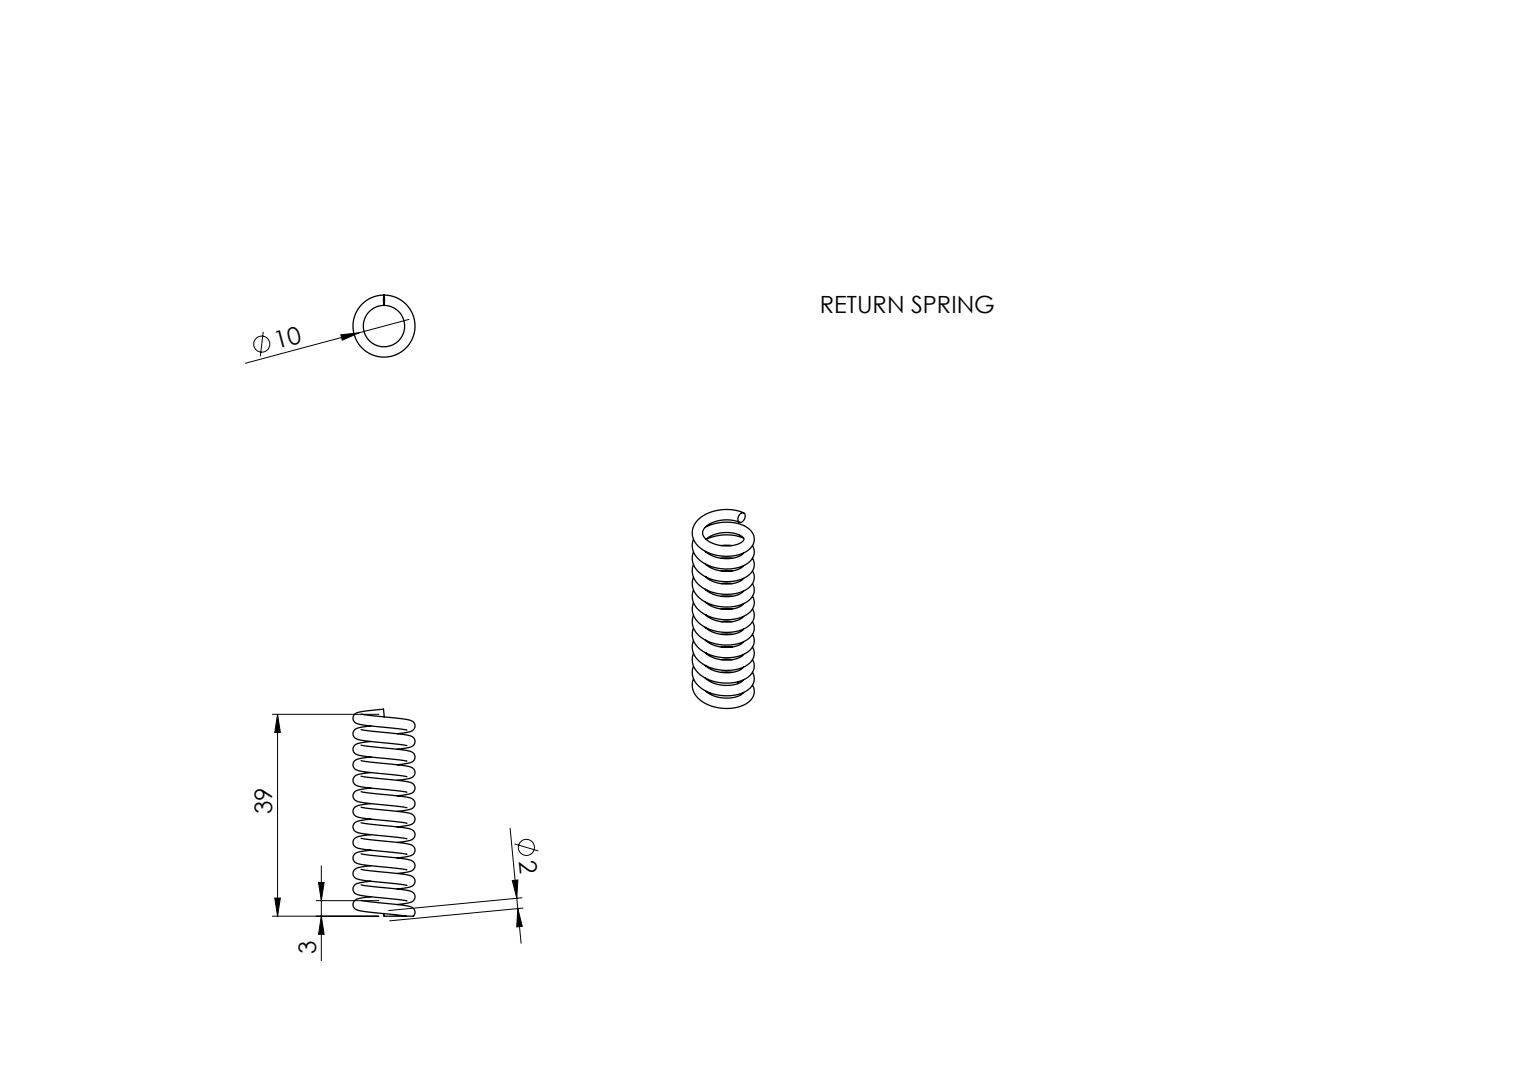
ISO-10303-21;
HEADER;
FILE_DESCRIPTION (('STEP AP214'),
    '1' );
FILE_NAME ('return spring.step',
    '2026-10-04T07:56:41',
    ( '' ),
    ( '' ),
    'SwSTEP 2.0',
    'SolidWorks 2026',
    '' );
FILE_SCHEMA (( 'AUTOMOTIVE_DESIGN' ));
ENDSEC;

DATA;
#1=CARTESIAN_POINT ( 'NONE',  ( 2.179377348189627916, -63.64547149457072805, 7.030887037049939003 ) ) ;
#3=CARTESIAN_POINT ( 'NONE',  ( 1.529537955723794918, -69.64547149457074227, 5.030887037049945221 ) ) ;
#4=CARTESIAN_POINT ( 'NONE',  ( -0.09506052544073731458, -60.49547149457074369, 4.999999999999997335 ) ) ;
#7=CARTESIAN_POINT ( 'NONE',  ( -3.015831842038216859, -60.30452850542926058, -3.989209796945429432 ) ) ;
#8=CARTESIAN_POINT ( 'NONE',  ( -7.360235569667856304, -89.74547149457073658, -0.09995255151716124498 ) ) ;
#10=CARTESIAN_POINT ( 'NONE',  ( -1.719659006605372076, -75.15452850542925489, -4.969112962950016588 ) ) ;
#15=CARTESIAN_POINT ( 'NONE',  ( -4.312004677470992142, -84.04547149457074795, 3.009306630940933758 ) ) ;
#16=CARTESIAN_POINT ( 'NONE',  ( 4.332187097882923332, -97.00000000000000000, -0.04074656551593417581 ) ) ;
#17=CARTESIAN_POINT ( 'NONE',  ( -2.610703060766926598, -69.04547149457074795, 1.773238653441125745 ) ) ;
#18=CARTESIAN_POINT ( 'NONE',  ( 6.628020296210641149, -74.40452850542925489, -2.253526892787612645 ) ) ;
#20=CARTESIAN_POINT ( 'NONE',  ( 4.725907263620373833, -82.09547149457074511, 1.635492904037598283 ) ) ;
#21=CARTESIAN_POINT ( 'NONE',  ( -5.257311121191324155, -60.75452850542925631, 0.09995255151729526277 ) ) ;
#22=CARTESIAN_POINT ( 'NONE',  ( -2.862020680886492308, -91.20452850542926626, 4.100960146804039752 ) ) ;
#23=CARTESIAN_POINT ( 'NONE',  ( -0.09506052544086251999, -66.00452850542926342, -6.999999999999997335 ) ) ;
#24=CARTESIAN_POINT ( 'NONE',  ( -2.823794231030039015, -86.59547149457075932, -1.017458915287723364 ) ) ;
#27=DIRECTION ( 'NONE',  ( -0.9954714945707483498, -0.09506052544079827971, 1.047588144072330487E-14 ) ) ;
#29=CARTESIAN_POINT ( 'NONE',  ( 4.194503406049339134, -89.55452850542926058, -3.171033256558100089 ) ) ;
#31=CARTESIAN_POINT ( 'NONE',  ( 1.529537955723690779, -80.85452850542925773, -5.030887037049978971 ) ) ;
#32=CARTESIAN_POINT ( 'NONE',  ( 2.493201789345269148, -59.55452850542924637, -1.934965279058294518 ) ) ;
#34=CARTESIAN_POINT ( 'NONE',  ( -1.719659006605370744, -90.15452850542922647, -4.969112962950016588 ) ) ;
#35=CARTESIAN_POINT ( 'NONE',  ( 4.037591185471445243, -92.70452850542926626, -5.718994135553947977 ) ) ;
#36=CARTESIAN_POINT ( 'NONE',  ( -3.015831842038128485, -81.19547149457073942, 3.989209796945492048 ) ) ;
#37=CARTESIAN_POINT ( 'NONE',  ( 2.823794231030039903, -71.40452850542924068, -1.017458915287783316 ) ) ;
#40=CARTESIAN_POINT ( 'NONE',  ( 2.823794231030042123, -89.40452850542926910, -1.017458915287783316 ) ) ;
#41=CARTESIAN_POINT ( 'NONE',  ( 2.179377348189484476, -95.85452850542924352, -7.030887037049986077 ) ) ;
#45=CARTESIAN_POINT ( 'NONE',  ( 1.719659006605391394, -79.65452850542925489, 4.969112962950016588 ) ) ;
#46=CARTESIAN_POINT ( 'NONE',  ( 2.369498399071079842, -94.84547149457073090, -6.969112962950057444 ) ) ;
#53=CARTESIAN_POINT ( 'NONE',  ( -1.529537955723671905, -61.35452850542925773, 5.030887037049979860 ) ) ;
#54=CARTESIAN_POINT ( 'NONE',  ( -4.191402346623057440, -87.19547149457073942, 5.607243785695398941 ) ) ;
#57=CARTESIAN_POINT ( 'NONE',  ( 5.257311121191341918, -71.25452850542923500, -0.09995255151729465215 ) ) ;
#61=CARTESIAN_POINT ( 'NONE',  ( 1.719659006605285922, -76.84547149457073090, -4.969112962950050338 ) ) ;
#62=CARTESIAN_POINT ( 'NONE',  ( 4.269446988268172483, -97.00000000000001421, -0.4101805542161022777 ) ) ;
#63=CARTESIAN_POINT ( 'NONE',  ( 0.8796985632579598091, -60.64547149457074227, 3.030887037049952326 ) ) ;
#64=CARTESIAN_POINT ( 'NONE',  ( 5.895805022753404678, -68.55452850542926058, -4.407101234057908989 ) ) ;
#66=CARTESIAN_POINT ( 'NONE',  ( -4.194503406049384431, -77.44547149457075363, -3.171033256558012159 ) ) ;
#67=CARTESIAN_POINT ( 'NONE',  ( 5.257311121191341918, -59.25452850542924210, -0.09995255151729465215 ) ) ;
#68=CARTESIAN_POINT ( 'NONE',  ( -4.725907263620319654, -87.90452850542926910, 1.635492904037698647 ) ) ;
#69=CARTESIAN_POINT ( 'NONE',  ( -4.191402346623179120, -72.30452850542926058, -5.607243785695311900 ) ) ;
#71=CARTESIAN_POINT ( 'NONE',  ( -2.823794231030039903, -77.59547149457073090, -1.017458915287723364 ) ) ;
#75=CARTESIAN_POINT ( 'NONE',  ( 2.862020680886515400, -86.70452850542925205, -4.100960146804039752 ) ) ;
#77=CARTESIAN_POINT ( 'NONE',  ( -1.529537955723670128, -79.35452850542925773, 5.030887037049979860 ) ) ;
#78=CARTESIAN_POINT ( 'NONE',  ( -2.610703060766966566, -63.45452850542924494, -1.773238653441072232 ) ) ;
#80=CARTESIAN_POINT ( 'NONE',  ( -2.862020680886493640, -82.20452850542925205, 4.100960146804039752 ) ) ;
#81=CARTESIAN_POINT ( 'NONE',  ( 2.369498399071075845, -64.84547149457071669, -6.969112962950057444 ) ) ;
#82=CARTESIAN_POINT ( 'NONE',  ( 1.069819614139556396, -70.65452850542925489, 2.969112962950023249 ) ) ;
#83=EDGE_CURVE ( 'NONE', #4707, #1590, #2672, .T. ) ;
#86=CARTESIAN_POINT ( 'NONE',  ( 3.154386672714810658, -89.25452850542926342, -0.09995255151727241993 ) ) ;
#87=CARTESIAN_POINT ( 'NONE',  ( 4.191402346623199549, -94.80452850542926058, 5.607243785695311900 ) ) ;
#89=CARTESIAN_POINT ( 'NONE',  ( 1.529537955723689890, -74.85452850542925773, -5.030887037049978971 ) ) ;
#90=CARTESIAN_POINT ( 'NONE',  ( -5.895805022753476621, -89.44547149457073942, -4.407101234057782868 ) ) ;
#93=CARTESIAN_POINT ( 'NONE',  ( -0.09506052544075821453, -63.49547149457075079, 2.999999999999997780 ) ) ;
#95=CARTESIAN_POINT ( 'NONE',  ( -4.312004677471060532, -60.45452850542923784, -3.009306630940844052 ) ) ;
#96=CARTESIAN_POINT ( 'NONE',  ( -6.013306294175058575, -87.04547149457074795, 4.245374608440741326 ) ) ;
#99=CARTESIAN_POINT ( 'NONE',  ( -3.015831842038215083, -75.30452850542926058, -3.989209796945429432 ) ) ;
#103=CARTESIAN_POINT ( 'NONE',  ( 2.862020680886599333, -78.79547149457074795, 4.100960146803977580 ) ) ;
#105=CARTESIAN_POINT ( 'NONE',  ( -1.840261337453202639, -60.19547149457074653, 2.371175808195584267 ) ) ;
#106=CARTESIAN_POINT ( 'NONE',  ( 6.686770931921523164, -65.10452850542924352, 2.072711028461649008 ) ) ;
#108=CARTESIAN_POINT ( 'NONE',  ( 1.529537955723795584, -81.64547149457074227, 5.030887037049945221 ) ) ;
#110=CARTESIAN_POINT ( 'NONE',  ( 3.015831842038235511, -88.80452850542926058, 3.989209796945429432 ) ) ;
#111=CARTESIAN_POINT ( 'NONE',  ( -6.013306294175152722, -72.45452850542925205, -4.245374608440613429 ) ) ;
#112=CARTESIAN_POINT ( 'NONE',  ( 3.154386672714809770, -79.24547149457073658, 0.09995255151720662534 ) ) ;
#118=CARTESIAN_POINT ( 'NONE',  ( -2.862020680886492308, -91.20452850542926626, 4.100960146804039752 ) ) ;
#120=CARTESIAN_POINT ( 'NONE',  ( 4.725907263620340970, -80.40452850542925489, -1.635492904037697981 ) ) ;
#121=CARTESIAN_POINT ( 'NONE',  ( 2.610703060766946582, -88.54547149457074795, -1.773238653441125523 ) ) ;
#123=CARTESIAN_POINT ( 'NONE',  ( -0.09506052544083921918, -84.00452850542926342, -4.999999999999997335 ) ) ;
#125=CARTESIAN_POINT ( 'NONE',  ( 0.09506052544073236021, -61.99547149457073658, -6.999999999999997335 ) ) ;
#127=CARTESIAN_POINT ( 'NONE',  ( -1.840261337453252821, -69.30452850542926058, -2.371175808195547852 ) ) ;
#131=CARTESIAN_POINT ( 'NONE',  ( 1.069819614139557284, -79.65452850542925489, 2.969112962950023249 ) ) ;
#132=CARTESIAN_POINT ( 'NONE',  ( 7.360235569667880284, -92.25452850542926342, -0.09995255151731691212 ) ) ;
#134=CARTESIAN_POINT ( 'NONE',  ( -6.628020296210666018, -86.59547149457075932, -2.253526892787471869 ) ) ;
#138=CARTESIAN_POINT ( 'NONE',  ( -0.8796985632579439329, -68.14547149457074227, -3.030887037049952326 ) ) ;
#139=CARTESIAN_POINT ( 'NONE',  ( -4.194503406049321370, -58.05452850542925347, 3.171033256558100533 ) ) ;
#141=CARTESIAN_POINT ( 'NONE',  ( 4.312004677471075631, -73.95452850542926626, 3.009306630940844496 ) ) ;
#142=CARTESIAN_POINT ( 'NONE',  ( -0.09506052544071266763, -87.49547149457075079, 6.999999999999997335 ) ) ;
#144=CARTESIAN_POINT ( 'NONE',  ( 0.09506052544086046607, -79.50452850542926342, 4.999999999999997335 ) ) ;
#147=CARTESIAN_POINT ( 'NONE',  ( -4.312004677470993030, -78.04547149457076216, 3.009306630940933758 ) ) ;
#149=CARTESIAN_POINT ( 'NONE',  ( -2.610703060766927930, -63.04547149457074084, 1.773238653441125745 ) ) ;
#150=CARTESIAN_POINT ( 'NONE',  ( -5.895805022753386915, -67.05452850542926058, 4.407101234057909878 ) ) ;
#152=CARTESIAN_POINT ( 'NONE',  ( -5.257311121191324155, -74.74547149457075079, -0.09995255151718371311 ) ) ;
#155=CARTESIAN_POINT ( 'NONE',  ( 0.09506052544086084077, -82.50452850542926342, 4.999999999999997335 ) ) ;
#156=CARTESIAN_POINT ( 'NONE',  ( 6.686770931921523164, -68.10452850542924352, 2.072711028461649008 ) ) ;
#157=CARTESIAN_POINT ( 'NONE',  ( 0.8796985632579618075, -75.64547149457072805, 3.030887037049952326 ) ) ;
#161=CARTESIAN_POINT ( 'NONE',  ( 2.862020680886516732, -95.70452850542926626, -4.100960146804039752 ) ) ;
#162=CARTESIAN_POINT ( 'NONE',  ( 3.015831842038235511, -88.80452850542926058, 3.989209796945429432 ) ) ;
#164=CARTESIAN_POINT ( 'NONE',  ( -2.862020680886494084, -79.20452850542925205, 4.100960146804039752 ) ) ;
#165=CARTESIAN_POINT ( 'NONE',  ( -3.154386672714787565, -89.74547149457073658, -0.09995255151720625064 ) ) ;
#166=CARTESIAN_POINT ( 'NONE',  ( 1.719659006605392504, -88.65452850542925489, 4.969112962950016588 ) ) ;
#168=CARTESIAN_POINT ( 'NONE',  ( -6.013306294175062128, -60.04547149457073374, 4.245374608440741326 ) ) ;
#169=CARTESIAN_POINT ( 'NONE',  ( -1.686450176301567350, -64.20452850542925205, 2.482926158054133303 ) ) ;
#172=CARTESIAN_POINT ( 'NONE',  ( 0.8796985632578988579, -74.85452850542925773, -3.030887037049972310 ) ) ;
#173=CARTESIAN_POINT ( 'NONE',  ( -2.179377348189460051, -88.35452850542924352, 7.030887037049988741 ) ) ;
#175=CARTESIAN_POINT ( 'NONE',  ( -4.037591185471542943, -89.29547149457074795, -5.718994135553860936 ) ) ;
#178=CARTESIAN_POINT ( 'NONE',  ( -1.069819614139475794, -66.34547149457073090, 2.969112962950044121 ) ) ;
#179=CARTESIAN_POINT ( 'NONE',  ( -4.725907263620323207, -63.90452850542925489, 1.635492904037698647 ) ) ;
#182=CARTESIAN_POINT ( 'NONE',  ( 5.257311121191341918, -71.25452850542923500, -0.09995255151729465215 ) ) ;
#183=CARTESIAN_POINT ( 'NONE',  ( 0.09506052544073499699, -82.99547149457075079, -6.999999999999997335 ) ) ;
#185=CARTESIAN_POINT ( 'NONE',  ( 1.529537955723690112, -77.85452850542922931, -5.030887037049978971 ) ) ;
#191=CARTESIAN_POINT ( 'NONE',  ( 3.015831842038148025, -70.69547149457073942, -3.989209796945492048 ) ) ;
#193=CARTESIAN_POINT ( 'NONE',  ( -1.686450176301618642, -65.29547149457073374, -2.482926158054096000 ) ) ;
#194=CARTESIAN_POINT ( 'NONE',  ( 7.360235569667877620, -74.25452850542924921, -0.09995255151731691212 ) ) ;
#197=CARTESIAN_POINT ( 'NONE',  ( 1.529537955723691001, -83.85452850542927195, -5.030887037049978971 ) ) ;
#198=CARTESIAN_POINT ( 'NONE',  ( -6.628020296210623385, -63.90452850542925489, 2.253526892787613978 ) ) ;
#199=CARTESIAN_POINT ( 'NONE',  ( -1.069819614139474906, -75.34547149457073090, 2.969112962950044121 ) ) ;
#202=CARTESIAN_POINT ( 'NONE',  ( -1.719659006605370744, -93.15452850542925489, -4.969112962950016588 ) ) ;
#203=CARTESIAN_POINT ( 'NONE',  ( 4.725907263620340970, -83.40452850542925489, -1.635492904037697981 ) ) ;
#205=CARTESIAN_POINT ( 'NONE',  ( 5.257311121191341030, -71.25452850542924921, -0.09995255151729466603 ) ) ;
#206=CARTESIAN_POINT ( 'NONE',  ( 2.610703060766947914, -94.54547149457073374, -1.773238653441125523 ) ) ;
#207=CARTESIAN_POINT ( 'NONE',  ( -4.194503406049315153, -91.05452850542923215, 3.171033256558100533 ) ) ;
#208=CARTESIAN_POINT ( 'NONE',  ( 6.013306294175077227, -61.54547149457074084, -4.245374608440741326 ) ) ;
#209=CARTESIAN_POINT ( 'NONE',  ( -1.840261337453252821, -66.30452850542926058, -2.371175808195547852 ) ) ;
#213=CARTESIAN_POINT ( 'NONE',  ( -1.686450176301564907, -82.20452850542925205, 2.482926158054133303 ) ) ;
#214=CARTESIAN_POINT ( 'NONE',  ( 2.179377348189483143, -86.85452850542924352, -7.030887037049986077 ) ) ;
#215=CARTESIAN_POINT ( 'NONE',  ( -4.191402346623057440, -87.19547149457073942, 5.607243785695398941 ) ) ;
#218=CARTESIAN_POINT ( 'NONE',  ( -0.09506052544075743738, -69.49547149457075079, 2.999999999999997780 ) ) ;
#223=CARTESIAN_POINT ( 'NONE',  ( -4.194503406049319594, -67.05452850542926058, 3.171033256558100533 ) ) ;
#224=CARTESIAN_POINT ( 'NONE',  ( 6.628020296210687334, -79.09547149457075932, 2.253526892787472757 ) ) ;
#228=CARTESIAN_POINT ( 'NONE',  ( -5.257311121191324155, -63.75452850542925631, 0.09995255151729526277 ) ) ;
#230=CARTESIAN_POINT ( 'NONE',  ( -5.257311121191324155, -71.74547149457075079, -0.09995255151718371311 ) ) ;
#232=CARTESIAN_POINT ( 'NONE',  ( 1.719659006605287921, -97.84547149457071669, -4.969112962950050338 ) ) ;
#233=CARTESIAN_POINT ( 'NONE',  ( 6.686770931921522276, -62.10452850542925063, 2.072711028461649008 ) ) ;
#235=CARTESIAN_POINT ( 'NONE',  ( 1.719659006605391616, -82.65452850542925489, 4.969112962950016588 ) ) ;
#236=CARTESIAN_POINT ( 'NONE',  ( 6.628020296210639373, -62.40452850542925489, -2.253526892787612645 ) ) ;
#237=CARTESIAN_POINT ( 'NONE',  ( 2.882544866740877065, -73.39547149457074227, -0.8366430509619593447 ) ) ;
#240=CARTESIAN_POINT ( 'NONE',  ( 3.015831842038236399, -94.80452850542924637, 3.989209796945429432 ) ) ;
#241=CARTESIAN_POINT ( 'NONE',  ( 1.529537955723690112, -77.85452850542922931, -5.030887037049978971 ) ) ;
#243=CARTESIAN_POINT ( 'NONE',  ( -4.312004677471057867, -72.45452850542923784, -3.009306630940843608 ) ) ;
#244=CARTESIAN_POINT ( 'NONE',  ( -0.8796985632579418235, -86.14547149457072805, -3.030887037049952326 ) ) ;
#245=CARTESIAN_POINT ( 'NONE',  ( 2.862020680886601998, -96.79547149457073374, 4.100960146803977580 ) ) ;
#246=CARTESIAN_POINT ( 'NONE',  ( 0.09506052544086046607, -79.50452850542926342, 4.999999999999997335 ) ) ;
#247=CARTESIAN_POINT ( 'NONE',  ( 2.369498399071225947, -85.65452850542926910, 6.969112962950009482 ) ) ;
#249=CARTESIAN_POINT ( 'NONE',  ( 1.686450176301584225, -68.70452850542925205, -2.482926158054133303 ) ) ;
#252=LINE ( 'NONE', #8058, #5108 ) ;
#253=CARTESIAN_POINT ( 'NONE',  ( 1.686450176301585335, -77.70452850542925205, -2.482926158054133303 ) ) ;
#254=CARTESIAN_POINT ( 'NONE',  ( 7.360235569667880284, -86.25452850542924921, -0.09995255151731691212 ) ) ;
#256=CARTESIAN_POINT ( 'NONE',  ( 4.191402346623080533, -88.69547149457073942, -5.607243785695398941 ) ) ;
#260=CARTESIAN_POINT ( 'NONE',  ( 0.09506052544077478461, -64.99547149457075079, -2.999999999999997780 ) ) ;
#263=CARTESIAN_POINT ( 'NONE',  ( 3.015831842038232402, -64.80452850542926058, 3.989209796945429432 ) ) ;
#264=CARTESIAN_POINT ( 'NONE',  ( 2.369498399071077177, -76.84547149457073090, -6.969112962950057444 ) ) ;
#265=FILL_AREA_STYLE ('',( #2132 ) ) ;
#268=CARTESIAN_POINT ( 'NONE',  ( -1.719659006605265716, -75.34547149457074511, 4.969112962950051227 ) ) ;
#269=CARTESIAN_POINT ( 'NONE',  ( -0.09506052544084110656, -69.00452850542926342, -4.999999999999997335 ) ) ;
#272=CARTESIAN_POINT ( 'NONE',  ( -4.784657899331159925, -65.89547149457074227, 1.454677039711874675 ) ) ;
#274=CARTESIAN_POINT ( 'NONE',  ( -4.784657899331155484, -95.89547149457074227, 1.454677039711874675 ) ) ;
#275=CARTESIAN_POINT ( 'NONE',  ( -6.013306294175153610, -60.45452850542925916, -4.245374608440613429 ) ) ;
#279=CARTESIAN_POINT ( 'NONE',  ( 1.529537955723690557, -80.85452850542925773, -5.030887037049978971 ) ) ;
#283=CARTESIAN_POINT ( 'NONE',  ( -4.312004677471056091, -87.45452850542925205, -3.009306630940844052 ) ) ;
#284=CARTESIAN_POINT ( 'NONE',  ( -1.529537955723669684, -82.35452850542922931, 5.030887037049979860 ) ) ;
#286=CARTESIAN_POINT ( 'NONE',  ( -0.09506052544084110656, -69.00452850542926342, -4.999999999999997335 ) ) ;
#287=CARTESIAN_POINT ( 'NONE',  ( 2.493201789345311337, -87.94547149457073942, 1.934965279058241006 ) ) ;
#288=CARTESIAN_POINT ( 'NONE',  ( -2.493201789345293129, -59.44547149457074653, -1.934965279058240561 ) ) ;
#289=CARTESIAN_POINT ( 'NONE',  ( 1.719659006605391172, -76.65452850542922647, 4.969112962950016588 ) ) ;
#290=CARTESIAN_POINT ( 'NONE',  ( 6.628020296210642037, -86.40452850542926910, -2.253526892787612645 ) ) ;
#292=CARTESIAN_POINT ( 'NONE',  ( -2.493201789345288688, -95.44547149457075363, -1.934965279058240561 ) ) ;
#296=CARTESIAN_POINT ( 'NONE',  ( 1.840261337453271473, -82.80452850542926058, 2.371175808195547852 ) ) ;
#297=CARTESIAN_POINT ( 'NONE',  ( -7.360235569667856304, -87.75452850542924921, 0.09995255151731782806 ) ) ;
#298=CARTESIAN_POINT ( 'NONE',  ( 2.369498399071078065, -79.84547149457074511, -6.969112962950057444 ) ) ;
#300=CARTESIAN_POINT ( 'NONE',  ( 2.862020680886601554, -93.79547149457074795, 4.100960146803977580 ) ) ;
#301=CARTESIAN_POINT ( 'NONE',  ( -0.8796985632578785408, -82.35452850542927195, 3.030887037049973198 ) ) ;
#306=CARTESIAN_POINT ( 'NONE',  ( -5.257311121191324155, -63.75452850542925631, 0.09995255151729526277 ) ) ;
#307=CARTESIAN_POINT ( 'NONE',  ( -2.369498399071056305, -84.34547149457075932, 6.969112962950058332 ) ) ;
#309=CARTESIAN_POINT ( 'NONE',  ( 1.529537955723795584, -75.64547149457072805, 5.030887037049945221 ) ) ;
#310=CARTESIAN_POINT ( 'NONE',  ( 4.784657899331176800, -73.39547149457074227, -1.454677039711874009 ) ) ;
#311=CARTESIAN_POINT ( 'NONE',  ( -4.194503406049319594, -67.05452850542926058, 3.171033256558100533 ) ) ;
#313=CARTESIAN_POINT ( 'NONE',  ( 1.529537955723795140, -69.64547149457074227, 5.030887037049945221 ) ) ;
#315=CARTESIAN_POINT ( 'NONE',  ( -6.686770931921508954, -57.60452850542926484, -2.072711028461647675 ) ) ;
#322=CARTESIAN_POINT ( 'NONE',  ( -4.194503406049315153, -88.05452850542921794, 3.171033256558100533 ) ) ;
#323=CARTESIAN_POINT ( 'NONE',  ( -4.312004677471057867, -78.45452850542925205, -3.009306630940844052 ) ) ;
#325=CARTESIAN_POINT ( 'NONE',  ( 1.719659006605389839, -67.65452850542925489, 4.969112962950015699 ) ) ;
#326=CARTESIAN_POINT ( 'NONE',  ( 0.09506052544077665811, -79.99547149457075079, -2.999999999999997780 ) ) ;
#327=CARTESIAN_POINT ( 'NONE',  ( -4.312004677470990366, -96.04547149457074795, 3.009306630940933758 ) ) ;
#329=CARTESIAN_POINT ( 'NONE',  ( -4.194503406049316929, -73.05452850542926058, 3.171033256558100533 ) ) ;
#330=CARTESIAN_POINT ( 'NONE',  ( -6.013306294175149169, -87.45452850542925205, -4.245374608440613429 ) ) ;
#331=CARTESIAN_POINT ( 'NONE',  ( 2.823794231030038571, -59.40452850542925489, -1.017458915287783316 ) ) ;
#336=CARTESIAN_POINT ( 'NONE',  ( 2.823794231030039903, -71.40452850542924068, -1.017458915287783316 ) ) ;
#337=CARTESIAN_POINT ( 'NONE',  ( -6.013306294175152722, -78.45452850542925205, -4.245374608440613429 ) ) ;
#338=CARTESIAN_POINT ( 'NONE',  ( -6.628020296210667794, -80.59547149457075932, -2.253526892787471869 ) ) ;
#340=CARTESIAN_POINT ( 'NONE',  ( -4.784657899331155484, -95.89547149457074227, 1.454677039711874675 ) ) ;
#341=CARTESIAN_POINT ( 'NONE',  ( 0.8796985632579006342, -89.85452850542924352, -3.030887037049972310 ) ) ;
#345=CARTESIAN_POINT ( 'NONE',  ( -2.882544866740875289, -93.60452850542925773, -0.8366430509618996147 ) ) ;
#346=CARTESIAN_POINT ( 'NONE',  ( 5.895805022753496161, -84.94547149457073942, 4.407101234057782868 ) ) ;
#349=CARTESIAN_POINT ( 'NONE',  ( 4.194503406049401306, -72.94547149457073942, 3.171033256558012159 ) ) ;
#350=CARTESIAN_POINT ( 'NONE',  ( -5.257311121191324155, -71.74547149457075079, -0.09995255151718371311 ) ) ;
#351=CARTESIAN_POINT ( 'NONE',  ( -4.312004677471058756, -69.45452850542925205, -3.009306630940844052 ) ) ;
#354=CARTESIAN_POINT ( 'NONE',  ( -4.725907263620354293, -68.59547149457073090, -1.635492904037597617 ) ) ;
#355=CARTESIAN_POINT ( 'NONE',  ( 2.369498399071222838, -58.65452850542925489, 6.969112962950009482 ) ) ;
#362=CARTESIAN_POINT ( 'NONE',  ( 5.257311121191341918, -83.25452850542926342, -0.09995255151729465215 ) ) ;
#363=CARTESIAN_POINT ( 'NONE',  ( 4.725907263620340082, -74.40452850542925489, -1.635492904037697981 ) ) ;
#364=CARTESIAN_POINT ( 'NONE',  ( -4.194503406049317817, -76.05452850542926058, 3.171033256558101865 ) ) ;
#365=CARTESIAN_POINT ( 'NONE',  ( 2.610703060766946138, -79.54547149457074795, -1.773238653441125523 ) ) ;
#366=CARTESIAN_POINT ( 'NONE',  ( 5.257311121191343695, -97.24547149457075079, 0.09995255151718437925 ) ) ;
#367=CARTESIAN_POINT ( 'NONE',  ( -4.312004677471058756, -69.45452850542925205, -3.009306630940844052 ) ) ;
#368=CARTESIAN_POINT ( 'NONE',  ( -4.191402346623178232, -84.30452850542926058, -5.607243785695311900 ) ) ;
#370=CARTESIAN_POINT ( 'NONE',  ( 0.09506052544083654077, -58.50452850542925631, 2.999999999999997780 ) ) ;
#377=CARTESIAN_POINT ( 'NONE',  ( -0.09506052544081970701, -72.00452850542926342, -2.999999999999997780 ) ) ;
#378=CARTESIAN_POINT ( 'NONE',  ( 6.013306294175077227, -79.54547149457074795, -4.245374608440741326 ) ) ;
#381=CARTESIAN_POINT ( 'NONE',  ( -2.610703060766964345, -81.45452850542925205, -1.773238653441072232 ) ) ;
#385=CARTESIAN_POINT ( 'NONE',  ( 0.09506052544084107880, -94.50452850542926342, 2.999999999999997780 ) ) ;
#387=CARTESIAN_POINT ( 'NONE',  ( -7.360235569667858968, -68.74547149457075079, -0.09995255151716124498 ) ) ;
#390=CARTESIAN_POINT ( 'NONE',  ( 4.194503406049403083, -75.94547149457073942, 3.171033256558012159 ) ) ;
#391=CARTESIAN_POINT ( 'NONE',  ( -0.09506052544073655131, -66.49547149457075079, 4.999999999999997335 ) ) ;
#392=CARTESIAN_POINT ( 'NONE',  ( 4.194503406049335581, -65.55452850542923215, -3.171033256558100089 ) ) ;
#398=CARTESIAN_POINT ( 'NONE',  ( 3.015831842038147137, -64.69547149457075363, -3.989209796945492048 ) ) ;
#400=CARTESIAN_POINT ( 'NONE',  ( 4.312004677471079184, -94.95452850542926626, 3.009306630940844496 ) ) ;
#405=CARTESIAN_POINT ( 'NONE',  ( -2.862020680886492752, -88.20452850542925205, 4.100960146804039752 ) ) ;
#406=CARTESIAN_POINT ( 'NONE',  ( -4.784657899331190123, -78.60452850542925773, -1.454677039711773867 ) ) ;
#408=CARTESIAN_POINT ( 'NONE',  ( -4.725907263620323207, -63.90452850542925489, 1.635492904037698647 ) ) ;
#409=CARTESIAN_POINT ( 'NONE',  ( -2.823794231030039459, -83.59547149457075932, -1.017458915287723364 ) ) ;
#410=CARTESIAN_POINT ( 'NONE',  ( -0.09506052544075858923, -60.49547149457073658, 2.999999999999997780 ) ) ;
#411=CARTESIAN_POINT ( 'NONE',  ( 5.257311121191341918, -68.25452850542926342, -0.09995255151729465215 ) ) ;
#412=CARTESIAN_POINT ( 'NONE',  ( 4.037591185471443467, -83.70452850542925205, -5.718994135553947977 ) ) ;
#413=CARTESIAN_POINT ( 'NONE',  ( 2.610703060766947914, -97.54547149457074795, -1.773238653441125523 ) ) ;
#418=CARTESIAN_POINT ( 'NONE',  ( -1.529537955723668574, -91.35452850542924352, 5.030887037049979860 ) ) ;
#419=CARTESIAN_POINT ( 'NONE',  ( -0.09506052544082045641, -66.00452850542926342, -2.999999999999997780 ) ) ;
#420=CARTESIAN_POINT ( 'NONE',  ( -5.895805022753477509, -80.44547149457073942, -4.407101234057782868 ) ) ;
#422=CARTESIAN_POINT ( 'NONE',  ( 0.09506052544075753452, -94.99547149457073658, -4.999999999999997335 ) ) ;
#423=CARTESIAN_POINT ( 'NONE',  ( -2.882544866740876177, -84.60452850542927195, -0.8366430509618996147 ) ) ;
#427=CARTESIAN_POINT ( 'NONE',  ( -5.257311121191324155, -60.75452850542925631, 0.09995255151729526277 ) ) ;
#428=CARTESIAN_POINT ( 'NONE',  ( -2.179377348189611929, -71.14547149457074227, -7.030887037049939003 ) ) ;
#430=CARTESIAN_POINT ( 'NONE',  ( 4.460500007776900588, -96.99999999999960210, 2.535776773627464564 ) ) ;
#431=CARTESIAN_POINT ( 'NONE',  ( 3.015831842038148025, -70.69547149457073942, -3.989209796945492048 ) ) ;
#432=CARTESIAN_POINT ( 'NONE',  ( -4.312004677470993919, -72.04547149457074795, 3.009306630940933758 ) ) ;
#433=CARTESIAN_POINT ( 'NONE',  ( -1.719659006605374962, -57.15452850542924068, -4.969112962950016588 ) ) ;
#436=CARTESIAN_POINT ( 'NONE',  ( 0.09506052544085857869, -64.50452850542926342, 4.999999999999997335 ) ) ;
#437=CARTESIAN_POINT ( 'NONE',  ( 4.312004677471010794, -64.54547149457073374, -3.009306630940933314 ) ) ;
#439=CARTESIAN_POINT ( 'NONE',  ( -4.194503406049314265, -94.05452850542926058, 3.171033256558100533 ) ) ;
#441=DIRECTION ( 'NONE',  ( -0.09506052544079829358, 0.9954714945707483498, 0.000000000000000000 ) ) ;
#444=CARTESIAN_POINT ( 'NONE',  ( -1.529537955723669684, -82.35452850542922931, 5.030887037049979860 ) ) ;
#445=CARTESIAN_POINT ( 'NONE',  ( 4.725907263620374721, -94.09547149457074511, 1.635492904037598283 ) ) ;
#446=CARTESIAN_POINT ( 'NONE',  ( 3.015831842038231958, -61.80452850542926058, 3.989209796945429432 ) ) ;
#447=CARTESIAN_POINT ( 'NONE',  ( -1.686450176301616199, -83.29547149457074795, -2.482926158054096000 ) ) ;
#448=CARTESIAN_POINT ( 'NONE',  ( 4.784657899331178577, -85.39547149457074227, -1.454677039711874009 ) ) ;
#449=CARTESIAN_POINT ( 'NONE',  ( 4.194503406049335581, -71.55452850542926058, -3.171033256558100089 ) ) ;
#450=CARTESIAN_POINT ( 'NONE',  ( 2.179377348189481811, -74.85452850542925773, -7.030887037049986077 ) ) ;
#454=CARTESIAN_POINT ( 'NONE',  ( -0.09506052544082121969, -60.00452850542925631, -2.999999999999997780 ) ) ;
#459=CARTESIAN_POINT ( 'NONE',  ( 0.09506052544086197875, -91.50452850542924921, 4.999999999999997335 ) ) ;
#460=CARTESIAN_POINT ( 'NONE',  ( -2.493201789345253161, -70.05452850542926058, 1.934965279058294518 ) ) ;
#461=CARTESIAN_POINT ( 'NONE',  ( 5.895805022753402902, -59.55452850542924637, -4.407101234057908989 ) ) ;
#462=CARTESIAN_POINT ( 'NONE',  ( -5.895805022753476621, -83.44547149457073942, -4.407101234057782868 ) ) ;
#464=CARTESIAN_POINT ( 'NONE',  ( -4.312004677470992142, -87.04547149457074795, 3.009306630940933314 ) ) ;
#465=CARTESIAN_POINT ( 'NONE',  ( -1.069819614139537078, -87.15452850542926910, -2.969112962950023249 ) ) ;
#469=CARTESIAN_POINT ( 'NONE',  ( -0.09506052544081666777, -96.00452850542926342, -2.999999999999997780 ) ) ;
#470=CARTESIAN_POINT ( 'NONE',  ( -7.360235569667858968, -71.74547149457075079, -0.09995255151716124498 ) ) ;
#472=CARTESIAN_POINT ( 'NONE',  ( 5.713289348668859624, -96.99999999999995737, -0.5550645300988114039 ) ) ;
#473=CARTESIAN_POINT ( 'NONE',  ( 4.725907263620372056, -67.09547149457073090, 1.635492904037598283 ) ) ;
#474=CARTESIAN_POINT ( 'NONE',  ( -4.725907263620354293, -71.59547149457074511, -1.635492904037597617 ) ) ;
#475=CARTESIAN_POINT ( 'NONE',  ( -5.257311121191324155, -60.75452850542925631, 0.09995255151729526277 ) ) ;
#478=CARTESIAN_POINT ( 'NONE',  ( -1.529537955723671239, -70.35452850542925773, 5.030887037049979860 ) ) ;
#479=CARTESIAN_POINT ( 'NONE',  ( 4.784657899331175912, -64.39547149457074227, -1.454677039711874009 ) ) ;
#484=CARTESIAN_POINT ( 'NONE',  ( 4.194503406049337357, -77.55452850542926058, -3.171033256558100089 ) ) ;
#485=CARTESIAN_POINT ( 'NONE',  ( -1.719659006605263940, -93.34547149457071669, 4.969112962950051227 ) ) ;
#486=CARTESIAN_POINT ( 'NONE',  ( 4.194503406049335581, -62.55452850542925347, -3.171033256558100977 ) ) ;
#487=CARTESIAN_POINT ( 'NONE',  ( -2.882544866740858414, -68.89547149457074227, 0.8366430509619596778 ) ) ;
#488=CARTESIAN_POINT ( 'NONE',  ( -4.191402346623179120, -75.30452850542926058, -5.607243785695311900 ) ) ;
#489=CARTESIAN_POINT ( 'NONE',  ( 4.725907263620373833, -85.09547149457074511, 1.635492904037598283 ) ) ;
#490=CARTESIAN_POINT ( 'NONE',  ( -4.725907263620322318, -69.90452850542925489, 1.635492904037698647 ) ) ;
#491=CARTESIAN_POINT ( 'NONE',  ( 2.369498399071225503, -79.65452850542925489, 6.969112962950009482 ) ) ;
#492=CARTESIAN_POINT ( 'NONE',  ( 0.8796985632579631398, -87.64547149457075648, 3.030887037049952326 ) ) ;
#496=ORIENTED_EDGE ( 'NONE', *, *, #8064, .T. ) ;
#497=CARTESIAN_POINT ( 'NONE',  ( -1.529537955723668796, -88.35452850542925773, 5.030887037049979860 ) ) ;
#498=CARTESIAN_POINT ( 'NONE',  ( 1.840261337453269919, -70.80452850542926058, 2.371175808195547852 ) ) ;
#500=CARTESIAN_POINT ( 'NONE',  ( 0.09506052544086197875, -91.50452850542924921, 4.999999999999997335 ) ) ;
#501=CARTESIAN_POINT ( 'NONE',  ( 5.895805022753492608, -69.94547149457073942, 4.407101234057782868 ) ) ;
#502=CARTESIAN_POINT ( 'NONE',  ( 4.784657899331178577, -82.39547149457074227, -1.454677039711874009 ) ) ;
#503=CARTESIAN_POINT ( 'NONE',  ( 1.069819614139557284, -79.65452850542925489, 2.969112962950023249 ) ) ;
#506=CARTESIAN_POINT ( 'NONE',  ( 1.719659006605388507, -61.65452850542923358, 4.969112962950016588 ) ) ;
#507=CARTESIAN_POINT ( 'NONE',  ( -6.013306294175060351, -75.04547149457074795, 4.245374608440741326 ) ) ;
#509=( NAMED_UNIT ( * ) PLANE_ANGLE_UNIT ( ) SI_UNIT ( $, .RADIAN. ) );
#511=CARTESIAN_POINT ( 'NONE',  ( 0.09506052544075412059, -67.99547149457075079, -4.999999999999997335 ) ) ;
#512=CARTESIAN_POINT ( 'NONE',  ( 6.628020296210689111, -94.09547149457074511, 2.253526892787472757 ) ) ;
#513=CARTESIAN_POINT ( 'NONE',  ( 2.823794231030042567, -95.40452850542926910, -1.017458915287783316 ) ) ;
#516=CARTESIAN_POINT ( 'NONE',  ( 5.257311121191341918, -65.25452850542926342, -0.09995255151729465215 ) ) ;
#517=CARTESIAN_POINT ( 'NONE',  ( 1.719659006605283924, -64.84547149457071669, -4.969112962950050338 ) ) ;
#526=CARTESIAN_POINT ( 'NONE',  ( -4.194503406049316041, -79.05452850542921794, 3.171033256558100533 ) ) ;
#528=CARTESIAN_POINT ( 'NONE',  ( 4.194503406049402194, -90.94547149457071100, 3.171033256558012159 ) ) ;
#529=CARTESIAN_POINT ( 'NONE',  ( 4.312004677471074743, -61.95452850542925205, 3.009306630940844052 ) ) ;
#530=CARTESIAN_POINT ( 'NONE',  ( -1.686450176301617976, -68.29547149457073374, -2.482926158054096000 ) ) ;
#531=CARTESIAN_POINT ( 'NONE',  ( 6.686770931921523164, -77.10452850542924352, 2.072711028461649008 ) ) ;
#532=CARTESIAN_POINT ( 'NONE',  ( -4.784657899331157260, -86.89547149457074227, 1.454677039711874675 ) ) ;
#533=CARTESIAN_POINT ( 'NONE',  ( 2.862020680886513180, -68.70452850542925205, -4.100960146804039752 ) ) ;
#535=CARTESIAN_POINT ( 'NONE',  ( -7.360235569667858968, -75.75452850542926342, 0.09995255151731782806 ) ) ;
#536=CARTESIAN_POINT ( 'NONE',  ( 2.493201789345310893, -84.94547149457073942, 1.934965279058241006 ) ) ;
#541=CARTESIAN_POINT ( 'NONE',  ( 0.09506052544086160405, -88.50452850542924921, 4.999999999999997335 ) ) ;
#542=CARTESIAN_POINT ( 'NONE',  ( 0.8796985632578971925, -62.85452850542923642, -3.030887037049972310 ) ) ;
#544=CARTESIAN_POINT ( 'NONE',  ( -2.862020680886492308, -94.20452850542926626, 4.100960146804039752 ) ) ;
#545=CARTESIAN_POINT ( 'NONE',  ( 7.360235569667877620, -67.24547149457075079, 0.09995255151716216091 ) ) ;
#546=CARTESIAN_POINT ( 'NONE',  ( -0.09506052544073390065, -87.49547149457075079, 4.999999999999997335 ) ) ;
#547=CARTESIAN_POINT ( 'NONE',  ( -2.610703060766965677, -72.45452850542925205, -1.773238653441072232 ) ) ;
#551=CARTESIAN_POINT ( 'NONE',  ( 1.686450176301586223, -83.70452850542925205, -2.482926158054133303 ) ) ;
#552=CARTESIAN_POINT ( 'NONE',  ( 7.360235569667877620, -67.24547149457075079, 0.09995255151716216091 ) ) ;
#553=CARTESIAN_POINT ( 'NONE',  ( 1.766089183626466941, -96.99999999999998579, -5.729544030250906417 ) ) ;
#554=CARTESIAN_POINT ( 'NONE',  ( 5.257311121191341030, -67.24547149457075079, 0.09995255151718437925 ) ) ;
#555=CARTESIAN_POINT ( 'NONE',  ( -5.895805022753475733, -95.44547149457075363, -4.407101234057782868 ) ) ;
#556=CARTESIAN_POINT ( 'NONE',  ( 2.493201789345274033, -95.55452850542926058, -1.934965279058294518 ) ) ;
#558=CARTESIAN_POINT ( 'NONE',  ( 0.09506052544085932809, -70.50452850542926342, 4.999999999999997335 ) ) ;
#559=CARTESIAN_POINT ( 'NONE',  ( 3.015831842038146693, -61.69547149457073942, -3.989209796945492048 ) ) ;
#567=CARTESIAN_POINT ( 'NONE',  ( -2.862020680886494528, -76.20452850542926626, 4.100960146804039752 ) ) ;
#568=CARTESIAN_POINT ( 'NONE',  ( -1.719659006605264384, -87.34547149457074511, 4.969112962950051227 ) ) ;
#569=CARTESIAN_POINT ( 'NONE',  ( 0.09506052544085857869, -64.50452850542926342, 4.999999999999997335 ) ) ;
#570=CARTESIAN_POINT ( 'NONE',  ( -1.069819614139475794, -69.34547149457073090, 2.969112962950044121 ) ) ;
#571=CARTESIAN_POINT ( 'NONE',  ( -2.179377348189460939, -82.35452850542927195, 7.030887037049988741 ) ) ;
#572=CARTESIAN_POINT ( 'NONE',  ( 5.257311121191342806, -88.24547149457073658, 0.09995255151718437925 ) ) ;
#574=CARTESIAN_POINT ( 'NONE',  ( 2.369498399071225059, -76.65452850542925489, 6.969112962950009482 ) ) ;
#575=CARTESIAN_POINT ( 'NONE',  ( -2.882544866740856637, -86.89547149457074227, 0.8366430509619596778 ) ) ;
#581=CARTESIAN_POINT ( 'NONE',  ( 4.312004677471078296, -88.95452850542925205, 3.009306630940844052 ) ) ;
#582=CARTESIAN_POINT ( 'NONE',  ( -1.840261337453253931, -60.30452850542926058, -2.371175808195547852 ) ) ;
#584=CARTESIAN_POINT ( 'NONE',  ( -7.360235569667860744, -57.75452850542924921, 0.09995255151731782806 ) ) ;
#586=CARTESIAN_POINT ( 'NONE',  ( -7.360235569667860744, -65.74547149457073658, -0.09995255151716124498 ) ) ;
#587=CARTESIAN_POINT ( 'NONE',  ( 4.725907263620374721, -91.09547149457074511, 1.635492904037598283 ) ) ;
#588=CARTESIAN_POINT ( 'NONE',  ( -1.840261337453252155, -72.30452850542926058, -2.371175808195547852 ) ) ;
#592=CARTESIAN_POINT ( 'NONE',  ( -1.840261337453250157, -87.30452850542926058, -2.371175808195547852 ) ) ;
#593=CARTESIAN_POINT ( 'NONE',  ( -0.09506052544071605381, -60.49547149457073658, 6.999999999999997335 ) ) ;
#595=CARTESIAN_POINT ( 'NONE',  ( 4.725907263620371168, -64.09547149457073090, 1.635492904037598283 ) ) ;
#596=CARTESIAN_POINT ( 'NONE',  ( 0.09506052544075337118, -61.99547149457074369, -4.999999999999997335 ) ) ;
#597=CARTESIAN_POINT ( 'NONE',  ( 0.8796985632579009673, -92.85452850542924352, -3.030887037049972310 ) ) ;
#599=CARTESIAN_POINT ( 'NONE',  ( 4.194503406049335581, -65.55452850542923215, -3.171033256558100089 ) ) ;
#600=CARTESIAN_POINT ( 'NONE',  ( -5.895805022753476621, -89.44547149457073942, -4.407101234057782868 ) ) ;
#606=CARTESIAN_POINT ( 'NONE',  ( 1.719659006605391394, -79.65452850542925489, 4.969112962950016588 ) ) ;
#607=CARTESIAN_POINT ( 'NONE',  ( 4.784657899331177688, -76.39547149457074227, -1.454677039711874009 ) ) ;
#608=CARTESIAN_POINT ( 'NONE',  ( 4.227364539074073946, -96.99999999999998579, -0.5958093000394333316 ) ) ;
#609=CARTESIAN_POINT ( 'NONE',  ( -2.882544866740858414, -71.89547149457074227, 0.8366430509619596778 ) ) ;
#610=CARTESIAN_POINT ( 'NONE',  ( -4.037591185471422150, -82.20452850542925205, 5.718994135553947977 ) ) ;
#612=CARTESIAN_POINT ( 'NONE',  ( 5.257311121191341918, -85.24547149457075079, 0.09995255151718437925 ) ) ;
#614=CARTESIAN_POINT ( 'NONE',  ( 4.725907263620342746, -95.40452850542925489, -1.635492904037697981 ) ) ;
#615=CARTESIAN_POINT ( 'NONE',  ( -2.369498399071206407, -81.15452850542924068, -6.969112962950009482 ) ) ;
#616=CARTESIAN_POINT ( 'NONE',  ( 0.8796985632579628067, -84.64547149457074227, 3.030887037049952326 ) ) ;
#621=CARTESIAN_POINT ( 'NONE',  ( 4.194503406049339134, -83.55452850542924637, -3.171033256558100977 ) ) ;
#622=CARTESIAN_POINT ( 'NONE',  ( -2.882544866740879730, -57.60452850542926484, -0.8366430509618996147 ) ) ;
#623=CARTESIAN_POINT ( 'NONE',  ( -4.037591185471424815, -61.20452850542925916, 5.718994135553947977 ) ) ;
#624=CARTESIAN_POINT ( 'NONE',  ( -2.179377348189611929, -71.14547149457074227, -7.030887037049939003 ) ) ;
#625=CARTESIAN_POINT ( 'NONE',  ( -4.784657899331157260, -83.89547149457074227, 1.454677039711874675 ) ) ;
#626=CARTESIAN_POINT ( 'NONE',  ( 1.069819614139557062, -76.65452850542925489, 2.969112962950023249 ) ) ;
#629=CARTESIAN_POINT ( 'NONE',  ( 0.09506052544083994083, -85.50452850542926342, 2.999999999999997780 ) ) ;
#630=CARTESIAN_POINT ( 'NONE',  ( 5.895805022753492608, -63.94547149457074653, 4.407101234057782868 ) ) ;
#632=CARTESIAN_POINT ( 'NONE',  ( 2.862020680886598889, -69.79547149457074795, 4.100960146803977580 ) ) ;
#633=CARTESIAN_POINT ( 'NONE',  ( -4.194503406049384431, -62.44547149457072521, -3.171033256558012159 ) ) ;
#638=CARTESIAN_POINT ( 'NONE',  ( -0.09506052544084186984, -63.00452850542925631, -4.999999999999997335 ) ) ;
#639=CARTESIAN_POINT ( 'NONE',  ( -0.09506052544071189048, -93.49547149457075079, 6.999999999999997335 ) ) ;
#642=CARTESIAN_POINT ( 'NONE',  ( -4.725907263620321430, -72.90452850542925489, 1.635492904037698647 ) ) ;
#645=CARTESIAN_POINT ( 'NONE',  ( 4.312004677471013459, -82.54547149457074795, -3.009306630940933314 ) ) ;
#648=CARTESIAN_POINT ( 'NONE',  ( 3.154386672714808437, -73.24547149457075079, 0.09995255151720662534 ) ) ;
#650=CARTESIAN_POINT ( 'NONE',  ( 6.013306294175169597, -73.95452850542925205, 4.245374608440616093 ) ) ;
#651=CARTESIAN_POINT ( 'NONE',  ( -3.015831842038128929, -78.19547149457075363, 3.989209796945492048 ) ) ;
#652=CARTESIAN_POINT ( 'NONE',  ( -2.862020680886496304, -61.20452850542925205, 4.100960146804039752 ) ) ;
#654=CARTESIAN_POINT ( 'NONE',  ( -0.09506052544086177059, -72.00452850542926342, -6.999999999999997335 ) ) ;
#656=CARTESIAN_POINT ( 'NONE',  ( -0.8796985632579414904, -89.14547149457072805, -3.030887037049952326 ) ) ;
#661=CARTESIAN_POINT ( 'NONE',  ( -4.312004677471056979, -84.45452850542922363, -3.009306630940844052 ) ) ;
#663=CARTESIAN_POINT ( 'NONE',  ( -5.257311121191323267, -84.75452850542924921, 0.09995255151729529053 ) ) ;
#664=CARTESIAN_POINT ( 'NONE',  ( -2.610703060766967454, -57.45452850542925916, -1.773238653441072232 ) ) ;
#667=CARTESIAN_POINT ( 'NONE',  ( -1.529537955723668574, -88.35452850542925773, 5.030887037049979860 ) ) ;
#668=CARTESIAN_POINT ( 'NONE',  ( -0.09506052544071454113, -72.49547149457075079, 6.999999999999997335 ) ) ;
#670=CARTESIAN_POINT ( 'NONE',  ( 0.09506052544075563326, -79.99547149457075079, -4.999999999999997335 ) ) ;
#671=CARTESIAN_POINT ( 'NONE',  ( -2.493201789345252717, -73.05452850542926058, 1.934965279058294518 ) ) ;
#676=CARTESIAN_POINT ( 'NONE',  ( 0.09506052544084032940, -88.50452850542926342, 2.999999999999997780 ) ) ;
#677=CARTESIAN_POINT ( 'NONE',  ( 6.013306294175077227, -61.54547149457074084, -4.245374608440741326 ) ) ;
#679=CARTESIAN_POINT ( 'NONE',  ( -4.784657899331190123, -72.60452850542925773, -1.454677039711773867 ) ) ;
#680=CARTESIAN_POINT ( 'NONE',  ( 6.628020296210689999, -97.09547149457074511, 2.253526892787472757 ) ) ;
#683=CARTESIAN_POINT ( 'NONE',  ( -3.015831842038217303, -57.30452850542925347, -3.989209796945429432 ) ) ;
#684=CARTESIAN_POINT ( 'NONE',  ( -6.686770931921456551, -92.89547149457074227, 2.072711028461789784 ) ) ;
#686=CARTESIAN_POINT ( 'NONE',  ( 4.784657899331209663, -74.10452850542925773, 1.454677039711774533 ) ) ;
#689=CARTESIAN_POINT ( 'NONE',  ( -2.862020680886579793, -83.29547149457074795, -4.100960146803977580 ) ) ;
#691=CARTESIAN_POINT ( 'NONE',  ( -2.882544866740859302, -65.89547149457074227, 0.8366430509619596778 ) ) ;
#692=CARTESIAN_POINT ( 'NONE',  ( -6.628020296210622497, -66.90452850542925489, 2.253526892787613978 ) ) ;
#695=CARTESIAN_POINT ( 'NONE',  ( -4.312004677470993030, -78.04547149457076216, 3.009306630940933758 ) ) ;
#696=CARTESIAN_POINT ( 'NONE',  ( -3.015831842038216859, -60.30452850542926058, -3.989209796945429432 ) ) ;
#697=CARTESIAN_POINT ( 'NONE',  ( 4.784657899331212327, -95.10452850542925773, 1.454677039711774533 ) ) ;
#698=CARTESIAN_POINT ( 'NONE',  ( 0.09506052544087986722, -64.50452850542926342, 6.999999999999997335 ) ) ;
#699=CARTESIAN_POINT ( 'NONE',  ( -1.069819614139474240, -81.34547149457074511, 2.969112962950044121 ) ) ;
#704=CARTESIAN_POINT ( 'NONE',  ( 1.719659006605392504, -88.65452850542925489, 4.969112962950016588 ) ) ;
#706=CARTESIAN_POINT ( 'NONE',  ( -1.529537955723669684, -82.35452850542924352, 5.030887037049979860 ) ) ;
#707=CARTESIAN_POINT ( 'NONE',  ( -2.610703060766923933, -96.04547149457074795, 1.773238653441125745 ) ) ;
#709=CARTESIAN_POINT ( 'NONE',  ( -2.862020680886492308, -91.20452850542926626, 4.100960146804039752 ) ) ;
#710=CARTESIAN_POINT ( 'NONE',  ( -0.09506052544071567911, -63.49547149457075079, 6.999999999999997335 ) ) ;
#711=CARTESIAN_POINT ( 'NONE',  ( -0.8796985632578805392, -67.35452850542924352, 3.030887037049973198 ) ) ;
#715=CARTESIAN_POINT ( 'NONE',  ( 2.823794231030041235, -83.40452850542925489, -1.017458915287783316 ) ) ;
#717=CARTESIAN_POINT ( 'NONE',  ( -2.179377348189612817, -62.14547149457074937, -7.030887037049939003 ) ) ;
#720=CARTESIAN_POINT ( 'NONE',  ( -4.784657899331190123, -75.60452850542925773, -1.454677039711773867 ) ) ;
#721=CARTESIAN_POINT ( 'NONE',  ( -6.013306294175058575, -93.04547149457074795, 4.245374608440741326 ) ) ;
#725=( GEOMETRIC_REPRESENTATION_CONTEXT ( 3 ) GLOBAL_UNCERTAINTY_ASSIGNED_CONTEXT ( ( #4274 ) ) GLOBAL_UNIT_ASSIGNED_CONTEXT ( ( #2414, #6289, #2536 ) ) REPRESENTATION_CONTEXT ( 'NONE', 'WORKASPACE' ) );
#727=CARTESIAN_POINT ( 'NONE',  ( -5.257311121191324155, -63.75452850542925631, 0.09995255151729526277 ) ) ;
#728=CARTESIAN_POINT ( 'NONE',  ( -5.895805022753476621, -86.44547149457073942, -4.407101234057782868 ) ) ;
#732=CARTESIAN_POINT ( 'NONE',  ( -1.529537955723670350, -76.35452850542925773, 5.030887037049979860 ) ) ;
#736=CARTESIAN_POINT ( 'NONE',  ( -4.725907263620352516, -83.59547149457074511, -1.635492904037597617 ) ) ;
#738=CARTESIAN_POINT ( 'NONE',  ( -0.09506052544075821453, -63.49547149457075079, 2.999999999999997780 ) ) ;
#739=CARTESIAN_POINT ( 'NONE',  ( 7.360235569667877620, -71.25452850542926342, -0.09995255151731691212 ) ) ;
#741=CARTESIAN_POINT ( 'NONE',  ( 4.784657899331177688, -76.39547149457074227, -1.454677039711874009 ) ) ;
#742=CARTESIAN_POINT ( 'NONE',  ( -5.257311121191324155, -57.75452850542923500, 0.09995255151729526277 ) ) ;
#743=CARTESIAN_POINT ( 'NONE',  ( 0.09506052544086121547, -85.50452850542926342, 4.999999999999997335 ) ) ;
#744=CARTESIAN_POINT ( 'NONE',  ( -7.360235569667860744, -63.75452850542926342, 0.09995255151731782806 ) ) ;
#745=CARTESIAN_POINT ( 'NONE',  ( 2.493201789345310448, -81.94547149457073942, 1.934965279058241006 ) ) ;
#749=CARTESIAN_POINT ( 'NONE',  ( 4.194503406049339134, -86.55452850542926058, -3.171033256558100089 ) ) ;
#751=CARTESIAN_POINT ( 'NONE',  ( -4.784657899331190123, -84.60452850542927195, -1.454677039711773867 ) ) ;
#752=CARTESIAN_POINT ( 'NONE',  ( 0.8796985632579640280, -93.64547149457074227, 3.030887037049952326 ) ) ;
#754=CARTESIAN_POINT ( 'NONE',  ( 4.194503406049339134, -89.55452850542926058, -3.171033256558100089 ) ) ;
#755=CARTESIAN_POINT ( 'NONE',  ( 6.686770931921476979, -61.39547149457074937, -2.072711028461788896 ) ) ;
#756=CARTESIAN_POINT ( 'NONE',  ( -0.8796985632578802061, -70.35452850542922931, 3.030887037049973198 ) ) ;
#757=DIRECTION ( 'NONE',  ( 0.09506052544079829358, -0.9954714945707482388, 0.000000000000000000 ) ) ;
#759=CARTESIAN_POINT ( 'NONE',  ( -2.882544866740877065, -78.60452850542927195, -0.8366430509618996147 ) ) ;
#760=CARTESIAN_POINT ( 'NONE',  ( -5.895805022753383362, -91.05452850542926058, 4.407101234057909878 ) ) ;
#762=CARTESIAN_POINT ( 'NONE',  ( -1.719659006605371854, -78.15452850542925489, -4.969112962950016588 ) ) ;
#763=CARTESIAN_POINT ( 'NONE',  ( 2.369498399071078509, -85.84547149457074511, -6.969112962950057444 ) ) ;
#766=CARTESIAN_POINT ( 'NONE',  ( -2.882544866740858414, -71.89547149457074227, 0.8366430509619596778 ) ) ;
#770=CARTESIAN_POINT ( 'NONE',  ( -3.015831842038215083, -75.30452850542926058, -3.989209796945429432 ) ) ;
#771=CARTESIAN_POINT ( 'NONE',  ( -5.895805022753476621, -92.44547149457073942, -4.407101234057782868 ) ) ;
#775=CARTESIAN_POINT ( 'NONE',  ( -2.862020680886494972, -73.20452850542925205, 4.100960146804039752 ) ) ;
#776=DIRECTION ( 'NONE',  ( -0.9954714945707483498, -0.09506052544079827971, 1.047588144072330487E-14 ) ) ;
#780=CARTESIAN_POINT ( 'NONE',  ( 0.09506052544075563326, -79.99547149457075079, -4.999999999999997335 ) ) ;
#782=CARTESIAN_POINT ( 'NONE',  ( -3.154386672714791118, -65.74547149457073658, -0.09995255151720625064 ) ) ;
#783=CARTESIAN_POINT ( 'NONE',  ( 0.09506052544088025580, -67.50452850542926342, 6.999999999999997335 ) ) ;
#785=CARTESIAN_POINT ( 'NONE',  ( 1.719659006605286145, -79.84547149457071669, -4.969112962950050338 ) ) ;
#786=CARTESIAN_POINT ( 'NONE',  ( 5.257311121191341918, -83.25452850542926342, -0.09995255151729465215 ) ) ;
#787=CARTESIAN_POINT ( 'NONE',  ( 4.191402346623196884, -67.80452850542926058, 5.607243785695311900 ) ) ;
#788=CARTESIAN_POINT ( 'NONE',  ( 0.09506052544077704669, -82.99547149457075079, -2.999999999999997780 ) ) ;
#793=CARTESIAN_POINT ( 'NONE',  ( 1.719659006605392504, -91.65452850542925489, 4.969112962950016588 ) ) ;
#795=CARTESIAN_POINT ( 'NONE',  ( 2.862020680886514956, -83.70452850542925205, -4.100960146804039752 ) ) ;
#796=CARTESIAN_POINT ( 'NONE',  ( -0.09506052544075442590, -93.49547149457075079, 2.999999999999997780 ) ) ;
#797=( BOUNDED_CURVE ( )  B_SPLINE_CURVE ( 2, ( #2958, #3507, #1099, #5525, #1568, #4134, #4935, #2251, #340, #1058, #6197, #7508, #6076, #8024, #422, #8105, #977, #8062, #4806, #3630, #4214, #2293, #300, #3544, #6114, #2917, #6787, #5483, #1020, #2331, #4896, #1699, #4255, #6825, #2996, #3671, #1738, #4296, #6239, #5562, #587, #5679, #5643, #1951, #6408, #1227, #2533, #2575, #7588, #7675, #5013, #4335, #6368, #3797, #4502, #5055, #1145, #2288, #7081, #5601, #6327, #3167, #5722, #1267, #546, #4973, #5136, #464, #7631, #1824, #8301, #7548, #5095, #3208, #3123, #4456, #1866, #1907, #3714, #2494, #1185, #7715, #4414, #6996, #7038, #1307, #3838, #4376, #625, #3879, #5764, #1779, #3039, #8182, #6909, #6951, #2410, #6284, #502, #3080, #8222, #2451, #3754, #8262, #5807, #6449, #36, #2622, #5182, #7761, #1992, #1351, #4541, #7124, #670, #3251, #6797, #945, #5570, #1578, #3005, #7436, #6165, #2303, #6124, #8153, #7352, #6084, #5409, #3516, #4184, #4144, #6755, #1028, #6877, #4907, #7989, #987, #4226, #6714, #2382, #390, #8033, #309, #2886, #268, #4263, #3554, #2217, #3597, #1108, #3642, #4776, #4865, #5454, #2848, #2260, #4816, #8114, #5532, #7394, #349, #6836, #1624, #2339, #2927, #5492, #1664, #8073, #6042, #4942, #2967, #1068, #7479, #1707, #6207, #431, #7516, #1747, #4305, #3049, #5687, #632, #3, #6374, #4509, #4983, #2540, #6251, #6336, #8190, #3845, #5729, #1193, #511, #4467, #8310, #3764, #2461, #554, #473, #8230, #7724, #1959, #5104, #5022, #7006, #7088, #8270, #7557, #6414, #3216, #1789, #7598, #2501, #5611, #2420, #6293, #5773, #3090, #595, #4344, #3680, #1233, #6920, #1155, #2582, #5650, #3132, #1915, #7046, #5145, #3723, #1834, #1276, #3804, #4385, #5062, #6961, #7641, #1874, #4422, #3174, #7682, #3073, #1259, #7073, #1178, #1858, #1817, #4407, #7030, #4534, #2569, #5635 ),
 .UNSPECIFIED., .F., .T. ) 
 B_SPLINE_CURVE_WITH_KNOTS ( ( 3, 2, 2, 2, 2, 2, 2, 2, 2, 2, 2, 2, 2, 2, 2, 2, 2, 2, 2, 2, 2, 2, 2, 2, 2, 2, 2, 2, 2, 2, 2, 2, 2, 2, 2, 2, 2, 2, 2, 2, 2, 2, 2, 2, 2, 2, 2, 2, 2, 2, 2, 2, 2, 2, 2, 2, 2, 2, 2, 2, 2, 2, 2, 2, 2, 2, 2, 2, 2, 2, 2, 2, 2, 2, 2, 2, 2, 2, 2, 2, 2, 2, 2, 2, 2, 2, 2, 2, 2, 2, 2, 2, 2, 2, 2, 2, 2, 2, 2, 2, 2, 2, 2, 2, 2, 2, 2, 2, 2, 2, 2, 2, 2, 2, 2, 2, 2, 2, 2, 2, 2, 2, 2, 2, 2, 2, 2, 3 ),
 ( 0.02555479535913396730, 0.03076923076923077094, 0.03846153846153846367, 0.04615384615384615641, 0.05384615384615384914, 0.06153846153846154188, 0.06923076923076923461, 0.07692307692307692735, 0.08461538461538462008, 0.09230769230769231282, 0.1000000000000000056, 0.1076923076923076983, 0.1153846153846153910, 0.1230769230769230838, 0.1307692307692307765, 0.1384615384615384692, 0.1461538461538461620, 0.1538461538461538547, 0.1615384615384615197, 0.1692307692307692402, 0.1769230769230769329, 0.1846153846153846256, 0.1923076923076923184, 0.2000000000000000111, 0.2076923076923077038, 0.2153846153846153966, 0.2230769230769230893, 0.2307692307692307820, 0.2384615384615384748, 0.2461538461538461675, 0.2538461538461538325, 0.2615384615384615530, 0.2692307692307692180, 0.2769230769230769384, 0.2846153846153846034, 0.2923076923076923239, 0.2999999999999999889, 0.3076923076923077094, 0.3153846153846153744, 0.3230769230769230949, 0.3307692307692307598, 0.3384615384615384803, 0.3461538461538461453, 0.3538461538461539213, 0.3615384615384615308, 0.3692307692307692513, 0.3769230769230769162, 0.3846153846153846367, 0.3923076923076923017, 0.4000000000000000222, 0.4076923076923076872, 0.4153846153846154077, 0.4230769230769230727, 0.4307692307692307931, 0.4384615384615384581, 0.4461538461538461786, 0.4538461538461538436, 0.4615384615384615641, 0.4692307692307692291, 0.4769230769230769496, 0.4846153846153846145, 0.4923076923076923350, 0.5000000000000000000, 0.5076923076923076650, 0.5153846153846153300, 0.5230769230769231060, 0.5307692307692307709, 0.5384615384615384359, 0.5461538461538461009, 0.5538461538461538769, 0.5615384615384615419, 0.5692307692307692069, 0.5769230769230768718, 0.5846153846153846478, 0.5923076923076923128, 0.5999999999999999778, 0.6076923076923076428, 0.6153846153846154188, 0.6230769230769230838, 0.6307692307692307487, 0.6384615384615384137, 0.6461538461538461897, 0.6538461538461538547, 0.6615384615384615197, 0.6692307692307691847, 0.6769230769230769607, 0.6846153846153846256, 0.6923076923076922906, 0.6999999999999999556, 0.7076923076923077316, 0.7153846153846153966, 0.7230769230769230616, 0.7307692307692307265, 0.7384615384615385025, 0.7461538461538461675, 0.7538461538461538325, 0.7615384615384614975, 0.7692307692307692735, 0.7769230769230769384, 0.7846153846153846034, 0.7923076923076922684, 0.8000000000000000444, 0.8076923076923077094, 0.8153846153846153744, 0.8230769230769230393, 0.8307692307692308153, 0.8384615384615384803, 0.8461538461538461453, 0.8538461538461538103, 0.8615384615384615863, 0.8692307692307692513, 0.8769230769230769162, 0.8846153846153845812, 0.8923076923076923572, 0.9000000000000000222, 0.9076923076923076872, 0.9153846153846153522, 0.9230769230769231282, 0.9307692307692307931, 0.9384615384615384581, 0.9461538461538461231, 0.9538461538461538991, 0.9615384615384615641, 0.9692307692307692291, 0.9769230769230768940, 0.9846153846153846700, 0.9923076923076923350, 1.000000000000000000 ),
 .UNSPECIFIED. ) 
 CURVE ( )  GEOMETRIC_REPRESENTATION_ITEM ( )  RATIONAL_B_SPLINE_CURVE ( ( 0.9786254102152882606, 0.9668223575118739532, 1.000000000000000000, 0.9510565162951535312, 1.000000000000000000, 0.9510565162951535312, 1.000000000000000000, 0.9510565162951535312, 1.000000000000000000, 0.9510565162951535312, 1.000000000000000000, 0.9510565162951535312, 1.000000000000000000, 0.9510565162951535312, 1.000000000000000000, 0.9510565162951535312, 1.000000000000000000, 0.9510565162951535312, 1.000000000000000000, 0.9510565162951535312, 1.000000000000000000, 0.9510565162951535312, 1.000000000000000000, 0.9510565162951535312, 1.000000000000000000, 0.9510565162951535312, 1.000000000000000000, 0.9510565162951535312, 1.000000000000000000, 0.9510565162951535312, 1.000000000000000000, 0.9510565162951535312, 1.000000000000000000, 0.9510565162951535312, 1.000000000000000000, 0.9510565162951535312, 1.000000000000000000, 0.9510565162951535312, 1.000000000000000000, 0.9510565162951535312, 1.000000000000000000, 0.9510565162951535312, 1.000000000000000000, 0.9510565162951535312, 1.000000000000000000, 0.9510565162951535312, 1.000000000000000000, 0.9510565162951535312, 1.000000000000000000, 0.9510565162951535312, 1.000000000000000000, 0.9510565162951535312, 1.000000000000000000, 0.9510565162951535312, 1.000000000000000000, 0.9510565162951535312, 1.000000000000000000, 0.9510565162951535312, 1.000000000000000000, 0.9510565162951535312, 1.000000000000000000, 0.9510565162951535312, 1.000000000000000000, 0.9510565162951535312, 1.000000000000000000, 0.9510565162951535312, 1.000000000000000000, 0.9510565162951535312, 1.000000000000000000, 0.9510565162951535312, 1.000000000000000000, 0.9510565162951535312, 1.000000000000000000, 0.9510565162951535312, 1.000000000000000000, 0.9510565162951535312, 1.000000000000000000, 0.9510565162951535312, 1.000000000000000000, 0.9510565162951535312, 1.000000000000000000, 0.9510565162951535312, 1.000000000000000000, 0.9510565162951535312, 1.000000000000000000, 0.9510565162951535312, 1.000000000000000000, 0.9510565162951535312, 1.000000000000000000, 0.9510565162951535312, 1.000000000000000000, 0.9510565162951535312, 1.000000000000000000, 0.9510565162951535312, 1.000000000000000000, 0.9510565162951535312, 1.000000000000000000, 0.9510565162951535312, 1.000000000000000000, 0.9510565162951535312, 1.000000000000000000, 0.9510565162951535312, 1.000000000000000000, 0.9510565162951535312, 1.000000000000000000, 0.9510565162951535312, 1.000000000000000000, 0.9510565162951535312, 1.000000000000000000, 0.9510565162951535312, 1.000000000000000000, 0.9510565162951535312, 1.000000000000000000, 0.9510565162951535312, 1.000000000000000000, 0.9510565162951535312, 1.000000000000000000, 0.9510565162951535312, 1.000000000000000000, 0.9510565162951535312, 1.000000000000000000, 0.9510565162951535312, 1.000000000000000000, 0.9510565162951535312, 1.000000000000000000, 0.9510565162951535312, 1.000000000000000000, 0.9510565162951535312, 1.000000000000000000, 0.9510565162951535312, 1.000000000000000000, 0.9510565162951535312, 1.000000000000000000, 0.9510565162951535312, 1.000000000000000000, 0.9510565162951535312, 1.000000000000000000, 0.9510565162951535312, 1.000000000000000000, 0.9510565162951535312, 1.000000000000000000, 0.9510565162951535312, 1.000000000000000000, 0.9510565162951535312, 1.000000000000000000, 0.9510565162951535312, 1.000000000000000000, 0.9510565162951535312, 1.000000000000000000, 0.9510565162951535312, 1.000000000000000000, 0.9510565162951535312, 1.000000000000000000, 0.9510565162951535312, 1.000000000000000000, 0.9510565162951535312, 1.000000000000000000, 0.9510565162951535312, 1.000000000000000000, 0.9510565162951535312, 1.000000000000000000, 0.9510565162951535312, 1.000000000000000000, 0.9510565162951535312, 1.000000000000000000, 0.9510565162951535312, 1.000000000000000000, 0.9510565162951535312, 1.000000000000000000, 0.9510565162951535312, 1.000000000000000000, 0.9510565162951535312, 1.000000000000000000, 0.9510565162951535312, 1.000000000000000000, 0.9510565162951535312, 1.000000000000000000, 0.9510565162951535312, 1.000000000000000000, 0.9510565162951535312, 1.000000000000000000, 0.9510565162951535312, 1.000000000000000000, 0.9510565162951535312, 1.000000000000000000, 0.9510565162951535312, 1.000000000000000000, 0.9510565162951535312, 1.000000000000000000, 0.9510565162951535312, 1.000000000000000000, 0.9510565162951535312, 1.000000000000000000, 0.9510565162951535312, 1.000000000000000000, 0.9510565162951535312, 1.000000000000000000, 0.9510565162951535312, 1.000000000000000000, 0.9510565162951535312, 1.000000000000000000, 0.9510565162951535312, 1.000000000000000000, 0.9510565162951535312, 1.000000000000000000, 0.9510565162951535312, 1.000000000000000000, 0.9510565162951535312, 1.000000000000000000, 0.9510565162951535312, 1.000000000000000000, 0.9510565162951535312, 1.000000000000000000, 0.9510565162951535312, 1.000000000000000000, 0.9510565162951535312, 1.000000000000000000, 0.9510565162951535312, 1.000000000000000000, 0.9510565162951535312, 1.000000000000000000, 0.9510565162951535312, 1.000000000000000000, 0.9510565162951535312, 1.000000000000000000, 0.9510565162951535312, 1.000000000000000000, 0.9510565162951535312, 1.000000000000000000, 0.9510565162951535312, 1.000000000000000000, 0.9510565162951535312, 1.000000000000000000, 0.9510565162951535312, 1.000000000000000000, 0.9510565162951535312, 1.000000000000000000, 0.9510565162951535312, 1.000000000000000000, 0.9510565162951535312, 1.000000000000000000, 0.9510565162951535312, 1.000000000000000000, 0.9510565162951535312, 1.000000000000000000, 0.9510565162951535312, 1.000000000000000000, 0.9510565162951535312, 1.000000000000000000, 0.9510565162951535312, 1.000000000000000000, 0.9510565162951535312, 1.000000000000000000, 0.9510565162951535312, 1.000000000000000000 ) ) 
 REPRESENTATION_ITEM ( '' )  );
#799=CARTESIAN_POINT ( 'NONE',  ( 4.784657899331211439, -89.10452850542925773, 1.454677039711774533 ) ) ;
#801=CARTESIAN_POINT ( 'NONE',  ( -2.369498399071204631, -93.15452850542925489, -6.969112962950009482 ) ) ;
#803=CARTESIAN_POINT ( 'NONE',  ( 2.882544866740894829, -62.10452850542925063, 0.8366430509618999478 ) ) ;
#808=CARTESIAN_POINT ( 'NONE',  ( 1.840261337453270807, -76.80452850542926058, 2.371175808195547852 ) ) ;
#809=CARTESIAN_POINT ( 'NONE',  ( -6.686770931921503625, -87.60452850542924352, -2.072711028461647675 ) ) ;
#811=CARTESIAN_POINT ( 'NONE',  ( -5.895805022753476621, -92.44547149457073942, -4.407101234057782868 ) ) ;
#814=CARTESIAN_POINT ( 'NONE',  ( -2.493201789345292241, -68.44547149457073942, -1.934965279058240561 ) ) ;
#817=CARTESIAN_POINT ( 'NONE',  ( 4.784657899331208775, -68.10452850542925773, 1.454677039711774533 ) ) ;
#818=CARTESIAN_POINT ( 'NONE',  ( -2.179377348189610153, -83.14547149457072805, -7.030887037049939003 ) ) ;
#820=CARTESIAN_POINT ( 'NONE',  ( -4.312004677471057867, -78.45452850542925205, -3.009306630940844052 ) ) ;
#822=CARTESIAN_POINT ( 'NONE',  ( -3.015831842038130262, -66.19547149457075363, 3.989209796945492048 ) ) ;
#824=CARTESIAN_POINT ( 'NONE',  ( -0.09506052544075783983, -66.49547149457075079, 2.999999999999997780 ) ) ;
#825=CARTESIAN_POINT ( 'NONE',  ( -2.179377348189462271, -67.35452850542924352, 7.030887037049988741 ) ) ;
#829=CARTESIAN_POINT ( 'NONE',  ( 4.312004677471078296, -88.95452850542922363, 3.009306630940844496 ) ) ;
#830=CARTESIAN_POINT ( 'NONE',  ( 6.686770931921523164, -65.10452850542924352, 2.072711028461649008 ) ) ;
#831=CARTESIAN_POINT ( 'NONE',  ( 2.823794231030060331, -79.09547149457075932, 1.017458915287723809 ) ) ;
#834=CARTESIAN_POINT ( 'NONE',  ( 1.529537955723692999, -95.85452850542922931, -5.030887037049978971 ) ) ;
#835=CARTESIAN_POINT ( 'NONE',  ( 0.09506052544086197875, -91.50452850542924921, 4.999999999999997335 ) ) ;
#837=CARTESIAN_POINT ( 'NONE',  ( -5.257311121191325043, -72.75452850542924921, 0.09995255151729529053 ) ) ;
#838=CARTESIAN_POINT ( 'NONE',  ( 0.8796985632579634729, -90.64547149457075648, 3.030887037049952326 ) ) ;
#839=CARTESIAN_POINT ( 'NONE',  ( -4.194503406049316041, -85.05452850542926058, 3.171033256558100533 ) ) ;
#840=CARTESIAN_POINT ( 'NONE',  ( -4.037591185471547384, -59.29547149457074084, -5.718994135553860936 ) ) ;
#841=CARTESIAN_POINT ( 'NONE',  ( 0.09506052544083729017, -64.50452850542926342, 2.999999999999997780 ) ) ;
#846=CARTESIAN_POINT ( 'NONE',  ( 1.686450176301585335, -74.70452850542925205, -2.482926158054133303 ) ) ;
#847=CARTESIAN_POINT ( 'NONE',  ( -4.037591185471421262, -88.20452850542925205, 5.718994135553947977 ) ) ;
#848=CARTESIAN_POINT ( 'NONE',  ( -4.037591185471543831, -86.29547149457074795, -5.718994135553860936 ) ) ;
#851=CARTESIAN_POINT ( 'NONE',  ( 3.154386672714807105, -64.24547149457075079, 0.09995255151720662534 ) ) ;
#855=CARTESIAN_POINT ( 'NONE',  ( 4.725907263620340082, -68.40452850542925489, -1.635492904037697981 ) ) ;
#856=CARTESIAN_POINT ( 'NONE',  ( -2.369498399071056305, -81.34547149457074511, 6.969112962950058332 ) ) ;
#859=CARTESIAN_POINT ( 'NONE',  ( -2.862020680886495416, -67.20452850542925205, 4.100960146804039752 ) ) ;
#865=CARTESIAN_POINT ( 'NONE',  ( 5.257311121191341918, -70.24547149457075079, 0.09995255151718437925 ) ) ;
#868=CARTESIAN_POINT ( 'NONE',  ( 2.610703060766943029, -61.54547149457074084, -1.773238653441125523 ) ) ;
#869=CARTESIAN_POINT ( 'NONE',  ( -6.628020296210623385, -60.90452850542925489, 2.253526892787613978 ) ) ;
#870=EDGE_LOOP ( 'NONE', ( #2926, #8293, #8072, #1678, #8003 ) ) ;
#872=CARTESIAN_POINT ( 'NONE',  ( 1.719659006605392060, -85.65452850542922647, 4.969112962950016588 ) ) ;
#873=CARTESIAN_POINT ( 'NONE',  ( -6.686770931921507177, -63.60452850542924352, -2.072711028461647675 ) ) ;
#874=CARTESIAN_POINT ( 'NONE',  ( 3.154386672714809325, -76.24547149457073658, 0.09995255151720662534 ) ) ;
#878=CARTESIAN_POINT ( 'NONE',  ( 3.015831842038234178, -79.80452850542926058, 3.989209796945429432 ) ) ;
#881=CARTESIAN_POINT ( 'NONE',  ( 3.015831842038233734, -73.80452850542926058, 3.989209796945429432 ) ) ;
#882=CARTESIAN_POINT ( 'NONE',  ( -2.823794231030039015, -86.59547149457075932, -1.017458915287723364 ) ) ;
#884=CARTESIAN_POINT ( 'NONE',  ( 1.529537955723798026, -96.64547149457071384, 5.030887037049945221 ) ) ;
#885=CARTESIAN_POINT ( 'NONE',  ( -0.09506052544085913381, -93.00452850542926342, -6.999999999999997335 ) ) ;
#886=CARTESIAN_POINT ( 'NONE',  ( -3.154386672714790674, -69.75452850542926342, 0.09995255151727280851 ) ) ;
#890=CARTESIAN_POINT ( 'NONE',  ( 3.154386672714809325, -77.25452850542924921, -0.09995255151727241993 ) ) ;
#891=CARTESIAN_POINT ( 'NONE',  ( 6.628020296210642037, -89.40452850542926910, -2.253526892787612645 ) ) ;
#892=CARTESIAN_POINT ( 'NONE',  ( -2.369498399071055417, -90.34547149457073090, 6.969112962950058332 ) ) ;
#895=CARTESIAN_POINT ( 'NONE',  ( -0.8796985632579434888, -71.14547149457074227, -3.030887037049952326 ) ) ;
#900=CARTESIAN_POINT ( 'NONE',  ( 4.312004677471073855, -64.95452850542926626, 3.009306630940844496 ) ) ;
#901=CARTESIAN_POINT ( 'NONE',  ( -7.360235569667858968, -80.74547149457075079, -0.09995255151716124498 ) ) ;
#905=CARTESIAN_POINT ( 'NONE',  ( -4.725907263620322318, -69.90452850542925489, 1.635492904037698647 ) ) ;
#907=CARTESIAN_POINT ( 'NONE',  ( 2.862020680886598445, -66.79547149457073374, 4.100960146803977580 ) ) ;
#909=CARTESIAN_POINT ( 'NONE',  ( 4.312004677471013459, -94.54547149457071953, -3.009306630940933314 ) ) ;
#910=CARTESIAN_POINT ( 'NONE',  ( -2.369498399071207739, -63.15452850542925489, -6.969112962950009482 ) ) ;
#911=ORIENTED_EDGE ( 'NONE', *, *, #7757, .T. ) ;
#913=CARTESIAN_POINT ( 'NONE',  ( 5.257311121191341918, -80.25452850542922079, -0.09995255151729465215 ) ) ;
#916=CARTESIAN_POINT ( 'NONE',  ( 4.725907263620341858, -86.40452850542926910, -1.635492904037697981 ) ) ;
#917=CARTESIAN_POINT ( 'NONE',  ( 2.862020680886514512, -77.70452850542926626, -4.100960146804039752 ) ) ;
#919=CARTESIAN_POINT ( 'NONE',  ( -4.194503406049319594, -70.05452850542924637, 3.171033256558101865 ) ) ;
#920=CARTESIAN_POINT ( 'NONE',  ( -1.840261337453198864, -87.19547149457073942, 2.371175808195584267 ) ) ;
#921=CARTESIAN_POINT ( 'NONE',  ( -2.610703060766927930, -63.04547149457074084, 1.773238653441125745 ) ) ;
#922=CARTESIAN_POINT ( 'NONE',  ( -4.784657899331190123, -78.60452850542925773, -1.454677039711773867 ) ) ;
#923=CARTESIAN_POINT ( 'NONE',  ( -5.895805022753383362, -91.05452850542926058, 4.407101234057909878 ) ) ;
#924=CARTESIAN_POINT ( 'NONE',  ( 2.882544866740894385, -59.10452850542926484, 0.8366430509618999478 ) ) ;
#929=CARTESIAN_POINT ( 'NONE',  ( 2.823794231030039903, -74.40452850542925489, -1.017458915287783316 ) ) ;
#930=CARTESIAN_POINT ( 'NONE',  ( 4.037591185471444355, -89.70452850542925205, -5.718994135553947977 ) ) ;
#933=CARTESIAN_POINT ( 'NONE',  ( 6.013306294175080779, -82.54547149457074795, -4.245374608440741326 ) ) ;
#936=CARTESIAN_POINT ( 'NONE',  ( 0.8796985632579601422, -63.64547149457072805, 3.030887037049952326 ) ) ;
#941=CARTESIAN_POINT ( 'NONE',  ( -4.194503406049320482, -64.05452850542926058, 3.171033256558100533 ) ) ;
#942=CARTESIAN_POINT ( 'NONE',  ( 2.179377348189629693, -78.64547149457074227, 7.030887037049939003 ) ) ;
#945=CARTESIAN_POINT ( 'NONE',  ( 4.312004677471011682, -79.54547149457074795, -3.009306630940932425 ) ) ;
#946=CARTESIAN_POINT ( 'NONE',  ( -1.529537955723777598, -74.14547149457074227, -5.030887037049945221 ) ) ;
#947=CARTESIAN_POINT ( 'NONE',  ( -4.725907263620322318, -66.90452850542925489, 1.635492904037698647 ) ) ;
#951=CARTESIAN_POINT ( 'NONE',  ( -3.015831842038129817, -72.19547149457073942, 3.989209796945492048 ) ) ;
#953=CARTESIAN_POINT ( 'NONE',  ( -0.09506052544086292244, -63.00452850542925631, -6.999999999999997335 ) ) ;
#958=CARTESIAN_POINT ( 'NONE',  ( 4.312004677471078296, -85.95452850542925205, 3.009306630940844496 ) ) ;
#959=CARTESIAN_POINT ( 'NONE',  ( 4.725907263620340970, -80.40452850542925489, -1.635492904037697981 ) ) ;
#962=CARTESIAN_POINT ( 'NONE',  ( -4.312004677471058756, -69.45452850542925205, -3.009306630940843608 ) ) ;
#963=CARTESIAN_POINT ( 'NONE',  ( 1.069819614139495112, -82.84547149457074511, -2.969112962950042789 ) ) ;
#964=CARTESIAN_POINT ( 'NONE',  ( -1.840261337453202195, -63.19547149457074653, 2.371175808195584267 ) ) ;
#965=CARTESIAN_POINT ( 'NONE',  ( -4.312004677471057867, -75.45452850542925205, -3.009306630940844052 ) ) ;
#966=CARTESIAN_POINT ( 'NONE',  ( 6.686770931921525829, -86.10452850542924352, 2.072711028461649008 ) ) ;
#967=CARTESIAN_POINT ( 'NONE',  ( 1.840261337453222179, -94.69547149457076785, -2.371175808195584267 ) ) ;
#972=CARTESIAN_POINT ( 'NONE',  ( -2.493201789345253605, -64.05452850542924637, 1.934965279058294518 ) ) ;
#973=CARTESIAN_POINT ( 'NONE',  ( -4.037591185471423039, -76.20452850542925205, 5.718994135553947977 ) ) ;
#975=CARTESIAN_POINT ( 'NONE',  ( 6.686770931921479644, -82.39547149457074227, -2.072711028461788896 ) ) ;
#977=CARTESIAN_POINT ( 'NONE',  ( 3.015831842038151134, -94.69547149457075363, -3.989209796945492048 ) ) ;
#978=CARTESIAN_POINT ( 'NONE',  ( 1.840261337453271473, -82.80452850542926058, 2.371175808195547852 ) ) ;
#983=CARTESIAN_POINT ( 'NONE',  ( -0.09506052544084110656, -69.00452850542926342, -4.999999999999997335 ) ) ;
#984=CARTESIAN_POINT ( 'NONE',  ( -2.179377348189610597, -77.14547149457074227, -7.030887037049939003 ) ) ;
#987=CARTESIAN_POINT ( 'NONE',  ( 4.312004677471011682, -76.54547149457073374, -3.009306630940932425 ) ) ;
#988=CARTESIAN_POINT ( 'NONE',  ( 4.312004677471011682, -70.54547149457074795, -3.009306630940933314 ) ) ;
#989=CARTESIAN_POINT ( 'NONE',  ( 5.257311121191341918, -62.25452850542924921, -0.09995255151729465215 ) ) ;
#993=CARTESIAN_POINT ( 'NONE',  ( 3.015831842038147581, -67.69547149457073942, -3.989209796945492048 ) ) ;
#995=CARTESIAN_POINT ( 'NONE',  ( -4.191402346623181785, -57.30452850542924637, -5.607243785695311900 ) ) ;
#1001=CARTESIAN_POINT ( 'NONE',  ( 3.015831842038235511, -88.80452850542926058, 3.989209796945429432 ) ) ;
#1002=CARTESIAN_POINT ( 'NONE',  ( -2.862020680886493640, -82.20452850542925205, 4.100960146804039752 ) ) ;
#1004=CARTESIAN_POINT ( 'NONE',  ( 4.312004677471076519, -73.95452850542926626, 3.009306630940844052 ) ) ;
#1005=CARTESIAN_POINT ( 'NONE',  ( 0.09506052544077629729, -76.99547149457075079, -2.999999999999997780 ) ) ;
#1007=CARTESIAN_POINT ( 'NONE',  ( 1.719659006605287921, -97.84547149457071669, -4.969112962950050338 ) ) ;
#1008=CARTESIAN_POINT ( 'NONE',  ( -4.784657899331191899, -63.60452850542925063, -1.454677039711773867 ) ) ;
#1009=CARTESIAN_POINT ( 'NONE',  ( 6.686770931921525829, -89.10452850542925773, 2.072711028461649008 ) ) ;
#1010=CARTESIAN_POINT ( 'NONE',  ( -1.840261337453253931, -60.30452850542926058, -2.371175808195547852 ) ) ;
#1015=CARTESIAN_POINT ( 'NONE',  ( 2.862020680886516732, -95.70452850542926626, -4.100960146804039752 ) ) ;
#1016=CARTESIAN_POINT ( 'NONE',  ( 2.882544866740895717, -68.10452850542924352, 0.8366430509618999478 ) ) ;
#1017=CARTESIAN_POINT ( 'NONE',  ( -6.686770931921458327, -83.89547149457074227, 2.072711028461789784 ) ) ;
#1020=CARTESIAN_POINT ( 'NONE',  ( -4.784657899331156372, -92.89547149457075648, 1.454677039711874675 ) ) ;
#1021=CARTESIAN_POINT ( 'NONE',  ( -2.882544866740875733, -87.60452850542924352, -0.8366430509618996147 ) ) ;
#1025=CARTESIAN_POINT ( 'NONE',  ( 0.8796985632579013004, -95.85452850542924352, -3.030887037049972310 ) ) ;
#1026=CARTESIAN_POINT ( 'NONE',  ( -7.360235569667858968, -74.74547149457073658, -0.09995255151716124498 ) ) ;
#1028=CARTESIAN_POINT ( 'NONE',  ( -1.529537955723777154, -77.14547149457074227, -5.030887037049945221 ) ) ;
#1029=CARTESIAN_POINT ( 'NONE',  ( 2.862020680886598445, -66.79547149457073374, 4.100960146803977580 ) ) ;
#1030=CARTESIAN_POINT ( 'NONE',  ( 4.725907263620339194, -62.40452850542925489, -1.635492904037697981 ) ) ;
#1033=CARTESIAN_POINT ( 'NONE',  ( -4.194503406049384431, -65.44547149457072521, -3.171033256558012159 ) ) ;
#1035=CARTESIAN_POINT ( 'NONE',  ( -5.895805022753386915, -64.05452850542924637, 4.407101234057909878 ) ) ;
#1042=CARTESIAN_POINT ( 'NONE',  ( -4.194503406049315153, -91.05452850542923215, 3.171033256558100533 ) ) ;
#1043=CARTESIAN_POINT ( 'NONE',  ( 1.719659006605391616, -82.65452850542925489, 4.969112962950016588 ) ) ;
#1044=CARTESIAN_POINT ( 'NONE',  ( 1.529537955723689002, -65.85452850542922931, -5.030887037049978971 ) ) ;
#1045=CARTESIAN_POINT ( 'NONE',  ( 2.882544866740877509, -76.39547149457074227, -0.8366430509619593447 ) ) ;
#1046=CARTESIAN_POINT ( 'NONE',  ( 4.194503406049402194, -93.94547149457075363, 3.171033256558012159 ) ) ;
#1047=CARTESIAN_POINT ( 'NONE',  ( -5.257311121191324155, -69.75452850542926342, 0.09995255151729526277 ) ) ;
#1048=CARTESIAN_POINT ( 'NONE',  ( -6.013306294175149169, -90.45452850542926626, -4.245374608440613429 ) ) ;
#1050=CARTESIAN_POINT ( 'NONE',  ( 2.493201789345311781, -93.94547149457073942, 1.934965279058241006 ) ) ;
#1054=CARTESIAN_POINT ( 'NONE',  ( 2.862020680886516288, -92.70452850542926626, -4.100960146804039752 ) ) ;
#1055=CARTESIAN_POINT ( 'NONE',  ( 2.823794231030039459, -68.40452850542925489, -1.017458915287783316 ) ) ;
#1056=CARTESIAN_POINT ( 'NONE',  ( 4.191402346623079644, -82.69547149457073942, -5.607243785695398941 ) ) ;
#1057=FACE_OUTER_BOUND ( 'NONE', #2231, .T. ) ;
#1058=CARTESIAN_POINT ( 'NONE',  ( -5.257311121191321490, -95.74547149457072237, -0.09995255151718372699 ) ) ;
#1059=CARTESIAN_POINT ( 'NONE',  ( 0.09506052544083956612, -82.50452850542926342, 2.999999999999997780 ) ) ;
#1064=CARTESIAN_POINT ( 'NONE',  ( -2.493201789345250052, -94.05452850542926058, 1.934965279058294518 ) ) ;
#1065=CARTESIAN_POINT ( 'NONE',  ( 6.013306294175077227, -70.54547149457074795, -4.245374608440741326 ) ) ;
#1066=SHAPE_REPRESENTATION ( 'return spring', ( #2840 ), #3385 ) ;
#1067=CARTESIAN_POINT ( 'NONE',  ( 3.783624887602714981, -96.99999999999998579, -4.615931839566195904 ) ) ;
#1068=CARTESIAN_POINT ( 'NONE',  ( -2.862020680886581125, -71.29547149457074795, -4.100960146803977580 ) ) ;
#1069=CARTESIAN_POINT ( 'NONE',  ( 4.194503406049400418, -66.94547149457075363, 3.171033256558012159 ) ) ;
#1070=CARTESIAN_POINT ( 'NONE',  ( 4.312004677471073855, -58.95452850542925205, 3.009306630940844496 ) ) ;
#1074=CARTESIAN_POINT ( 'NONE',  ( 7.360235569667880284, -97.24547149457075079, 0.09995255151716216091 ) ) ;
#1075=CARTESIAN_POINT ( 'NONE',  ( -3.015831842038213306, -93.30452850542926058, -3.989209796945429432 ) ) ;
#1082=CARTESIAN_POINT ( 'NONE',  ( 1.719659006605392060, -85.65452850542922647, 4.969112962950016588 ) ) ;
#1083=CARTESIAN_POINT ( 'NONE',  ( -4.784657899331156372, -89.89547149457075648, 1.454677039711874675 ) ) ;
#1084=CARTESIAN_POINT ( 'NONE',  ( 1.529537955723688780, -62.85452850542924352, -5.030887037049978971 ) ) ;
#1085=CARTESIAN_POINT ( 'NONE',  ( -2.610703060766925265, -84.04547149457074795, 1.773238653441125745 ) ) ;
#1086=CARTESIAN_POINT ( 'NONE',  ( -1.529537955723774711, -92.14547149457071384, -5.030887037049945221 ) ) ;
#1087=CARTESIAN_POINT ( 'NONE',  ( 3.015831842038232846, -67.80452850542926058, 3.989209796945429432 ) ) ;
#1088=CARTESIAN_POINT ( 'NONE',  ( -4.037591185471421262, -88.20452850542925205, 5.718994135553947977 ) ) ;
#1089=CARTESIAN_POINT ( 'NONE',  ( 1.069819614139496666, -94.84547149457073090, -2.969112962950042789 ) ) ;
#1093=CARTESIAN_POINT ( 'NONE',  ( 3.015831842038235955, -91.80452850542926058, 3.989209796945429432 ) ) ;
#1094=CARTESIAN_POINT ( 'NONE',  ( 1.069819614139555730, -64.65452850542924068, 2.969112962950023249 ) ) ;
#1095=CARTESIAN_POINT ( 'NONE',  ( 5.257311121191342806, -92.25452850542922079, -0.09995255151729465215 ) ) ;
#1096=CARTESIAN_POINT ( 'NONE',  ( -7.360235569667858968, -74.74547149457073658, -0.09995255151716124498 ) ) ;
#1097=CARTESIAN_POINT ( 'NONE',  ( -1.529537955723667908, -94.35452850542922931, 5.030887037049979860 ) ) ;
#1099=CARTESIAN_POINT ( 'NONE',  ( 2.862020680886601998, -96.79547149457073374, 4.100960146803977580 ) ) ;
#1100=CARTESIAN_POINT ( 'NONE',  ( -2.493201789345250940, -85.05452850542926058, 1.934965279058294518 ) ) ;
#1103=CARTESIAN_POINT ( 'NONE',  ( 4.312004677471073855, -58.95452850542925205, 3.009306630940844496 ) ) ;
#1104=CARTESIAN_POINT ( 'NONE',  ( 2.179377348189628361, -66.64547149457072805, 7.030887037049939003 ) ) ;
#1108=CARTESIAN_POINT ( 'NONE',  ( -4.725907263620353405, -74.59547149457074511, -1.635492904037597617 ) ) ;
#1109=CARTESIAN_POINT ( 'NONE',  ( -5.257311121191324155, -68.74547149457072237, -0.09995255151718371311 ) ) ;
#1110=CARTESIAN_POINT ( 'NONE',  ( 1.529537955723688336, -59.85452850542924352, -5.030887037049978971 ) ) ;
#1113=CARTESIAN_POINT ( 'NONE',  ( 4.784657899331208775, -68.10452850542925773, 1.454677039711774533 ) ) ;
#1114=CARTESIAN_POINT ( 'NONE',  ( 4.312004677471010794, -61.54547149457073374, -3.009306630940933314 ) ) ;
#1121=CARTESIAN_POINT ( 'NONE',  ( -1.719659006605371632, -81.15452850542922647, -4.969112962950016588 ) ) ;
#1123=CARTESIAN_POINT ( 'NONE',  ( 3.015831842038149802, -85.69547149457073942, -3.989209796945492048 ) ) ;
#1124=CARTESIAN_POINT ( 'NONE',  ( 1.719659006605388507, -58.65452850542925489, 4.969112962950015699 ) ) ;
#1125=CARTESIAN_POINT ( 'NONE',  ( 2.610703060766946138, -85.54547149457074795, -1.773238653441125523 ) ) ;
#1126=CARTESIAN_POINT ( 'NONE',  ( -2.369498399071206407, -78.15452850542924068, -6.969112962950009482 ) ) ;
#1127=CARTESIAN_POINT ( 'NONE',  ( 3.015831842038150246, -88.69547149457073942, -3.989209796945492048 ) ) ;
#1128=CARTESIAN_POINT ( 'NONE',  ( -2.862020680886495416, -70.20452850542925205, 4.100960146804039752 ) ) ;
#1129=CARTESIAN_POINT ( 'NONE',  ( -4.037591185471423039, -76.20452850542925205, 5.718994135553947977 ) ) ;
#1134=CARTESIAN_POINT ( 'NONE',  ( -2.882544866740855749, -92.89547149457074227, 0.8366430509619596778 ) ) ;
#1139=VERTEX_POINT ( 'NONE', #7940 ) ;
#1140=CARTESIAN_POINT ( 'NONE',  ( -1.529537955723668130, -94.35452850542924352, 5.030887037049979860 ) ) ;
#1141=CARTESIAN_POINT ( 'NONE',  ( 1.840261337453269919, -67.80452850542926058, 2.371175808195547852 ) ) ;
#1142=CARTESIAN_POINT ( 'NONE',  ( -0.09506052544083808120, -93.00452850542926342, -4.999999999999997335 ) ) ;
#1143=CARTESIAN_POINT ( 'NONE',  ( 2.369498399071077177, -73.84547149457073090, -6.969112962950057444 ) ) ;
#1144=CARTESIAN_POINT ( 'NONE',  ( 5.257311121191342806, -92.25452850542922079, -0.09995255151729465215 ) ) ;
#1145=CARTESIAN_POINT ( 'NONE',  ( 3.015831842038150246, -88.69547149457073942, -3.989209796945492048 ) ) ;
#1146=CARTESIAN_POINT ( 'NONE',  ( 2.882544866740898382, -89.10452850542925773, 0.8366430509618999478 ) ) ;
#1149=PRESENTATION_STYLE_ASSIGNMENT (( #3841 ) ) ;
#1150=CARTESIAN_POINT ( 'NONE',  ( -4.194503406049320482, -61.05452850542923926, 3.171033256558100533 ) ) ;
#1151=CARTESIAN_POINT ( 'NONE',  ( -6.013306294175061240, -69.04547149457074795, 4.245374608440741326 ) ) ;
#1154=CARTESIAN_POINT ( 'NONE',  ( 4.597760815568308068, -96.99999999999982947, 2.447692062181759720 ) ) ;
#1155=CARTESIAN_POINT ( 'NONE',  ( -1.719659006605267493, -63.34547149457074511, 4.969112962950051227 ) ) ;
#1156=CARTESIAN_POINT ( 'NONE',  ( 7.360235569667880284, -94.24547149457075079, 0.09995255151716216091 ) ) ;
#1157=CARTESIAN_POINT ( 'NONE',  ( -1.686450176301564019, -91.20452850542925205, 2.482926158054133303 ) ) ;
#1160=CARTESIAN_POINT ( 'NONE',  ( 5.257311121191341918, -71.25452850542923500, -0.09995255151729465215 ) ) ;
#1161=CARTESIAN_POINT ( 'NONE',  ( -0.09506052544071151578, -96.49547149457075079, 6.999999999999997335 ) ) ;
#1167=CARTESIAN_POINT ( 'NONE',  ( -5.257311121191324155, -72.75452850542924921, 0.09995255151729526277 ) ) ;
#1168=CARTESIAN_POINT ( 'NONE',  ( -4.784657899331157260, -86.89547149457074227, 1.454677039711874675 ) ) ;
#1169=CARTESIAN_POINT ( 'NONE',  ( -2.862020680886496748, -58.20452850542925916, 4.100960146804039752 ) ) ;
#1170=CARTESIAN_POINT ( 'NONE',  ( -0.8796985632579434888, -71.14547149457074227, -3.030887037049952326 ) ) ;
#1171=CARTESIAN_POINT ( 'NONE',  ( 4.191402346623197772, -76.80452850542926058, 5.607243785695311900 ) ) ;
#1172=CARTESIAN_POINT ( 'NONE',  ( -4.784657899331156372, -92.89547149457075648, 1.454677039711874675 ) ) ;
#1173=CARTESIAN_POINT ( 'NONE',  ( -1.719659006605374074, -63.15452850542925489, -4.969112962950016588 ) ) ;
#1174=CARTESIAN_POINT ( 'NONE',  ( 2.179377348189482699, -80.85452850542925773, -7.030887037049986077 ) ) ;
#1175=CARTESIAN_POINT ( 'NONE',  ( 1.686450176301636850, -84.79547149457074795, 2.482926158054096000 ) ) ;
#1178=CARTESIAN_POINT ( 'NONE',  ( -4.312004677470996583, -60.04547149457074084, 3.009306630940933314 ) ) ;
#1180=CARTESIAN_POINT ( 'NONE',  ( -4.312004677471055203, -93.45452850542925205, -3.009306630940843608 ) ) ;
#1181=CARTESIAN_POINT ( 'NONE',  ( -2.493201789345288688, -95.44547149457075363, -1.934965279058240561 ) ) ;
#1183=CARTESIAN_POINT ( 'NONE',  ( -6.013306294175153610, -60.45452850542925916, -4.245374608440613429 ) ) ;
#1184=CARTESIAN_POINT ( 'NONE',  ( -5.895805022753479285, -68.44547149457073942, -4.407101234057782868 ) ) ;
#1185=CARTESIAN_POINT ( 'NONE',  ( 4.725907263620373833, -85.09547149457074511, 1.635492904037598283 ) ) ;
#1186=CARTESIAN_POINT ( 'NONE',  ( -2.882544866740877954, -72.60452850542924352, -0.8366430509618996147 ) ) ;
#1190=CARTESIAN_POINT ( 'NONE',  ( 4.194503406049334693, -62.55452850542925347, -3.171033256558100089 ) ) ;
#1191=CARTESIAN_POINT ( 'NONE',  ( -4.037591185471545607, -68.29547149457073374, -5.718994135553860936 ) ) ;
#1193=CARTESIAN_POINT ( 'NONE',  ( -1.529537955723777820, -68.14547149457074227, -5.030887037049945221 ) ) ;
#1194=CARTESIAN_POINT ( 'NONE',  ( -4.191402346623055664, -96.19547149457075363, 5.607243785695398941 ) ) ;
#1195=CARTESIAN_POINT ( 'NONE',  ( 3.154386672714811102, -95.25452850542926342, -0.09995255151727241993 ) ) ;
#1198=CARTESIAN_POINT ( 'NONE',  ( 1.529537955723689224, -71.85452850542925773, -5.030887037049978971 ) ) ;
#1199=CARTESIAN_POINT ( 'NONE',  ( -6.686770931921456551, -95.89547149457075648, 2.072711028461789784 ) ) ;
#1209=CARTESIAN_POINT ( 'NONE',  ( 2.862020680886514956, -80.70452850542925205, -4.100960146804039752 ) ) ;
#1210=CARTESIAN_POINT ( 'NONE',  ( -3.015831842038127597, -87.19547149457073942, 3.989209796945492048 ) ) ;
#1211=CARTESIAN_POINT ( 'NONE',  ( -5.257311121191325931, -57.75452850542924921, 0.09995255151729529053 ) ) ;
#1212=CARTESIAN_POINT ( 'NONE',  ( 3.154386672714808437, -70.24547149457075079, 0.09995255151720662534 ) ) ;
#1213=CARTESIAN_POINT ( 'NONE',  ( 7.360235569667878508, -83.25452850542926342, -0.09995255151731691212 ) ) ;
#1214=CARTESIAN_POINT ( 'NONE',  ( 1.529537955723796472, -87.64547149457071384, 5.030887037049945221 ) ) ;
#1215=CARTESIAN_POINT ( 'NONE',  ( 3.015831842038231958, -61.80452850542926058, 3.989209796945429432 ) ) ;
#1217=CARTESIAN_POINT ( 'NONE',  ( 7.360235569667877620, -77.25452850542924921, -0.09995255151731691212 ) ) ;
#1218=CARTESIAN_POINT ( 'NONE',  ( -2.493201789345289132, -92.44547149457073942, -1.934965279058240561 ) ) ;
#1223=CARTESIAN_POINT ( 'NONE',  ( 5.257311121191343695, -92.25452850542924921, -0.09995255151729466603 ) ) ;
#1224=CARTESIAN_POINT ( 'NONE',  ( -0.09506052544082083111, -63.00452850542925631, -2.999999999999997780 ) ) ;
#1225=CARTESIAN_POINT ( 'NONE',  ( 4.191402346623195996, -58.80452850542926058, 5.607243785695311900 ) ) ;
#1226=CARTESIAN_POINT ( 'NONE',  ( 4.191402346623077868, -73.69547149457073942, -5.607243785695398941 ) ) ;
#1227=CARTESIAN_POINT ( 'NONE',  ( -1.719659006605263940, -90.34547149457074511, 4.969112962950051227 ) ) ;
#1228=CARTESIAN_POINT ( 'NONE',  ( -1.686450176301565351, -79.20452850542925205, 2.482926158054133303 ) ) ;
#1230=CARTESIAN_POINT ( 'NONE',  ( -2.823794231030019475, -87.90452850542926910, 1.017458915287783316 ) ) ;
#1231=CARTESIAN_POINT ( 'NONE',  ( 6.628020296210686446, -64.09547149457071669, 2.253526892787472757 ) ) ;
#1233=CARTESIAN_POINT ( 'NONE',  ( 1.529537955723794251, -63.64547149457074227, 5.030887037049945221 ) ) ;
#1234=CARTESIAN_POINT ( 'NONE',  ( 4.784657899331175912, -61.39547149457074227, -1.454677039711874009 ) ) ;
#1235=CARTESIAN_POINT ( 'NONE',  ( -0.8796985632578772085, -94.35452850542925773, 3.030887037049973198 ) ) ;
#1237=CARTESIAN_POINT ( 'NONE',  ( -4.784657899331190123, -72.60452850542925773, -1.454677039711773867 ) ) ;
#1239=CARTESIAN_POINT ( 'NONE',  ( 0.09506052544073614885, -91.99547149457075079, -6.999999999999997335 ) ) ;
#1246=CARTESIAN_POINT ( 'NONE',  ( -1.529537955723670128, -79.35452850542925773, 5.030887037049979860 ) ) ;
#1247=CARTESIAN_POINT ( 'NONE',  ( 4.725907263620374721, -88.09547149457074511, 1.635492904037598283 ) ) ;
#1249=CARTESIAN_POINT ( 'NONE',  ( -2.493201789345291353, -74.44547149457072521, -1.934965279058240561 ) ) ;
#1250=CARTESIAN_POINT ( 'NONE',  ( 2.179377348189481811, -74.85452850542925773, -7.030887037049986077 ) ) ;
#1251=CARTESIAN_POINT ( 'NONE',  ( 0.09506052544075639654, -85.99547149457075079, -4.999999999999997335 ) ) ;
#1254=CARTESIAN_POINT ( 'NONE',  ( -4.191402346623179120, -75.30452850542926058, -5.607243785695311900 ) ) ;
#1255=CARTESIAN_POINT ( 'NONE',  ( -3.154386672714788453, -86.74547149457075079, -0.09995255151720625064 ) ) ;
#1259=CARTESIAN_POINT ( 'NONE',  ( -1.719659006605267937, -60.34547149457073800, 4.969112962950051227 ) ) ;
#1261=CARTESIAN_POINT ( 'NONE',  ( 5.257311121191342806, -80.25452850542924921, -0.09995255151729466603 ) ) ;
#1262=CARTESIAN_POINT ( 'NONE',  ( -0.09506052544082159439, -57.00452850542925631, -2.999999999999997780 ) ) ;
#1263=CARTESIAN_POINT ( 'NONE',  ( 4.312004677471078296, -91.95452850542925205, 3.009306630940844496 ) ) ;
#1266=CARTESIAN_POINT ( 'NONE',  ( -4.191402346623058328, -72.19547149457073942, 5.607243785695398941 ) ) ;
#1267=CARTESIAN_POINT ( 'NONE',  ( 1.529537955723796916, -87.64547149457072805, 5.030887037049945221 ) ) ;
#1268=CARTESIAN_POINT ( 'NONE',  ( -2.882544866740877509, -75.60452850542924352, -0.8366430509618996147 ) ) ;
#1270=B_SPLINE_CURVE_WITH_KNOTS ( 'NONE', 3,
 ( #1416, #1972, #4441, #7829, #2057, #6429, #3274, #6553, #7149, #2514, #6392, #5078, #3149, #3231, #16, #62, #608, #8285, #1891, #5745, #2645, #8326, #7783, #2559, #5120, #2598, #4523, #7103, #5922, #3479, #8038, #7873 ),
 .UNSPECIFIED., .F., .F.,
 ( 4, 2, 2, 2, 2, 2, 2, 2, 2, 2, 2, 2, 2, 2, 2, 4 ),
 ( 0.01224977136307512857, 0.01231928787409572804, 0.01238880438511632751, 0.01252783740715752644, 0.01280590345123992606, 0.01336203553940472182, 0.01447429971573431680, 0.01503043180389911429, 0.01558656389206391005, 0.01669882806839350503, 0.01725496015655830079, 0.01781109224472309654, 0.01836722433288789230, 0.01892335642105269153, 0.02003562059738228651, 0.02114788477371187803 ),
 .UNSPECIFIED. ) ;
#1271=FACE_OUTER_BOUND ( 'NONE', #6683, .T. ) ;
#1272=SURFACE_STYLE_FILL_AREA ( #3170 ) ;
#1273=CARTESIAN_POINT ( 'NONE',  ( -2.493201789345250052, -91.05452850542926058, 1.934965279058294518 ) ) ;
#1274=CARTESIAN_POINT ( 'NONE',  ( 7.360235569667875843, -61.24547149457073658, 0.09995255151716216091 ) ) ;
#1276=CARTESIAN_POINT ( 'NONE',  ( 0.09506052544075337118, -61.99547149457074369, -4.999999999999997335 ) ) ;
#1277=CARTESIAN_POINT ( 'NONE',  ( 5.895805022753498825, -96.94547149457073942, 4.407101234057782868 ) ) ;
#1280=CARTESIAN_POINT ( 'NONE',  ( 0.09506052544085971667, -73.50452850542924921, 4.999999999999997335 ) ) ;
#1281=CARTESIAN_POINT ( 'NONE',  ( 6.686770931921479644, -88.39547149457074227, -2.072711028461788896 ) ) ;
#1287=CARTESIAN_POINT ( 'NONE',  ( -4.784657899331190123, -78.60452850542925773, -1.454677039711773867 ) ) ;
#1288=CARTESIAN_POINT ( 'NONE',  ( -4.312004677470992142, -81.04547149457070532, 3.009306630940933758 ) ) ;
#1291=CARTESIAN_POINT ( 'NONE',  ( -0.09506052544075743738, -69.49547149457075079, 2.999999999999997780 ) ) ;
#1292=CARTESIAN_POINT ( 'NONE',  ( 5.895805022753404678, -65.55452850542926058, -4.407101234057908989 ) ) ;
#1293=CARTESIAN_POINT ( 'NONE',  ( 1.719659006605286367, -82.84547149457074511, -4.969112962950050338 ) ) ;
#1295=CARTESIAN_POINT ( 'NONE',  ( 1.719659006605392504, -91.65452850542925489, 4.969112962950016588 ) ) ;
#1296=CARTESIAN_POINT ( 'NONE',  ( 2.369498399071224615, -70.65452850542925489, 6.969112962950009482 ) ) ;
#1297=CARTESIAN_POINT ( 'NONE',  ( 2.823794231030061663, -91.09547149457074511, 1.017458915287723809 ) ) ;
#1301=CARTESIAN_POINT ( 'NONE',  ( 4.784657899331211439, -86.10452850542925773, 1.454677039711774533 ) ) ;
#1303=CARTESIAN_POINT ( 'NONE',  ( 1.719659006605390950, -76.65452850542924068, 4.969112962950015699 ) ) ;
#1304=CARTESIAN_POINT ( 'NONE',  ( -2.882544866740879286, -60.60452850542926484, -0.8366430509618996147 ) ) ;
#1305=CARTESIAN_POINT ( 'NONE',  ( 1.719659006605391616, -82.65452850542925489, 4.969112962950016588 ) ) ;
#1306=CARTESIAN_POINT ( 'NONE',  ( 0.09506052544073274879, -64.99547149457075079, -6.999999999999997335 ) ) ;
#1307=CARTESIAN_POINT ( 'NONE',  ( -1.719659006605264606, -84.34547149457073090, 4.969112962950051227 ) ) ;
#1308=CARTESIAN_POINT ( 'NONE',  ( 0.8796985632578985248, -71.85452850542924352, -3.030887037049972310 ) ) ;
#1310=PLANE ( 'NONE',  #6178 ) ;
#1312=CARTESIAN_POINT ( 'NONE',  ( 1.069819614139558839, -91.65452850542924068, 2.969112962950023249 ) ) ;
#1313=CARTESIAN_POINT ( 'NONE',  ( -2.179377348189613262, -59.14547149457074227, -7.030887037049939003 ) ) ;
#1315=CARTESIAN_POINT ( 'NONE',  ( -3.015831842038215527, -72.30452850542926058, -3.989209796945429432 ) ) ;
#1316=CARTESIAN_POINT ( 'NONE',  ( 4.725907263620371168, -61.09547149457074511, 1.635492904037598283 ) ) ;
#1319=CARTESIAN_POINT ( 'NONE',  ( 4.312004677471073855, -58.95452850542925205, 3.009306630940844496 ) ) ;
#1321=CARTESIAN_POINT ( 'NONE',  ( 2.179377348189630581, -87.64547149457075648, 7.030887037049939003 ) ) ;
#1323=CARTESIAN_POINT ( 'NONE',  ( 3.015831842038233734, -73.80452850542926058, 3.989209796945429432 ) ) ;
#1327=CARTESIAN_POINT ( 'NONE',  ( 4.725907263620373833, -82.09547149457074511, 1.635492904037598283 ) ) ;
#1330=CARTESIAN_POINT ( 'NONE',  ( 1.840261337453219959, -73.69547149457073942, -2.371175808195584267 ) ) ;
#1332=CARTESIAN_POINT ( 'NONE',  ( 7.360235569667877620, -68.25452850542924921, -0.09995255151731691212 ) ) ;
#1334=CARTESIAN_POINT ( 'NONE',  ( 3.015831842038149802, -82.69547149457073942, -3.989209796945492048 ) ) ;
#1335=CARTESIAN_POINT ( 'NONE',  ( 4.784657899331207886, -59.10452850542925773, 1.454677039711774533 ) ) ;
#1337=CARTESIAN_POINT ( 'NONE',  ( 7.360235569667877620, -68.25452850542924921, -0.09995255151731691212 ) ) ;
#1340=CARTESIAN_POINT ( 'NONE',  ( -1.840261337453199975, -81.19547149457073942, 2.371175808195584267 ) ) ;
#1343=CARTESIAN_POINT ( 'NONE',  ( 1.719659006605392504, -94.65452850542921226, 4.969112962950016588 ) ) ;
#1344=CARTESIAN_POINT ( 'NONE',  ( 4.194503406049338246, -83.55452850542921794, -3.171033256558100089 ) ) ;
#1346=CARTESIAN_POINT ( 'NONE',  ( 4.312004677471078296, -82.95452850542925205, 3.009306630940844052 ) ) ;
#1347=CARTESIAN_POINT ( 'NONE',  ( 2.882544866740894385, -59.10452850542926484, 0.8366430509618999478 ) ) ;
#1349=CARTESIAN_POINT ( 'NONE',  ( -4.725907263620320542, -84.90452850542925489, 1.635492904037698647 ) ) ;
#1350=CARTESIAN_POINT ( 'NONE',  ( 4.037591185471560706, -63.79547149457074084, 5.718994135553860936 ) ) ;
#1351=CARTESIAN_POINT ( 'NONE',  ( -4.194503406049383543, -80.44547149457073942, -3.171033256558012159 ) ) ;
#1352=CARTESIAN_POINT ( 'NONE',  ( 2.823794231030039015, -65.40452850542925489, -1.017458915287783316 ) ) ;
#1356=CARTESIAN_POINT ( 'NONE',  ( 2.823794231030042567, -92.40452850542925489, -1.017458915287783316 ) ) ;
#1357=CARTESIAN_POINT ( 'NONE',  ( 2.179377348189627472, -60.64547149457074227, 7.030887037049939003 ) ) ;
#1360=CARTESIAN_POINT ( 'NONE',  ( -5.257311121191323267, -81.75452850542926342, 0.09995255151729526277 ) ) ;
#1361=CARTESIAN_POINT ( 'NONE',  ( 4.191402346623079644, -85.69547149457073942, -5.607243785695398941 ) ) ;
#1364=CARTESIAN_POINT ( 'NONE',  ( 4.194503406049334693, -59.55452850542926058, -3.171033256558100089 ) ) ;
#1365=CARTESIAN_POINT ( 'NONE',  ( -7.360235569667858080, -86.74547149457075079, -0.09995255151716124498 ) ) ;
#1368=CARTESIAN_POINT ( 'NONE',  ( 4.194503406049337357, -74.55452850542923215, -3.171033256558100089 ) ) ;
#1371=CARTESIAN_POINT ( 'NONE',  ( 1.719659006605286145, -79.84547149457071669, -4.969112962950050338 ) ) ;
#1373=CARTESIAN_POINT ( 'NONE',  ( 0.09506052544075790922, -97.99547149457075079, -4.999999999999997335 ) ) ;
#1374=CARTESIAN_POINT ( 'NONE',  ( -0.09506052544086177059, -72.00452850542926342, -6.999999999999997335 ) ) ;
#1376=CARTESIAN_POINT ( 'NONE',  ( 3.015831842038148913, -76.69547149457075363, -3.989209796945492048 ) ) ;
#1377=CARTESIAN_POINT ( 'NONE',  ( 4.302742873392585210, -96.99999999999947420, 2.548615363087012753 ) ) ;
#1378=CARTESIAN_POINT ( 'NONE',  ( -3.015831842038213750, -87.30452850542926058, -3.989209796945429432 ) ) ;
#1379=CARTESIAN_POINT ( 'NONE',  ( -4.191402346623180009, -66.30452850542926058, -5.607243785695311900 ) ) ;
#1380=CARTESIAN_POINT ( 'NONE',  ( -1.069819614139474462, -78.34547149457074511, 2.969112962950044121 ) ) ;
#1384=CARTESIAN_POINT ( 'NONE',  ( 3.015831842038235067, -85.80452850542926058, 3.989209796945429432 ) ) ;
#1386=CARTESIAN_POINT ( 'NONE',  ( 4.784657899331210551, -83.10452850542927195, 1.454677039711774533 ) ) ;
#1387=CARTESIAN_POINT ( 'NONE',  ( 1.840261337453221957, -91.69547149457075363, -2.371175808195584267 ) ) ;
#1389=CARTESIAN_POINT ( 'NONE',  ( 4.312004677471076519, -82.95452850542925205, 3.009306630940844496 ) ) ;
#1390=CARTESIAN_POINT ( 'NONE',  ( 7.360235569667875843, -61.24547149457073658, 0.09995255151716216091 ) ) ;
#1391=CARTESIAN_POINT ( 'NONE',  ( 0.09506052544083769262, -67.50452850542926342, 2.999999999999997780 ) ) ;
#1395=CARTESIAN_POINT ( 'NONE',  ( -0.09506052544081818045, -84.00452850542926342, -2.999999999999997780 ) ) ;
#1397=CARTESIAN_POINT ( 'NONE',  ( -4.037591185471420374, -94.20452850542928047, 5.718994135553947977 ) ) ;
#1400=CARTESIAN_POINT ( 'NONE',  ( 4.194503406049337357, -77.55452850542926058, -3.171033256558100089 ) ) ;
#1401=CARTESIAN_POINT ( 'NONE',  ( -5.895805022753476621, -86.44547149457073942, -4.407101234057782868 ) ) ;
#1404=CARTESIAN_POINT ( 'NONE',  ( 0.8796985632579609193, -69.64547149457072805, 3.030887037049952326 ) ) ;
#1406=CARTESIAN_POINT ( 'NONE',  ( 1.719659006605388507, -61.65452850542923358, 4.969112962950016588 ) ) ;
#1407=CARTESIAN_POINT ( 'NONE',  ( 7.360235569667880284, -94.24547149457075079, 0.09995255151716216091 ) ) ;
#1409=( LENGTH_UNIT ( ) NAMED_UNIT ( * ) SI_UNIT ( .MILLI., .METRE. ) );
#1411=CARTESIAN_POINT ( 'NONE',  ( 3.015831842038233290, -70.80452850542926058, 3.989209796945429432 ) ) ;
#1415=CARTESIAN_POINT ( 'NONE',  ( -4.194503406049384431, -77.44547149457075363, -3.171033256558012159 ) ) ;
#1416=CARTESIAN_POINT ( 'NONE',  ( 4.302742873392585210, -96.99999999999947420, 2.548615363087012753 ) ) ;
#1417=CARTESIAN_POINT ( 'NONE',  ( 3.015831842038151578, -97.69547149457075363, -3.989209796945492048 ) ) ;
#1418=CARTESIAN_POINT ( 'NONE',  ( 2.369498399071224615, -70.65452850542925489, 6.969112962950009482 ) ) ;
#1420=CARTESIAN_POINT ( 'NONE',  ( 4.725907263620372945, -79.09547149457074511, 1.635492904037598283 ) ) ;
#1423=CARTESIAN_POINT ( 'NONE',  ( -3.015831842038213750, -84.30452850542926058, -3.989209796945429432 ) ) ;
#1424=CARTESIAN_POINT ( 'NONE',  ( -5.895805022753386915, -67.05452850542926058, 4.407101234057909878 ) ) ;
#1425=CARTESIAN_POINT ( 'NONE',  ( 0.8796985632579621406, -78.64547149457074227, 3.030887037049952326 ) ) ;
#1430=CARTESIAN_POINT ( 'NONE',  ( -4.194503406049315153, -91.05452850542923215, 3.171033256558100533 ) ) ;
#1432=CARTESIAN_POINT ( 'NONE',  ( -4.194503406049316929, -82.05452850542926058, 3.171033256558101865 ) ) ;
#1433=CARTESIAN_POINT ( 'NONE',  ( 0.09506052544077819855, -91.99547149457075079, -2.999999999999997780 ) ) ;
#1435=CARTESIAN_POINT ( 'NONE',  ( -4.725907263620320542, -81.90452850542925489, 1.635492904037698647 ) ) ;
#1436=CARTESIAN_POINT ( 'NONE',  ( -6.686770931921503625, -93.60452850542925773, -2.072711028461647675 ) ) ;
#1437=CARTESIAN_POINT ( 'NONE',  ( 2.610703060766982553, -67.95452850542925205, 1.773238653441072232 ) ) ;
#1440=CARTESIAN_POINT ( 'NONE',  ( -2.610703060766964345, -78.45452850542925205, -1.773238653441072232 ) ) ;
#1441=CARTESIAN_POINT ( 'NONE',  ( 7.360235569667880284, -89.25452850542926342, -0.09995255151731691212 ) ) ;
#1443=CARTESIAN_POINT ( 'NONE',  ( 5.895805022753496161, -87.94547149457073942, 4.407101234057782868 ) ) ;
#1446=CARTESIAN_POINT ( 'NONE',  ( 2.610703060766944361, -70.54547149457074795, -1.773238653441125523 ) ) ;
#1448=CARTESIAN_POINT ( 'NONE',  ( -4.725907263620322318, -66.90452850542925489, 1.635492904037698647 ) ) ;
#1449=CARTESIAN_POINT ( 'NONE',  ( -0.09506052544071380561, -78.49547149457075079, 6.999999999999997335 ) ) ;
#1452=CARTESIAN_POINT ( 'NONE',  ( 2.862020680886514512, -77.70452850542926626, -4.100960146804039752 ) ) ;
#1455=CARTESIAN_POINT ( 'NONE',  ( 2.862020680886599777, -81.79547149457073374, 4.100960146803977580 ) ) ;
#1457=CARTESIAN_POINT ( 'NONE',  ( 0.8796985632579601422, -63.64547149457072805, 3.030887037049952326 ) ) ;
#1458=CARTESIAN_POINT ( 'NONE',  ( 2.369498399071224615, -73.65452850542925489, 6.969112962950009482 ) ) ;
#1462=CARTESIAN_POINT ( 'NONE',  ( -2.862020680886493640, -82.20452850542925205, 4.100960146804039752 ) ) ;
#1463=CARTESIAN_POINT ( 'NONE',  ( -6.013306294175152722, -69.45452850542925205, -4.245374608440613429 ) ) ;
#1465=CARTESIAN_POINT ( 'NONE',  ( 2.882544866740877954, -82.39547149457074227, -0.8366430509619593447 ) ) ;
#1471=CARTESIAN_POINT ( 'NONE',  ( -4.725907263620319654, -90.90452850542926910, 1.635492904037698647 ) ) ;
#1473=CARTESIAN_POINT ( 'NONE',  ( -4.194503406049317817, -73.05452850542926058, 3.171033256558101865 ) ) ;
#1474=CARTESIAN_POINT ( 'NONE',  ( -0.09506052544075518917, -87.49547149457075079, 2.999999999999997780 ) ) ;
#1475=CARTESIAN_POINT ( 'NONE',  ( 4.725907263620341858, -86.40452850542926910, -1.635492904037697981 ) ) ;
#1477=CARTESIAN_POINT ( 'NONE',  ( 7.360235569667875843, -64.24547149457075079, 0.09995255151716216091 ) ) ;
#1479=CARTESIAN_POINT ( 'NONE',  ( 3.154386672714807549, -68.25452850542924921, -0.09995255151727241993 ) ) ;
#1483=CARTESIAN_POINT ( 'NONE',  ( -2.610703060766965233, -75.45452850542925205, -1.773238653441072232 ) ) ;
#1484=CARTESIAN_POINT ( 'NONE',  ( -6.013306294175149169, -93.45452850542926626, -4.245374608440613429 ) ) ;
#1485=CARTESIAN_POINT ( 'NONE',  ( -2.179377348189609265, -89.14547149457072805, -7.030887037049939003 ) ) ;
#1488=CARTESIAN_POINT ( 'NONE',  ( 1.686450176301634851, -66.79547149457073374, 2.482926158054096000 ) ) ;
#1491=CARTESIAN_POINT ( 'NONE',  ( 4.312004677471074743, -70.95452850542925205, 3.009306630940844496 ) ) ;
#1492=CARTESIAN_POINT ( 'NONE',  ( -6.013306294175058575, -81.04547149457074795, 4.245374608440741326 ) ) ;
#1495=CARTESIAN_POINT ( 'NONE',  ( -4.312004677471057867, -75.45452850542925205, -3.009306630940844052 ) ) ;
#1496=CARTESIAN_POINT ( 'NONE',  ( -4.481820730511953954E-14, -57.99999999999999289, -4.999999999999997335 ) ) ;
#1498=CARTESIAN_POINT ( 'NONE',  ( -5.257311121191324155, -68.74547149457072237, -0.09995255151718371311 ) ) ;
#1500=CARTESIAN_POINT ( 'NONE',  ( -1.719659006605263496, -96.34547149457074511, 4.969112962950051227 ) ) ;
#1501=CARTESIAN_POINT ( 'NONE',  ( 5.895805022753402902, -62.55452850542925347, -4.407101234057908989 ) ) ;
#1504=CARTESIAN_POINT ( 'NONE',  ( 4.725907263620341858, -86.40452850542926910, -1.635492904037697981 ) ) ;
#1505=CARTESIAN_POINT ( 'NONE',  ( 5.895805022753402902, -62.55452850542925347, -4.407101234057908989 ) ) ;
#1506=CARTESIAN_POINT ( 'NONE',  ( -3.154386672714789785, -77.74547149457073658, -0.09995255151720625064 ) ) ;
#1509=CARTESIAN_POINT ( 'NONE',  ( 5.257311121191342806, -92.25452850542922079, -0.09995255151729465215 ) ) ;
#1510=CARTESIAN_POINT ( 'NONE',  ( 4.312004677471076519, -79.95452850542922363, 3.009306630940844496 ) ) ;
#1512=CARTESIAN_POINT ( 'NONE',  ( 5.257311121191341030, -68.25452850542926342, -0.09995255151729466603 ) ) ;
#1513=CARTESIAN_POINT ( 'NONE',  ( -3.154386672714788453, -86.74547149457075079, -0.09995255151720625064 ) ) ;
#1515=CARTESIAN_POINT ( 'NONE',  ( -3.154386672714792006, -62.74547149457073658, -0.09995255151720625064 ) ) ;
#1516=CARTESIAN_POINT ( 'NONE',  ( -6.013306294175061240, -63.04547149457074084, 4.245374608440741326 ) ) ;
#1517=CARTESIAN_POINT ( 'NONE',  ( 1.840261337453268808, -61.80452850542926058, 2.371175808195547852 ) ) ;
#1523=CARTESIAN_POINT ( 'NONE',  ( 0.09506052544083919142, -79.50452850542926342, 2.999999999999997780 ) ) ;
#1524=CARTESIAN_POINT ( 'NONE',  ( 6.686770931921525829, -86.10452850542924352, 2.072711028461649008 ) ) ;
#1525=CARTESIAN_POINT ( 'NONE',  ( -2.369498399071056305, -84.34547149457075932, 6.969112962950058332 ) ) ;
#1528=CARTESIAN_POINT ( 'NONE',  ( -2.823794231030041235, -65.59547149457073090, -1.017458915287723364 ) ) ;
#1531=CARTESIAN_POINT ( 'NONE',  ( -1.719659006605373630, -66.15452850542926910, -4.969112962950016588 ) ) ;
#1532=CARTESIAN_POINT ( 'NONE',  ( -6.686770931921458327, -83.89547149457074227, 2.072711028461789784 ) ) ;
#1535=CARTESIAN_POINT ( 'NONE',  ( 1.719659006605389617, -67.65452850542925489, 4.969112962950016588 ) ) ;
#1540=CARTESIAN_POINT ( 'NONE',  ( -4.312004677470993919, -69.04547149457071953, 3.009306630940933758 ) ) ;
#1542=CARTESIAN_POINT ( 'NONE',  ( 0.09506052544077440991, -61.99547149457073658, -2.999999999999997780 ) ) ;
#1543=CARTESIAN_POINT ( 'NONE',  ( -0.09506052544086329714, -60.00452850542925631, -6.999999999999997335 ) ) ;
#1547=CARTESIAN_POINT ( 'NONE',  ( -3.015831842038213750, -90.30452850542926058, -3.989209796945429432 ) ) ;
#1552=CARTESIAN_POINT ( 'NONE',  ( 1.719659006605392504, -91.65452850542925489, 4.969112962950016588 ) ) ;
#1553=CARTESIAN_POINT ( 'NONE',  ( 3.015831842038234623, -82.80452850542926058, 3.989209796945429432 ) ) ;
#1555=CARTESIAN_POINT ( 'NONE',  ( -0.09506052544084034328, -75.00452850542924921, -4.999999999999997335 ) ) ;
#1556=CARTESIAN_POINT ( 'NONE',  ( 2.882544866740878842, -88.39547149457074227, -0.8366430509619593447 ) ) ;
#1557=CARTESIAN_POINT ( 'NONE',  ( 1.719659006605287477, -94.84547149457074511, -4.969112962950050338 ) ) ;
#1558=CARTESIAN_POINT ( 'NONE',  ( -3.015831842038214194, -81.30452850542926058, -3.989209796945429432 ) ) ;
#1559=CARTESIAN_POINT ( 'NONE',  ( 4.191402346623198660, -88.80452850542926058, 5.607243785695311900 ) ) ;
#1560=CARTESIAN_POINT ( 'NONE',  ( -0.09506052544082159439, -57.00452850542925631, -2.999999999999997780 ) ) ;
#1564=CARTESIAN_POINT ( 'NONE',  ( -1.686450176301565351, -79.20452850542925205, 2.482926158054133303 ) ) ;
#1565=CARTESIAN_POINT ( 'NONE',  ( -0.09506052544085952238, -90.00452850542926342, -6.999999999999997335 ) ) ;
#1566=CARTESIAN_POINT ( 'NONE',  ( -4.037591185471543831, -83.29547149457074795, -5.718994135553860936 ) ) ;
#1568=CARTESIAN_POINT ( 'NONE',  ( -0.09506052544073276267, -96.49547149457075079, 4.999999999999997335 ) ) ;
#1569=CARTESIAN_POINT ( 'NONE',  ( -1.840261337453200863, -72.19547149457073942, 2.371175808195584267 ) ) ;
#1575=CARTESIAN_POINT ( 'NONE',  ( -4.194503406049319594, -70.05452850542923215, 3.171033256558100533 ) ) ;
#1576=CARTESIAN_POINT ( 'NONE',  ( -6.628020296210667794, -77.59547149457073090, -2.253526892787471869 ) ) ;
#1578=CARTESIAN_POINT ( 'NONE',  ( 5.257311121191341030, -79.24547149457073658, 0.09995255151718437925 ) ) ;
#1579=CARTESIAN_POINT ( 'NONE',  ( -2.862020680886580681, -74.29547149457074795, -4.100960146803977580 ) ) ;
#1580=CARTESIAN_POINT ( 'NONE',  ( 1.719659006605389173, -64.65452850542925489, 4.969112962950016588 ) ) ;
#1583=CARTESIAN_POINT ( 'NONE',  ( -4.725907263620353405, -74.59547149457074511, -1.635492904037597617 ) ) ;
#1586=CARTESIAN_POINT ( 'NONE',  ( -5.895805022753386915, -58.05452850542925347, 4.407101234057909878 ) ) ;
#1589=ADVANCED_FACE ( 'NONE', ( #1057 ), #4779, .T. ) ;
#1590=VERTEX_POINT ( 'NONE', #1377 ) ;
#1592=CARTESIAN_POINT ( 'NONE',  ( 5.257311121191342806, -89.25452850542924921, -0.09995255151729465215 ) ) ;
#1593=CARTESIAN_POINT ( 'NONE',  ( -4.725907263620320542, -81.90452850542925489, 1.635492904037698647 ) ) ;
#1595=CARTESIAN_POINT ( 'NONE',  ( -4.725907263620322318, -69.90452850542925489, 1.635492904037698647 ) ) ;
#1596=CARTESIAN_POINT ( 'NONE',  ( -0.8796985632579421566, -83.14547149457072805, -3.030887037049952326 ) ) ;
#1597=CARTESIAN_POINT ( 'NONE',  ( -3.015831842038126709, -93.19547149457075363, 3.989209796945492048 ) ) ;
#1598=CARTESIAN_POINT ( 'NONE',  ( 5.257311121191341918, -77.25452850542926342, -0.09995255151729465215 ) ) ;
#1599=CARTESIAN_POINT ( 'NONE',  ( 5.895805022753407343, -89.55452850542926058, -4.407101234057908989 ) ) ;
#1600=CARTESIAN_POINT ( 'NONE',  ( -3.154386672714792006, -57.75452850542924921, 0.09995255151727280851 ) ) ;
#1606=CARTESIAN_POINT ( 'NONE',  ( 2.493201789345270480, -65.55452850542926058, -1.934965279058294518 ) ) ;
#1607=CARTESIAN_POINT ( 'NONE',  ( -6.686770931921503625, -90.60452850542925773, -2.072711028461647675 ) ) ;
#1611=CARTESIAN_POINT ( 'NONE',  ( 4.191402346623078756, -76.69547149457073942, -5.607243785695398941 ) ) ;
#1615=CARTESIAN_POINT ( 'NONE',  ( -0.8796985632578778747, -88.35452850542924352, 3.030887037049973198 ) ) ;
#1619=CARTESIAN_POINT ( 'NONE',  ( 4.312004677471074743, -67.95452850542922363, 3.009306630940844496 ) ) ;
#1620=CARTESIAN_POINT ( 'NONE',  ( 4.191402346623078756, -79.69547149457075363, -5.607243785695398941 ) ) ;
#1621=( NAMED_UNIT ( * ) SI_UNIT ( $, .STERADIAN. ) SOLID_ANGLE_UNIT ( ) );
#1624=CARTESIAN_POINT ( 'NONE',  ( 1.529537955723795140, -72.64547149457074227, 5.030887037049945221 ) ) ;
#1625=CARTESIAN_POINT ( 'NONE',  ( 5.257311121191341918, -73.24547149457072237, 0.09995255151718437925 ) ) ;
#1626=CARTESIAN_POINT ( 'NONE',  ( 1.529537955723689002, -65.85452850542924352, -5.030887037049978971 ) ) ;
#1629=CARTESIAN_POINT ( 'NONE',  ( 4.194503406049401306, -72.94547149457073942, 3.171033256558012159 ) ) ;
#1631=CARTESIAN_POINT ( 'NONE',  ( -0.09506052544086367184, -57.00452850542925631, -6.999999999999997335 ) ) ;
#1636=CARTESIAN_POINT ( 'NONE',  ( 0.09506052544086197875, -91.50452850542924921, 4.999999999999997335 ) ) ;
#1637=CARTESIAN_POINT ( 'NONE',  ( -0.09506052544084034328, -75.00452850542924921, -4.999999999999997335 ) ) ;
#1639=CARTESIAN_POINT ( 'NONE',  ( 4.312004677471075631, -67.95452850542923784, 3.009306630940844052 ) ) ;
#1640=CARTESIAN_POINT ( 'NONE',  ( -1.686450176301616644, -80.29547149457074795, -2.482926158054096000 ) ) ;
#1641=CARTESIAN_POINT ( 'NONE',  ( -1.719659006605263940, -93.34547149457071669, 4.969112962950051227 ) ) ;
#1642=CARTESIAN_POINT ( 'NONE',  ( 4.312004677471074743, -67.95452850542922363, 3.009306630940844496 ) ) ;
#1643=CARTESIAN_POINT ( 'NONE',  ( -2.369498399071205963, -87.15452850542926910, -6.969112962950009482 ) ) ;
#1644=CARTESIAN_POINT ( 'NONE',  ( 1.840261337453268586, -58.80452850542926058, 2.371175808195547852 ) ) ;
#1651=CARTESIAN_POINT ( 'NONE',  ( 2.610703060766982553, -67.95452850542925205, 1.773238653441072232 ) ) ;
#1652=CARTESIAN_POINT ( 'NONE',  ( 7.360235569667877620, -76.24547149457073658, 0.09995255151716216091 ) ) ;
#1655=CARTESIAN_POINT ( 'NONE',  ( -0.09506052544081743105, -90.00452850542926342, -2.999999999999997780 ) ) ;
#1656=UNCERTAINTY_MEASURE_WITH_UNIT (LENGTH_MEASURE( 1.000000000000000082E-05 ), #4224, 'distance_accuracy_value', 'NONE');
#1661=CARTESIAN_POINT ( 'NONE',  ( 4.725907263620339194, -62.40452850542925489, -1.635492904037697981 ) ) ;
#1662=CARTESIAN_POINT ( 'NONE',  ( 4.037591185471562483, -75.79547149457074795, 5.718994135553860936 ) ) ;
#1664=CARTESIAN_POINT ( 'NONE',  ( -4.312004677470993919, -72.04547149457074795, 3.009306630940933314 ) ) ;
#1665=CARTESIAN_POINT ( 'NONE',  ( -3.015831842038129817, -69.19547149457073942, 3.989209796945492048 ) ) ;
#1666=CARTESIAN_POINT ( 'NONE',  ( -3.015831842038215971, -69.30452850542926058, -3.989209796945429432 ) ) ;
#1669=CARTESIAN_POINT ( 'NONE',  ( -0.09506052544073655131, -66.49547149457075079, 4.999999999999997335 ) ) ;
#1672=CARTESIAN_POINT ( 'NONE',  ( 4.725907263620342746, -95.40452850542925489, -1.635492904037697981 ) ) ;
#1675=DIRECTION ( 'NONE',  ( 0.9954714945707483498, 0.09506052544079827971, -1.047588144072330487E-14 ) ) ;
#1678=ORIENTED_EDGE ( 'NONE', *, *, #7828, .T. ) ;
#1680=CARTESIAN_POINT ( 'NONE',  ( 1.529537955723691001, -83.85452850542927195, -5.030887037049978971 ) ) ;
#1681=CARTESIAN_POINT ( 'NONE',  ( 4.784657899331209663, -74.10452850542925773, 1.454677039711774533 ) ) ;
#1682=CARTESIAN_POINT ( 'NONE',  ( -4.784657899331191899, -60.60452850542925773, -1.454677039711773867 ) ) ;
#1683=CARTESIAN_POINT ( 'NONE',  ( 0.09506052544077704669, -82.99547149457075079, -2.999999999999997780 ) ) ;
#1684=CARTESIAN_POINT ( 'NONE',  ( 0.09506052544075753452, -94.99547149457073658, -4.999999999999997335 ) ) ;
#1685=CARTESIAN_POINT ( 'NONE',  ( 1.719659006605389839, -70.65452850542926910, 4.969112962950016588 ) ) ;
#1686=CARTESIAN_POINT ( 'NONE',  ( 6.628020296210642037, -89.40452850542926910, -2.253526892787612645 ) ) ;
#1688=CARTESIAN_POINT ( 'NONE',  ( -3.154386672714787565, -95.74547149457073658, -0.09995255151720625064 ) ) ;
#1695=CARTESIAN_POINT ( 'NONE',  ( -1.069819614139538855, -72.15452850542922647, -2.969112962950023249 ) ) ;
#1696=CARTESIAN_POINT ( 'NONE',  ( -2.369498399071057193, -78.34547149457074511, 6.969112962950058332 ) ) ;
#1697=CARTESIAN_POINT ( 'NONE',  ( -0.09506052544083770650, -96.00452850542926342, -4.999999999999997335 ) ) ;
#1699=CARTESIAN_POINT ( 'NONE',  ( -4.194503406049381766, -92.44547149457075363, -3.171033256558012159 ) ) ;
#1700=CARTESIAN_POINT ( 'NONE',  ( 0.8796985632578994130, -80.85452850542925773, -3.030887037049972310 ) ) ;
#1704=CARTESIAN_POINT ( 'NONE',  ( 0.09506052544085781542, -58.50452850542925631, 4.999999999999997335 ) ) ;
#1705=CARTESIAN_POINT ( 'NONE',  ( -6.686770931921459216, -68.89547149457074227, 2.072711028461789784 ) ) ;
#1707=CARTESIAN_POINT ( 'NONE',  ( 0.09506052544075450916, -70.99547149457075079, -4.999999999999997335 ) ) ;
#1708=CARTESIAN_POINT ( 'NONE',  ( -4.725907263620355181, -65.59547149457073090, -1.635492904037597617 ) ) ;
#1709=CARTESIAN_POINT ( 'NONE',  ( -4.194503406049320482, -61.05452850542923926, 3.171033256558100533 ) ) ;
#1711=CARTESIAN_POINT ( 'NONE',  ( 1.529537955723793585, -60.64547149457074937, 5.030887037049945221 ) ) ;
#1713=CARTESIAN_POINT ( 'NONE',  ( -4.784657899331188347, -93.60452850542925773, -1.454677039711773867 ) ) ;
#1718=DIRECTION ( 'NONE',  ( -0.09506052544079829358, 0.9954714945707483498, 0.000000000000000000 ) ) ;
#1719=CARTESIAN_POINT ( 'NONE',  ( -3.015831842038213750, -87.30452850542926058, -3.989209796945429432 ) ) ;
#1720=CARTESIAN_POINT ( 'NONE',  ( 4.784657899331179465, -88.39547149457074227, -1.454677039711874009 ) ) ;
#1722=CARTESIAN_POINT ( 'NONE',  ( -4.784657899331191011, -66.60452850542924352, -1.454677039711773867 ) ) ;
#1723=CARTESIAN_POINT ( 'NONE',  ( -0.8796985632579424896, -80.14547149457074227, -3.030887037049952326 ) ) ;
#1724=CARTESIAN_POINT ( 'NONE',  ( -4.312004677470992142, -84.04547149457074795, 3.009306630940933758 ) ) ;
#1726=CARTESIAN_POINT ( 'NONE',  ( 1.719659006605389617, -67.65452850542925489, 4.969112962950016588 ) ) ;
#1727=CARTESIAN_POINT ( 'NONE',  ( 2.369498399071226835, -88.65452850542926910, 6.969112962950009482 ) ) ;
#1730=CARTESIAN_POINT ( 'NONE',  ( -2.493201789345254493, -58.05452850542925347, 1.934965279058294518 ) ) ;
#1734=CARTESIAN_POINT ( 'NONE',  ( -3.015831842038213306, -93.30452850542926058, -3.989209796945429432 ) ) ;
#1735=CARTESIAN_POINT ( 'NONE',  ( -2.493201789345253161, -67.05452850542926058, 1.934965279058294518 ) ) ;
#1736=CARTESIAN_POINT ( 'NONE',  ( -6.013306294175060351, -75.04547149457074795, 4.245374608440741326 ) ) ;
#1738=CARTESIAN_POINT ( 'NONE',  ( 3.015831842038150690, -91.69547149457073942, -3.989209796945492048 ) ) ;
#1739=CARTESIAN_POINT ( 'NONE',  ( 0.8796985632579000791, -86.85452850542924352, -3.030887037049972310 ) ) ;
#1743=CARTESIAN_POINT ( 'NONE',  ( -2.823794231030019031, -93.90452850542926910, 1.017458915287783316 ) ) ;
#1745=CARTESIAN_POINT ( 'NONE',  ( 7.360235569667877620, -73.24547149457075079, 0.09995255151716216091 ) ) ;
#1746=CARTESIAN_POINT ( 'NONE',  ( 2.484839419076748879, -97.00000000000000000, -5.444361870252323321 ) ) ;
#1747=CARTESIAN_POINT ( 'NONE',  ( 4.784657899331176800, -70.39547149457074227, -1.454677039711874009 ) ) ;
#1748=CARTESIAN_POINT ( 'NONE',  ( -4.312004677470993919, -69.04547149457071953, 3.009306630940933758 ) ) ;
#1749=CARTESIAN_POINT ( 'NONE',  ( 1.686450176301587334, -92.70452850542926626, -2.482926158054133303 ) ) ;
#1753=CARTESIAN_POINT ( 'NONE',  ( 1.529537955723689224, -68.85452850542921510, -5.030887037049978971 ) ) ;
#1755=CARTESIAN_POINT ( 'NONE',  ( -2.862020680886582014, -65.29547149457073374, -4.100960146803977580 ) ) ;
#1756=DIRECTION ( 'NONE',  ( 1.000000000000000000, 0.000000000000000000, 0.000000000000000000 ) ) ;
#1761=CARTESIAN_POINT ( 'NONE',  ( -4.194503406049316929, -76.05452850542926058, 3.171033256558100533 ) ) ;
#1762=CARTESIAN_POINT ( 'NONE',  ( 4.312004677471013459, -88.54547149457074795, -3.009306630940933314 ) ) ;
#1763=CARTESIAN_POINT ( 'NONE',  ( 4.725907263620339194, -59.40452850542926200, -1.635492904037697981 ) ) ;
#1764=CARTESIAN_POINT ( 'NONE',  ( -1.069819614139474462, -78.34547149457074511, 2.969112962950044121 ) ) ;
#1765=CARTESIAN_POINT ( 'NONE',  ( -4.037591185471422150, -79.20452850542925205, 5.718994135553947977 ) ) ;
#1766=CARTESIAN_POINT ( 'NONE',  ( -5.257311121191323267, -83.74547149457075079, -0.09995255151718371311 ) ) ;
#1767=CARTESIAN_POINT ( 'NONE',  ( 1.529537955723689224, -71.85452850542925773, -5.030887037049978971 ) ) ;
#1768=CARTESIAN_POINT ( 'NONE',  ( -4.037591185471422150, -79.20452850542925205, 5.718994135553947977 ) ) ;
#1769=CARTESIAN_POINT ( 'NONE',  ( 1.840261337453221513, -88.69547149457073942, -2.371175808195584267 ) ) ;
#1773=CARTESIAN_POINT ( 'NONE',  ( -1.719659006605370744, -90.15452850542925489, -4.969112962950015699 ) ) ;
#1774=CARTESIAN_POINT ( 'NONE',  ( -2.493201789345252717, -73.05452850542926058, 1.934965279058294518 ) ) ;
#1775=CARTESIAN_POINT ( 'NONE',  ( 4.312004677471079184, -94.95452850542926626, 3.009306630940844496 ) ) ;
#1777=CARTESIAN_POINT ( 'NONE',  ( 5.895805022753492608, -66.94547149457073942, 4.407101234057782868 ) ) ;
#1779=CARTESIAN_POINT ( 'NONE',  ( -4.194503406049382654, -83.44547149457072521, -3.171033256558012159 ) ) ;
#1780=CARTESIAN_POINT ( 'NONE',  ( 3.154386672714810658, -89.25452850542926342, -0.09995255151727241993 ) ) ;
#1784=CARTESIAN_POINT ( 'NONE',  ( 1.719659006605388285, -58.65452850542924068, 4.969112962950016588 ) ) ;
#1785=CARTESIAN_POINT ( 'NONE',  ( -5.895805022753479285, -68.44547149457073942, -4.407101234057782868 ) ) ;
#1787=CARTESIAN_POINT ( 'NONE',  ( 5.060638198296488532, -96.99999999999998579, 1.908797354467637541 ) ) ;
#1789=CARTESIAN_POINT ( 'NONE',  ( -2.862020680886582014, -65.29547149457073374, -4.100960146803977580 ) ) ;
#1790=CARTESIAN_POINT ( 'NONE',  ( -2.862020680886581570, -68.29547149457074795, -4.100960146803977580 ) ) ;
#1791=CARTESIAN_POINT ( 'NONE',  ( -2.823794231030019031, -90.90452850542926910, 1.017458915287783316 ) ) ;
#1795=CARTESIAN_POINT ( 'NONE',  ( 1.719659006605389839, -70.65452850542926910, 4.969112962950016588 ) ) ;
#1796=CARTESIAN_POINT ( 'NONE',  ( -4.194503406049384431, -59.44547149457074653, -3.171033256558012159 ) ) ;
#1803=CARTESIAN_POINT ( 'NONE',  ( 4.312004677471075631, -76.95452850542923784, 3.009306630940844496 ) ) ;
#1805=CARTESIAN_POINT ( 'NONE',  ( -5.257311121191322378, -89.74547149457070816, -0.09995255151718371311 ) ) ;
#1806=CARTESIAN_POINT ( 'NONE',  ( -4.784657899331191899, -63.60452850542925063, -1.454677039711773867 ) ) ;
#1807=CARTESIAN_POINT ( 'NONE',  ( 2.882544866740877065, -73.39547149457074227, -0.8366430509619593447 ) ) ;
#1808=CARTESIAN_POINT ( 'NONE',  ( -0.09506052544086027178, -84.00452850542926342, -6.999999999999997335 ) ) ;
#1809=CARTESIAN_POINT ( 'NONE',  ( 4.312004677471013459, -88.54547149457074795, -3.009306630940933314 ) ) ;
#1810=CARTESIAN_POINT ( 'NONE',  ( -3.015831842038216859, -63.30452850542925347, -3.989209796945429432 ) ) ;
#1811=CARTESIAN_POINT ( 'NONE',  ( 6.013306294175169597, -73.95452850542925205, 4.245374608440616093 ) ) ;
#1814=CARTESIAN_POINT ( 'NONE',  ( -1.686450176301615311, -89.29547149457074795, -2.482926158054096000 ) ) ;
#1817=CARTESIAN_POINT ( 'NONE',  ( -5.257311121191325931, -59.74547149457072948, -0.09995255151718372699 ) ) ;
#1820=CARTESIAN_POINT ( 'NONE',  ( 1.719659006605392948, -94.65452850542924068, 4.969112962950015699 ) ) ;
#1821=CARTESIAN_POINT ( 'NONE',  ( 2.493201789345269592, -62.55452850542925347, -1.934965279058294518 ) ) ;
#1822=CARTESIAN_POINT ( 'NONE',  ( -3.015831842038213306, -93.30452850542926058, -3.989209796945429432 ) ) ;
#1823=CARTESIAN_POINT ( 'NONE',  ( 2.179377348189628361, -66.64547149457072805, 7.030887037049939003 ) ) ;
#1824=CARTESIAN_POINT ( 'NONE',  ( -5.257311121191323267, -86.74547149457073658, -0.09995255151718372699 ) ) ;
#1825=CARTESIAN_POINT ( 'NONE',  ( 3.154386672714808437, -74.25452850542924921, -0.09995255151727241993 ) ) ;
#1829=CARTESIAN_POINT ( 'NONE',  ( 1.840261337453273249, -94.80452850542926058, 2.371175808195547852 ) ) ;
#1830=CARTESIAN_POINT ( 'NONE',  ( -2.369498399071058081, -69.34547149457073090, 6.969112962950058332 ) ) ;
#1834=CARTESIAN_POINT ( 'NONE',  ( -1.529537955723778930, -62.14547149457074937, -5.030887037049945221 ) ) ;
#1835=CARTESIAN_POINT ( 'NONE',  ( -1.719659006605267937, -60.34547149457073090, 4.969112962950051227 ) ) ;
#1836=CARTESIAN_POINT ( 'NONE',  ( -0.09506052544084224454, -60.00452850542925631, -4.999999999999997335 ) ) ;
#1839=CARTESIAN_POINT ( 'NONE',  ( -4.194503406049320482, -64.05452850542926058, 3.171033256558100533 ) ) ;
#1840=CARTESIAN_POINT ( 'NONE',  ( 4.784657899331175912, -61.39547149457074227, -1.454677039711874009 ) ) ;
#1846=CARTESIAN_POINT ( 'NONE',  ( 4.784657899331209663, -77.10452850542925773, 1.454677039711774533 ) ) ;
#1847=CARTESIAN_POINT ( 'NONE',  ( 3.015831842038150246, -88.69547149457073942, -3.989209796945492048 ) ) ;
#1848=CARTESIAN_POINT ( 'NONE',  ( 4.312004677471074743, -58.95452850542925205, 3.009306630940844052 ) ) ;
#1849=CARTESIAN_POINT ( 'NONE',  ( 0.09506052544077592259, -73.99547149457075079, -2.999999999999997780 ) ) ;
#1850=CARTESIAN_POINT ( 'NONE',  ( -4.191402346623178232, -81.30452850542926058, -5.607243785695311900 ) ) ;
#1851=CARTESIAN_POINT ( 'NONE',  ( 0.09506052544075677124, -88.99547149457073658, -4.999999999999997335 ) ) ;
#1853=CARTESIAN_POINT ( 'NONE',  ( 0.09506052544088175460, -79.50452850542926342, 6.999999999999997335 ) ) ;
#1854=CARTESIAN_POINT ( 'NONE',  ( -2.493201789345289132, -89.44547149457073942, -1.934965279058240561 ) ) ;
#1855=EDGE_CURVE ( 'NONE', #6384, #1139, #4766, .T. ) ;
#1858=CARTESIAN_POINT ( 'NONE',  ( -4.784657899331160813, -59.89547149457074227, 1.454677039711874675 ) ) ;
#1861=CARTESIAN_POINT ( 'NONE',  ( 3.015831842038236399, -94.80452850542924637, 3.989209796945429432 ) ) ;
#1862=CARTESIAN_POINT ( 'NONE',  ( -3.154386672714792006, -60.75452850542924921, 0.09995255151727280851 ) ) ;
#1864=CARTESIAN_POINT ( 'NONE',  ( -0.09506052544086329714, -60.00452850542925631, -6.999999999999997335 ) ) ;
#1865=CARTESIAN_POINT ( 'NONE',  ( 4.191402346623077868, -67.69547149457073942, -5.607243785695398941 ) ) ;
#1866=CARTESIAN_POINT ( 'NONE',  ( 3.015831842038149802, -85.69547149457073942, -3.989209796945492048 ) ) ;
#1867=CARTESIAN_POINT ( 'NONE',  ( 2.493201789345271369, -74.55452850542926058, -1.934965279058294518 ) ) ;
#1871=CARTESIAN_POINT ( 'NONE',  ( 1.069819614139558617, -88.65452850542926910, 2.969112962950023249 ) ) ;
#1872=CARTESIAN_POINT ( 'NONE',  ( -7.360235569667860744, -62.74547149457073658, -0.09995255151716124498 ) ) ;
#1873=CARTESIAN_POINT ( 'NONE',  ( 2.012110789770938712, -97.00000000000001421, -5.644421105825153440 ) ) ;
#1874=CARTESIAN_POINT ( 'NONE',  ( 4.725907263620371168, -61.09547149457074511, 1.635492904037598283 ) ) ;
#1875=CARTESIAN_POINT ( 'NONE',  ( -6.686770931921456551, -95.89547149457075648, 2.072711028461789784 ) ) ;
#1876=CARTESIAN_POINT ( 'NONE',  ( 0.09506052544084107880, -94.50452850542926342, 2.999999999999997780 ) ) ;
#1879=CARTESIAN_POINT ( 'NONE',  ( -2.862020680886495416, -70.20452850542925205, 4.100960146804039752 ) ) ;
#1881=CARTESIAN_POINT ( 'NONE',  ( -6.628020296210665130, -92.59547149457074511, -2.253526892787471869 ) ) ;
#1889=CARTESIAN_POINT ( 'NONE',  ( -4.784657899331190123, -81.60452850542925773, -1.454677039711773867 ) ) ;
#1890=CARTESIAN_POINT ( 'NONE',  ( 2.862020680886600221, -84.79547149457074795, 4.100960146803977580 ) ) ;
#1891=CARTESIAN_POINT ( 'NONE',  ( 3.924576421043429963, -96.99999999999988631, -1.488513849420440627 ) ) ;
#1892=CARTESIAN_POINT ( 'NONE',  ( -1.686450176301617976, -71.29547149457074795, -2.482926158054096000 ) ) ;
#1893=CARTESIAN_POINT ( 'NONE',  ( -6.686770931921506289, -78.60452850542927195, -2.072711028461647675 ) ) ;
#1894=CARTESIAN_POINT ( 'NONE',  ( -2.862020680886578905, -92.29547149457074795, -4.100960146803977580 ) ) ;
#1897=CARTESIAN_POINT ( 'NONE',  ( 4.037591185471443467, -80.70452850542925205, -5.718994135553947977 ) ) ;
#1898=CARTESIAN_POINT ( 'NONE',  ( -0.09506052544075518917, -87.49547149457075079, 2.999999999999997780 ) ) ;
#1903=CARTESIAN_POINT ( 'NONE',  ( -4.725907263620320542, -81.90452850542925489, 1.635492904037698647 ) ) ;
#1904=CARTESIAN_POINT ( 'NONE',  ( 2.610703060766947914, -97.54547149457074795, -1.773238653441125523 ) ) ;
#1905=CARTESIAN_POINT ( 'NONE',  ( 4.194503406049339134, -92.55452850542924637, -3.171033256558100089 ) ) ;
#1906=CARTESIAN_POINT ( 'NONE',  ( 6.013306294175077227, -73.54547149457074795, -4.245374608440741326 ) ) ;
#1907=CARTESIAN_POINT ( 'NONE',  ( 4.312004677471013459, -85.54547149457073374, -3.009306630940932425 ) ) ;
#1908=CARTESIAN_POINT ( 'NONE',  ( -1.686450176301566017, -76.20452850542925205, 2.482926158054133303 ) ) ;
#1911=CARTESIAN_POINT ( 'NONE',  ( 1.840261337453271917, -85.80452850542926058, 2.371175808195547852 ) ) ;
#1912=CARTESIAN_POINT ( 'NONE',  ( 2.369498399071075845, -64.84547149457071669, -6.969112962950057444 ) ) ;
#1915=CARTESIAN_POINT ( 'NONE',  ( -5.257311121191325043, -62.74547149457074369, -0.09995255151718372699 ) ) ;
#1916=CARTESIAN_POINT ( 'NONE',  ( 5.895805022753496161, -93.94547149457073942, 4.407101234057782868 ) ) ;
#1920=CARTESIAN_POINT ( 'NONE',  ( 4.725907263620340082, -68.40452850542925489, -1.635492904037697981 ) ) ;
#1921=CARTESIAN_POINT ( 'NONE',  ( -2.179377348189609265, -89.14547149457072805, -7.030887037049939003 ) ) ;
#1927=CARTESIAN_POINT ( 'NONE',  ( -5.257311121191324155, -78.75452850542924921, 0.09995255151729526277 ) ) ;
#1928=CARTESIAN_POINT ( 'NONE',  ( -3.015831842038129373, -75.19547149457073942, 3.989209796945492048 ) ) ;
#1930=CARTESIAN_POINT ( 'NONE',  ( -2.493201789345292241, -68.44547149457073942, -1.934965279058240561 ) ) ;
#1931=CARTESIAN_POINT ( 'NONE',  ( -7.360235569667858968, -75.75452850542926342, 0.09995255151731782806 ) ) ;
#1932=CARTESIAN_POINT ( 'NONE',  ( 5.257311121191341918, -76.24547149457073658, 0.09995255151718437925 ) ) ;
#1934=CARTESIAN_POINT ( 'NONE',  ( -4.725907263620324095, -57.90452850542925489, 1.635492904037698647 ) ) ;
#1936=CARTESIAN_POINT ( 'NONE',  ( 2.179377348189481811, -77.85452850542925773, -7.030887037049986077 ) ) ;
#1937=CARTESIAN_POINT ( 'NONE',  ( -2.823794231030039459, -83.59547149457075932, -1.017458915287723364 ) ) ;
#1942=CARTESIAN_POINT ( 'NONE',  ( -5.257311121191323267, -84.75452850542923500, 0.09995255151729526277 ) ) ;
#1944=CARTESIAN_POINT ( 'NONE',  ( 4.784657899331209663, -77.10452850542925773, 1.454677039711774533 ) ) ;
#1945=CARTESIAN_POINT ( 'NONE',  ( 0.8796985632578967484, -59.85452850542925773, -3.030887037049972310 ) ) ;
#1947=CARTESIAN_POINT ( 'NONE',  ( -4.312004677471055203, -93.45452850542922363, -3.009306630940844052 ) ) ;
#1950=CARTESIAN_POINT ( 'NONE',  ( -0.09506052544071530441, -66.49547149457075079, 6.999999999999997335 ) ) ;
#1951=CARTESIAN_POINT ( 'NONE',  ( 1.529537955723797360, -90.64547149457075648, 5.030887037049945221 ) ) ;
#1952=CARTESIAN_POINT ( 'NONE',  ( -3.154386672714790674, -72.75452850542926342, 0.09995255151727280851 ) ) ;
#1953=AXIS2_PLACEMENT_3D ( 'NONE', #1496, #776, #4106 ) ;
#1956=CARTESIAN_POINT ( 'NONE',  ( -2.610703060766963901, -84.45452850542925205, -1.773238653441072232 ) ) ;
#1957=CARTESIAN_POINT ( 'NONE',  ( 0.09506052544073274879, -64.99547149457075079, -6.999999999999997335 ) ) ;
#1959=CARTESIAN_POINT ( 'NONE',  ( 1.529537955723794473, -66.64547149457072805, 5.030887037049945221 ) ) ;
#1960=CARTESIAN_POINT ( 'NONE',  ( 4.312004677471010794, -61.54547149457073374, -3.009306630940933314 ) ) ;
#1964=CARTESIAN_POINT ( 'NONE',  ( -4.784657899331191899, -60.60452850542925773, -1.454677039711773867 ) ) ;
#1965=CARTESIAN_POINT ( 'NONE',  ( -2.369498399071055417, -90.34547149457073090, 6.969112962950058332 ) ) ;
#1967=CARTESIAN_POINT ( 'NONE',  ( 1.529537955723689890, -74.85452850542925773, -5.030887037049978971 ) ) ;
#1971=CARTESIAN_POINT ( 'NONE',  ( -1.719659006605264384, -84.34547149457071669, 4.969112962950051227 ) ) ;
#1972=CARTESIAN_POINT ( 'NONE',  ( 4.282105902239295325, -96.99999999999998579, 2.536915707574844525 ) ) ;
#1973=CARTESIAN_POINT ( 'NONE',  ( 2.823794231030058555, -67.09547149457073090, 1.017458915287723809 ) ) ;
#1974=CARTESIAN_POINT ( 'NONE',  ( 6.013306294175168709, -70.95452850542925205, 4.245374608440616093 ) ) ;
#1976=CARTESIAN_POINT ( 'NONE',  ( 0.09506052544075600796, -82.99547149457075079, -4.999999999999997335 ) ) ;
#1977=CARTESIAN_POINT ( 'NONE',  ( 5.257311121191341918, -62.25452850542924921, -0.09995255151729465215 ) ) ;
#1978=CARTESIAN_POINT ( 'NONE',  ( 3.015831842038235955, -91.80452850542926058, 3.989209796945429432 ) ) ;
#1979=CARTESIAN_POINT ( 'NONE',  ( -7.360235569667858968, -72.75452850542926342, 0.09995255151731782806 ) ) ;
#1980=CARTESIAN_POINT ( 'NONE',  ( 2.882544866740877509, -76.39547149457074227, -0.8366430509619593447 ) ) ;
#1985=CARTESIAN_POINT ( 'NONE',  ( 1.529537955723691889, -86.85452850542921510, -5.030887037049978971 ) ) ;
#1987=CARTESIAN_POINT ( 'NONE',  ( -4.194503406049316929, -79.05452850542923215, 3.171033256558101865 ) ) ;
#1988=CARTESIAN_POINT ( 'NONE',  ( -2.493201789345254493, -58.05452850542925347, 1.934965279058294518 ) ) ;
#1990=CARTESIAN_POINT ( 'NONE',  ( -4.312004677471056979, -84.45452850542922363, -3.009306630940844052 ) ) ;
#1991=CARTESIAN_POINT ( 'NONE',  ( 5.895805022753407343, -92.55452850542926058, -4.407101234057908989 ) ) ;
#1992=CARTESIAN_POINT ( 'NONE',  ( -4.725907263620353405, -80.59547149457074511, -1.635492904037597617 ) ) ;
#1993=CARTESIAN_POINT ( 'NONE',  ( -0.8796985632578793179, -76.35452850542924352, 3.030887037049973198 ) ) ;
#1996=CARTESIAN_POINT ( 'NONE',  ( -2.823794231030019919, -84.90452850542926910, 1.017458915287783316 ) ) ;
#1997=CARTESIAN_POINT ( 'NONE',  ( -4.037591185471547384, -59.29547149457074084, -5.718994135553860936 ) ) ;
#1999=CARTESIAN_POINT ( 'NONE',  ( -4.194503406049316041, -79.05452850542921794, 3.171033256558100533 ) ) ;
#2000=CARTESIAN_POINT ( 'NONE',  ( 6.686770931921479644, -94.39547149457074227, -2.072711028461788896 ) ) ;
#2003=CARTESIAN_POINT ( 'NONE',  ( 1.719659006605388285, -58.65452850542924068, 4.969112962950016588 ) ) ;
#2004=CARTESIAN_POINT ( 'NONE',  ( 4.037591185471564259, -90.79547149457074795, 5.718994135553860936 ) ) ;
#2007=CARTESIAN_POINT ( 'NONE',  ( -1.719659006605371854, -78.15452850542925489, -4.969112962950016588 ) ) ;
#2011=CARTESIAN_POINT ( 'NONE',  ( -5.257311121191323267, -83.74547149457075079, -0.09995255151718371311 ) ) ;
#2013=CARTESIAN_POINT ( 'NONE',  ( 1.840261337453218626, -61.69547149457074653, -2.371175808195584267 ) ) ;
#2015=CARTESIAN_POINT ( 'NONE',  ( -2.179377348189461827, -73.35452850542924352, 7.030887037049988741 ) ) ;
#2018=CARTESIAN_POINT ( 'NONE',  ( 1.719659006605285922, -76.84547149457073090, -4.969112962950050338 ) ) ;
#2019=APPLICATION_CONTEXT ( 'automotive_design' ) ;
#2020=CARTESIAN_POINT ( 'NONE',  ( 0.09506052544085819012, -61.50452850542925631, 4.999999999999997335 ) ) ;
#2021=CARTESIAN_POINT ( 'NONE',  ( -2.862020680886492752, -88.20452850542925205, 4.100960146804039752 ) ) ;
#2022=CARTESIAN_POINT ( 'NONE',  ( 2.179377348189480923, -68.85452850542924352, -7.030887037049986077 ) ) ;
#2023=CARTESIAN_POINT ( 'NONE',  ( 1.686450176301585335, -77.70452850542925205, -2.482926158054133303 ) ) ;
#2024=CARTESIAN_POINT ( 'NONE',  ( 2.882544866740877954, -79.39547149457074227, -0.8366430509619593447 ) ) ;
#2028=CARTESIAN_POINT ( 'NONE',  ( 0.09506052544086121547, -85.50452850542926342, 4.999999999999997335 ) ) ;
#2030=CARTESIAN_POINT ( 'NONE',  ( -1.719659006605371854, -81.15452850542924068, -4.969112962950015699 ) ) ;
#2031=CARTESIAN_POINT ( 'NONE',  ( -1.840261337453198198, -93.19547149457075363, 2.371175808195584267 ) ) ;
#2034=CARTESIAN_POINT ( 'NONE',  ( 3.015831842038235511, -88.80452850542926058, 3.989209796945429432 ) ) ;
#2036=CARTESIAN_POINT ( 'NONE',  ( 6.628020296210686446, -64.09547149457071669, 2.253526892787472757 ) ) ;
#2037=CARTESIAN_POINT ( 'NONE',  ( 1.840261337453269253, -64.80452850542926058, 2.371175808195547852 ) ) ;
#2040=CARTESIAN_POINT ( 'NONE',  ( -1.686450176301564241, -88.20452850542925205, 2.482926158054133303 ) ) ;
#2042=CARTESIAN_POINT ( 'NONE',  ( -6.013306294175061240, -66.04547149457074795, 4.245374608440741326 ) ) ;
#2044=CARTESIAN_POINT ( 'NONE',  ( -3.015831842038215083, -75.30452850542926058, -3.989209796945429432 ) ) ;
#2045=CARTESIAN_POINT ( 'NONE',  ( 4.037591185471564259, -87.79547149457074795, 5.718994135553860936 ) ) ;
#2048=CARTESIAN_POINT ( 'NONE',  ( -0.09506052544075783983, -66.49547149457075079, 2.999999999999997780 ) ) ;
#2049=CARTESIAN_POINT ( 'NONE',  ( 6.013306294175080779, -88.54547149457074795, -4.245374608440741326 ) ) ;
#2052=CARTESIAN_POINT ( 'NONE',  ( -0.09506052544084073186, -72.00452850542926342, -4.999999999999997335 ) ) ;
#2056=CARTESIAN_POINT ( 'NONE',  ( -2.862020680886580237, -80.29547149457074795, -4.100960146803977580 ) ) ;
#2057=CARTESIAN_POINT ( 'NONE',  ( 4.239768230324508558, -96.99999999999998579, 2.450885936931344045 ) ) ;
#2058=CARTESIAN_POINT ( 'NONE',  ( 2.493201789345308228, -63.94547149457074653, 1.934965279058241006 ) ) ;
#2059=CARTESIAN_POINT ( 'NONE',  ( -4.191402346623179120, -72.30452850542926058, -5.607243785695311900 ) ) ;
#2061=CARTESIAN_POINT ( 'NONE',  ( -1.719659006605265272, -75.34547149457074511, 4.969112962950051227 ) ) ;
#2062=CARTESIAN_POINT ( 'NONE',  ( -4.312004677471056091, -87.45452850542925205, -3.009306630940844052 ) ) ;
#2063=CARTESIAN_POINT ( 'NONE',  ( -6.628020296210620721, -72.90452850542925489, 2.253526892787613978 ) ) ;
#2064=CARTESIAN_POINT ( 'NONE',  ( 0.09506052544077592259, -73.99547149457075079, -2.999999999999997780 ) ) ;
#2068=CARTESIAN_POINT ( 'NONE',  ( 4.312004677471078296, -91.95452850542925205, 3.009306630940844496 ) ) ;
#2070=CARTESIAN_POINT ( 'NONE',  ( -0.09506052544083998246, -78.00452850542926342, -4.999999999999997335 ) ) ;
#2071=CARTESIAN_POINT ( 'NONE',  ( 2.882544866740879286, -91.39547149457074227, -0.8366430509619593447 ) ) ;
#2073=CARTESIAN_POINT ( 'NONE',  ( 0.09506052544086084077, -82.50452850542926342, 4.999999999999997335 ) ) ;
#2074=CARTESIAN_POINT ( 'NONE',  ( -2.179377348189612817, -62.14547149457074937, -7.030887037049939003 ) ) ;
#2075=CARTESIAN_POINT ( 'NONE',  ( 2.823794231030038571, -62.40452850542925489, -1.017458915287783316 ) ) ;
#2078=CARTESIAN_POINT ( 'NONE',  ( 0.8796985632578994130, -80.85452850542925773, -3.030887037049972310 ) ) ;
#2079=CARTESIAN_POINT ( 'NONE',  ( 4.191402346623198660, -88.80452850542926058, 5.607243785695311900 ) ) ;
#2082=CARTESIAN_POINT ( 'NONE',  ( -0.09506052544071304233, -84.49547149457075079, 6.999999999999997335 ) ) ;
#2085=CARTESIAN_POINT ( 'NONE',  ( 2.823794231030058999, -70.09547149457073090, 1.017458915287723809 ) ) ;
#2089=CARTESIAN_POINT ( 'NONE',  ( 4.725907263620340082, -71.40452850542925489, -1.635492904037697981 ) ) ;
#2090=CARTESIAN_POINT ( 'NONE',  ( 6.013306294175077227, -76.54547149457074795, -4.245374608440741326 ) ) ;
#2094=CARTESIAN_POINT ( 'NONE',  ( 4.784657899331209663, -77.10452850542925773, 1.454677039711774533 ) ) ;
#2098=CARTESIAN_POINT ( 'NONE',  ( -1.529537955723776710, -80.14547149457072805, -5.030887037049945221 ) ) ;
#2100=CARTESIAN_POINT ( 'NONE',  ( 4.725907263620375609, -97.09547149457074511, 1.635492904037598283 ) ) ;
#2101=CARTESIAN_POINT ( 'NONE',  ( -6.013306294175152722, -72.45452850542925205, -4.245374608440613429 ) ) ;
#2103=CARTESIAN_POINT ( 'NONE',  ( -4.725907263620353405, -74.59547149457074511, -1.635492904037597617 ) ) ;
#2104=CARTESIAN_POINT ( 'NONE',  ( -1.529537955723668796, -85.35452850542924352, 5.030887037049979860 ) ) ;
#2105=CARTESIAN_POINT ( 'NONE',  ( -4.037591185471423039, -73.20452850542925205, 5.718994135553947977 ) ) ;
#2106=CARTESIAN_POINT ( 'NONE',  ( -2.493201789345290464, -83.44547149457073942, -1.934965279058240561 ) ) ;
#2109=CARTESIAN_POINT ( 'NONE',  ( 1.529537955723692555, -92.85452850542925773, -5.030887037049978971 ) ) ;
#2110=CARTESIAN_POINT ( 'NONE',  ( 2.862020680886514956, -83.70452850542925205, -4.100960146804039752 ) ) ;
#2112=CARTESIAN_POINT ( 'NONE',  ( -5.257311121191325043, -75.75452850542923500, 0.09995255151729529053 ) ) ;
#2113=CARTESIAN_POINT ( 'NONE',  ( 1.069819614139496000, -88.84547149457073090, -2.969112962950042789 ) ) ;
#2115=CARTESIAN_POINT ( 'NONE',  ( 3.015831842038235067, -85.80452850542926058, 3.989209796945429432 ) ) ;
#2116=CARTESIAN_POINT ( 'NONE',  ( 6.013306294175077227, -64.54547149457073374, -4.245374608440741326 ) ) ;
#2118=CARTESIAN_POINT ( 'NONE',  ( 1.686450176301584003, -65.70452850542925205, -2.482926158054133303 ) ) ;
#2121=CARTESIAN_POINT ( 'NONE',  ( -1.686450176301566017, -76.20452850542925205, 2.482926158054133303 ) ) ;
#2122=CARTESIAN_POINT ( 'NONE',  ( -0.09506052544085988321, -87.00452850542926342, -6.999999999999997335 ) ) ;
#2123=CARTESIAN_POINT ( 'NONE',  ( 2.369498399071079398, -91.84547149457074511, -6.969112962950057444 ) ) ;
#2126=DIRECTION ( 'NONE',  ( -1.000000000000000000, -1.261617073437677752E-16, 0.000000000000000000 ) ) ;
#2127=CARTESIAN_POINT ( 'NONE',  ( -2.493201789345292241, -65.44547149457075363, -1.934965279058240561 ) ) ;
#2130=CARTESIAN_POINT ( 'NONE',  ( -1.719659006605372964, -72.15452850542921226, -4.969112962950016588 ) ) ;
#2131=CARTESIAN_POINT ( 'NONE',  ( 6.013306294175077227, -79.54547149457074795, -4.245374608440741326 ) ) ;
#2132=FILL_AREA_STYLE_COLOUR ( '', #7005 ) ;
#2135=CARTESIAN_POINT ( 'NONE',  ( 0.09506052544085932809, -70.50452850542926342, 4.999999999999997335 ) ) ;
#2138=CARTESIAN_POINT ( 'NONE',  ( -2.862020680886580681, -74.29547149457074795, -4.100960146803977580 ) ) ;
#2140=CARTESIAN_POINT ( 'NONE',  ( 1.529537955723798026, -96.64547149457071384, 5.030887037049945221 ) ) ;
#2141=CARTESIAN_POINT ( 'NONE',  ( -4.037591185471424815, -64.20452850542925205, 5.718994135553947977 ) ) ;
#2144=CARTESIAN_POINT ( 'NONE',  ( 2.862020680886514956, -83.70452850542925205, -4.100960146804039752 ) ) ;
#2145=CARTESIAN_POINT ( 'NONE',  ( 0.09506052544088025580, -67.50452850542926342, 6.999999999999997335 ) ) ;
#2147=CARTESIAN_POINT ( 'NONE',  ( 1.686450176301636183, -78.79547149457074795, 2.482926158054096000 ) ) ;
#2152=CARTESIAN_POINT ( 'NONE',  ( 4.725907263620340082, -77.40452850542925489, -1.635492904037697981 ) ) ;
#2154=CARTESIAN_POINT ( 'NONE',  ( -1.719659006605373408, -69.15452850542924068, -4.969112962950015699 ) ) ;
#2155=CARTESIAN_POINT ( 'NONE',  ( 2.493201789345311781, -90.94547149457073942, 1.934965279058241006 ) ) ;
#2156=CARTESIAN_POINT ( 'NONE',  ( 2.882544866740875289, -61.39547149457074937, -0.8366430509619593447 ) ) ;
#2158=CARTESIAN_POINT ( 'NONE',  ( 2.179377348189627472, -60.64547149457074227, 7.030887037049939003 ) ) ;
#2159=CARTESIAN_POINT ( 'NONE',  ( -1.840261337453253487, -63.30452850542926058, -2.371175808195547852 ) ) ;
#2163=CARTESIAN_POINT ( 'NONE',  ( 2.493201789345271369, -74.55452850542926058, -1.934965279058294518 ) ) ;
#2164=CARTESIAN_POINT ( 'NONE',  ( 5.895805022753407343, -89.55452850542926058, -4.407101234057908989 ) ) ;
#2165=CARTESIAN_POINT ( 'NONE',  ( 4.037591185471564259, -90.79547149457074795, 5.718994135553860936 ) ) ;
#2168=CARTESIAN_POINT ( 'NONE',  ( -2.610703060766927042, -66.04547149457074795, 1.773238653441125745 ) ) ;
#2172=CARTESIAN_POINT ( 'NONE',  ( 2.862020680886513180, -68.70452850542925205, -4.100960146804039752 ) ) ;
#2173=CARTESIAN_POINT ( 'NONE',  ( 6.686770931921477867, -76.39547149457074227, -2.072711028461788896 ) ) ;
#2176=CARTESIAN_POINT ( 'NONE',  ( 5.257311121191341918, -68.25452850542926342, -0.09995255151729465215 ) ) ;
#2179=CARTESIAN_POINT ( 'NONE',  ( -4.194503406049384431, -68.44547149457073942, -3.171033256558012159 ) ) ;
#2181=CARTESIAN_POINT ( 'NONE',  ( -1.069819614139476460, -63.34547149457073800, 2.969112962950044121 ) ) ;
#2182=CARTESIAN_POINT ( 'NONE',  ( 4.037591185471440802, -59.70452850542925916, -5.718994135553947977 ) ) ;
#2185=CARTESIAN_POINT ( 'NONE',  ( -3.015831842038214194, -81.30452850542926058, -3.989209796945429432 ) ) ;
#2186=CARTESIAN_POINT ( 'NONE',  ( -2.369498399071207739, -63.15452850542925489, -6.969112962950009482 ) ) ;
#2187=CARTESIAN_POINT ( 'NONE',  ( 1.840261337453219959, -73.69547149457073942, -2.371175808195584267 ) ) ;
#2191=CARTESIAN_POINT ( 'NONE',  ( -4.725907263620321430, -75.90452850542925489, 1.635492904037698647 ) ) ;
#2193=CARTESIAN_POINT ( 'NONE',  ( 4.312004677471075631, -70.95452850542925205, 3.009306630940844052 ) ) ;
#2194=CARTESIAN_POINT ( 'NONE',  ( -3.154386672714787565, -92.74547149457073658, -0.09995255151720625064 ) ) ;
#2195=CARTESIAN_POINT ( 'NONE',  ( 0.09506052544077400746, -58.99547149457073658, -2.999999999999997780 ) ) ;
#2196=CARTESIAN_POINT ( 'NONE',  ( -2.862020680886494972, -73.20452850542925205, 4.100960146804039752 ) ) ;
#2197=CARTESIAN_POINT ( 'NONE',  ( 0.09506052544088325340, -91.50452850542926342, 6.999999999999997335 ) ) ;
#2198=CARTESIAN_POINT ( 'NONE',  ( -3.154386672714791118, -66.75452850542926342, 0.09995255151727280851 ) ) ;
#2203=CARTESIAN_POINT ( 'NONE',  ( 2.610703060766983885, -79.95452850542925205, 1.773238653441072232 ) ) ;
#2204=CARTESIAN_POINT ( 'NONE',  ( 2.179377348189483143, -89.85452850542924352, -7.030887037049986077 ) ) ;
#2205=CARTESIAN_POINT ( 'NONE',  ( -2.369498399071055861, -87.34547149457073090, 6.969112962950058332 ) ) ;
#2209=CARTESIAN_POINT ( 'NONE',  ( -1.840261337453201529, -69.19547149457073942, 2.371175808195584267 ) ) ;
#2214=CARTESIAN_POINT ( 'NONE',  ( -4.784657899331191011, -66.60452850542924352, -1.454677039711773867 ) ) ;
#2215=CARTESIAN_POINT ( 'NONE',  ( -6.628020296210667794, -80.59547149457075932, -2.253526892787471869 ) ) ;
#2217=CARTESIAN_POINT ( 'NONE',  ( -4.784657899331158148, -74.89547149457074227, 1.454677039711874675 ) ) ;
#2219=CARTESIAN_POINT ( 'NONE',  ( 5.257311121191341918, -65.25452850542926342, -0.09995255151729465215 ) ) ;
#2223=AXIS2_PLACEMENT_3D ( 'NONE', #6216, #1675, #441 ) ;
#2224=CARTESIAN_POINT ( 'NONE',  ( -4.725907263620355181, -65.59547149457073090, -1.635492904037597617 ) ) ;
#2226=CARTESIAN_POINT ( 'NONE',  ( 4.784657899331179465, -94.39547149457074227, -1.454677039711874009 ) ) ;
#2227=CARTESIAN_POINT ( 'NONE',  ( -6.686770931921507177, -60.60452850542926484, -2.072711028461647675 ) ) ;
#2231=EDGE_LOOP ( 'NONE', ( #8196, #4744, #7445, #5754, #7625 ) ) ;
#2233=CARTESIAN_POINT ( 'NONE',  ( -4.312004677471056979, -84.45452850542922363, -3.009306630940844052 ) ) ;
#2234=CARTESIAN_POINT ( 'NONE',  ( -4.784657899331190123, -81.60452850542925773, -1.454677039711773867 ) ) ;
#2236=CARTESIAN_POINT ( 'NONE',  ( 2.862020680886513624, -71.70452850542925205, -4.100960146804039752 ) ) ;
#2237=CARTESIAN_POINT ( 'NONE',  ( -2.610703060766926153, -78.04547149457074795, 1.773238653441125745 ) ) ;
#2238=CARTESIAN_POINT ( 'NONE',  ( 3.015831842038151134, -94.69547149457075363, -3.989209796945492048 ) ) ;
#2239=CARTESIAN_POINT ( 'NONE',  ( 2.862020680886514512, -77.70452850542926626, -4.100960146804039752 ) ) ;
#2240=CARTESIAN_POINT ( 'NONE',  ( -2.179377348189459607, -91.35452850542925773, 7.030887037049988741 ) ) ;
#2241=CARTESIAN_POINT ( 'NONE',  ( -2.823794231030038571, -95.59547149457074511, -1.017458915287723364 ) ) ;
#2243=ORIENTED_EDGE ( 'NONE', *, *, #83, .T. ) ;
#2247=CARTESIAN_POINT ( 'NONE',  ( -2.610703060766964345, -81.45452850542925205, -1.773238653441072232 ) ) ;
#2248=CARTESIAN_POINT ( 'NONE',  ( -6.686770931921504513, -84.60452850542927195, -2.072711028461647675 ) ) ;
#2249=CARTESIAN_POINT ( 'NONE',  ( -6.013306294175058575, -81.04547149457074795, 4.245374608440741326 ) ) ;
#2251=CARTESIAN_POINT ( 'NONE',  ( -4.312004677470990366, -96.04547149457074795, 3.009306630940933314 ) ) ;
#2252=CARTESIAN_POINT ( 'NONE',  ( 2.493201789345272701, -86.55452850542926058, -1.934965279058294518 ) ) ;
#2257=CARTESIAN_POINT ( 'NONE',  ( 0.09506052544085932809, -70.50452850542926342, 4.999999999999997335 ) ) ;
#2258=CARTESIAN_POINT ( 'NONE',  ( -6.686770931921458327, -80.89547149457074227, 2.072711028461789784 ) ) ;
#2260=CARTESIAN_POINT ( 'NONE',  ( 3.015831842038148469, -73.69547149457073942, -3.989209796945492048 ) ) ;
#2261=CARTESIAN_POINT ( 'NONE',  ( -3.015831842038130262, -66.19547149457075363, 3.989209796945492048 ) ) ;
#2262=CARTESIAN_POINT ( 'NONE',  ( -3.015831842038216859, -63.30452850542925347, -3.989209796945429432 ) ) ;
#2264=CARTESIAN_POINT ( 'NONE',  ( -4.784657899331158148, -74.89547149457074227, 1.454677039711874675 ) ) ;
#2267=CARTESIAN_POINT ( 'NONE',  ( -4.191402346623180897, -60.30452850542926058, -5.607243785695311900 ) ) ;
#2272=CARTESIAN_POINT ( 'NONE',  ( -1.719659006605371188, -84.15452850542925489, -4.969112962950016588 ) ) ;
#2273=CARTESIAN_POINT ( 'NONE',  ( 1.719659006605391172, -76.65452850542922647, 4.969112962950016588 ) ) ;
#2275=CARTESIAN_POINT ( 'NONE',  ( -4.194503406049319594, -67.05452850542926058, 3.171033256558101865 ) ) ;
#2276=CARTESIAN_POINT ( 'NONE',  ( -2.882544866740857969, -77.89547149457074227, 0.8366430509619596778 ) ) ;
#2277=CARTESIAN_POINT ( 'NONE',  ( -4.784657899331155484, -95.89547149457074227, 1.454677039711874675 ) ) ;
#2278=CARTESIAN_POINT ( 'NONE',  ( -5.257311121191324155, -72.75452850542924921, 0.09995255151729526277 ) ) ;
#2279=CARTESIAN_POINT ( 'NONE',  ( -4.037591185471421262, -91.20452850542925205, 5.718994135553947977 ) ) ;
#2280=CARTESIAN_POINT ( 'NONE',  ( 1.069819614139497332, -97.84547149457073090, -2.969112962950042789 ) ) ;
#2286=CARTESIAN_POINT ( 'NONE',  ( 0.8796985632578976366, -65.85452850542924352, -3.030887037049972310 ) ) ;
#2288=CARTESIAN_POINT ( 'NONE',  ( 4.312004677471013459, -88.54547149457074795, -3.009306630940932425 ) ) ;
#2290=CARTESIAN_POINT ( 'NONE',  ( -2.179377348189610153, -83.14547149457072805, -7.030887037049939003 ) ) ;
#2293=CARTESIAN_POINT ( 'NONE',  ( 4.194503406049403083, -93.94547149457075363, 3.171033256558012159 ) ) ;
#2294=CARTESIAN_POINT ( 'NONE',  ( 2.823794231030042123, -89.40452850542926910, -1.017458915287783316 ) ) ;
#2299=CARTESIAN_POINT ( 'NONE',  ( -0.09506052544081705635, -93.00452850542926342, -2.999999999999997780 ) ) ;
#2300=CARTESIAN_POINT ( 'NONE',  ( 6.013306294175077227, -67.54547149457074795, -4.245374608440741326 ) ) ;
#2301=SHAPE_REPRESENTATION_RELATIONSHIP ( 'NONE' , 'NONE' ,  #1066, #3582 ) ;
#2303=CARTESIAN_POINT ( 'NONE',  ( 1.529537955723795584, -78.64547149457074227, 5.030887037049945221 ) ) ;
#2304=CARTESIAN_POINT ( 'NONE',  ( 5.257311121191341918, -70.24547149457075079, 0.09995255151718437925 ) ) ;
#2305=CARTESIAN_POINT ( 'NONE',  ( 4.194503406049335581, -68.55452850542926058, -3.171033256558100089 ) ) ;
#2307=CARTESIAN_POINT ( 'NONE',  ( -1.529537955723777598, -74.14547149457074227, -5.030887037049945221 ) ) ;
#2309=CARTESIAN_POINT ( 'NONE',  ( -0.09506052544083770650, -96.00452850542926342, -4.999999999999997335 ) ) ;
#2314=CARTESIAN_POINT ( 'NONE',  ( 4.725907263620341858, -89.40452850542926910, -1.635492904037697981 ) ) ;
#2315=CARTESIAN_POINT ( 'NONE',  ( -0.09506052544083998246, -78.00452850542926342, -4.999999999999997335 ) ) ;
#2316=CARTESIAN_POINT ( 'NONE',  ( 4.784657899331207886, -59.10452850542925773, 1.454677039711774533 ) ) ;
#2317=CARTESIAN_POINT ( 'NONE',  ( 0.8796985632579624736, -81.64547149457074227, 3.030887037049952326 ) ) ;
#2318=CARTESIAN_POINT ( 'NONE',  ( -1.840261337453202639, -60.19547149457074653, 2.371175808195584267 ) ) ;
#2319=CARTESIAN_POINT ( 'NONE',  ( 4.725907263620340082, -68.40452850542925489, -1.635492904037697981 ) ) ;
#2320=CARTESIAN_POINT ( 'NONE',  ( 2.369498399071227279, -91.65452850542924068, 6.969112962950009482 ) ) ;
#2321=CARTESIAN_POINT ( 'NONE',  ( -2.610703060766967010, -60.45452850542925916, -1.773238653441072232 ) ) ;
#2328=CARTESIAN_POINT ( 'NONE',  ( 0.09506052544083769262, -67.50452850542926342, 2.999999999999997780 ) ) ;
#2329=CARTESIAN_POINT ( 'NONE',  ( -6.686770931921459216, -77.89547149457074227, 2.072711028461789784 ) ) ;
#2331=CARTESIAN_POINT ( 'NONE',  ( -5.257311121191322378, -92.74547149457073658, -0.09995255151718372699 ) ) ;
#2332=CARTESIAN_POINT ( 'NONE',  ( -1.840261337453249935, -90.30452850542926058, -2.371175808195547852 ) ) ;
#2336=CARTESIAN_POINT ( 'NONE',  ( -3.154386672714787565, -93.75452850542926342, 0.09995255151727280851 ) ) ;
#2337=CARTESIAN_POINT ( 'NONE',  ( 7.360235569667877620, -70.24547149457075079, 0.09995255151716216091 ) ) ;
#2338=CARTESIAN_POINT ( 'NONE',  ( 1.023909817990208637, -97.00000000000002842, -5.931815031828092444 ) ) ;
#2339=CARTESIAN_POINT ( 'NONE',  ( -0.09506052544073578803, -72.49547149457075079, 4.999999999999997335 ) ) ;
#2340=CARTESIAN_POINT ( 'NONE',  ( 3.015831842038148469, -73.69547149457073942, -3.989209796945492048 ) ) ;
#2341=CARTESIAN_POINT ( 'NONE',  ( -2.862020680886496304, -61.20452850542925205, 4.100960146804039752 ) ) ;
#2346=CARTESIAN_POINT ( 'NONE',  ( 0.09506052544075337118, -61.99547149457074369, -4.999999999999997335 ) ) ;
#2349=CARTESIAN_POINT ( 'NONE',  ( -1.719659006605370744, -93.15452850542925489, -4.969112962950016588 ) ) ;
#2351=MECHANICAL_DESIGN_GEOMETRIC_PRESENTATION_REPRESENTATION('',(#5975),#725);
#2357=CARTESIAN_POINT ( 'NONE',  ( 0.09506052544086084077, -82.50452850542926342, 4.999999999999997335 ) ) ;
#2358=CARTESIAN_POINT ( 'NONE',  ( -4.194503406049382654, -92.44547149457073942, -3.171033256558012159 ) ) ;
#2359=CARTESIAN_POINT ( 'NONE',  ( 2.862020680886512736, -65.70452850542925205, -4.100960146804039752 ) ) ;
#2360=CARTESIAN_POINT ( 'NONE',  ( 2.823794231030060331, -82.09547149457075932, 1.017458915287723809 ) ) ;
#2361=CARTESIAN_POINT ( 'NONE',  ( -0.09506052544073390065, -87.49547149457075079, 4.999999999999997335 ) ) ;
#2362=CARTESIAN_POINT ( 'NONE',  ( -1.719659006605373630, -66.15452850542926910, -4.969112962950016588 ) ) ;
#2363=CARTESIAN_POINT ( 'NONE',  ( 6.686770931921524941, -83.10452850542927195, 2.072711028461649008 ) ) ;
#2364=CARTESIAN_POINT ( 'NONE',  ( 2.882544866740879730, -94.39547149457074227, -0.8366430509619593447 ) ) ;
#2368=CARTESIAN_POINT ( 'NONE',  ( 1.529537955723691889, -86.85452850542924352, -5.030887037049978971 ) ) ;
#2369=CARTESIAN_POINT ( 'NONE',  ( -0.8796985632578802061, -70.35452850542922931, 3.030887037049973198 ) ) ;
#2371=CARTESIAN_POINT ( 'NONE',  ( -2.369498399071057637, -75.34547149457073090, 6.969112962950058332 ) ) ;
#2372=CARTESIAN_POINT ( 'NONE',  ( 4.194503406049339134, -92.55452850542924637, -3.171033256558100089 ) ) ;
#2374=CARTESIAN_POINT ( 'NONE',  ( -1.840261337453250157, -87.30452850542926058, -2.371175808195547852 ) ) ;
#2377=CARTESIAN_POINT ( 'NONE',  ( 5.257311121191341918, -59.25452850542924210, -0.09995255151729465215 ) ) ;
#2378=CARTESIAN_POINT ( 'NONE',  ( 0.09506052544073390065, -73.99547149457075079, -6.999999999999997335 ) ) ;
#2382=CARTESIAN_POINT ( 'NONE',  ( 4.725907263620372945, -76.09547149457074511, 1.635492904037598283 ) ) ;
#2383=CARTESIAN_POINT ( 'NONE',  ( -2.862020680886581125, -71.29547149457074795, -4.100960146803977580 ) ) ;
#2384=CARTESIAN_POINT ( 'NONE',  ( -4.725907263620324095, -57.90452850542925489, 1.635492904037698647 ) ) ;
#2386=CARTESIAN_POINT ( 'NONE',  ( -4.725907263620322318, -66.90452850542925489, 1.635492904037698647 ) ) ;
#2387=CARTESIAN_POINT ( 'NONE',  ( 5.257311121191341918, -61.24547149457074369, 0.09995255151718437925 ) ) ;
#2392=CARTESIAN_POINT ( 'NONE',  ( 3.015831842038235067, -85.80452850542926058, 3.989209796945429432 ) ) ;
#2394=CARTESIAN_POINT ( 'NONE',  ( 4.784657899331179465, -91.39547149457075648, -1.454677039711874009 ) ) ;
#2395=CARTESIAN_POINT ( 'NONE',  ( 4.784657899331208775, -65.10452850542924352, 1.454677039711774533 ) ) ;
#2396=CARTESIAN_POINT ( 'NONE',  ( 2.882544866740878398, -85.39547149457074227, -0.8366430509619593447 ) ) ;
#2397=CARTESIAN_POINT ( 'NONE',  ( -6.686770931921504513, -81.60452850542927195, -2.072711028461647675 ) ) ;
#2398=CARTESIAN_POINT ( 'NONE',  ( 1.529537955723796028, -84.64547149457074227, 5.030887037049945221 ) ) ;
#2400=CARTESIAN_POINT ( 'NONE',  ( -4.784657899331191011, -66.60452850542924352, -1.454677039711773867 ) ) ;
#2401=CARTESIAN_POINT ( 'NONE',  ( 4.191402346623198660, -82.80452850542926058, 5.607243785695311900 ) ) ;
#2402=CARTESIAN_POINT ( 'NONE',  ( 2.493201789345269148, -59.55452850542924637, -1.934965279058294518 ) ) ;
#2406=CARTESIAN_POINT ( 'NONE',  ( -4.725907263620319654, -90.90452850542926910, 1.635492904037698647 ) ) ;
#2407=CARTESIAN_POINT ( 'NONE',  ( -2.610703060766965677, -72.45452850542925205, -1.773238653441072232 ) ) ;
#2408=CARTESIAN_POINT ( 'NONE',  ( -0.09506052544086367184, -57.00452850542925631, -6.999999999999997335 ) ) ;
#2409=CARTESIAN_POINT ( 'NONE',  ( 0.09506052544073312349, -67.99547149457075079, -6.999999999999997335 ) ) ;
#2410=CARTESIAN_POINT ( 'NONE',  ( 3.015831842038149802, -82.69547149457073942, -3.989209796945492048 ) ) ;
#2411=CARTESIAN_POINT ( 'NONE',  ( -2.610703060766963901, -84.45452850542925205, -1.773238653441072232 ) ) ;
#2414=( LENGTH_UNIT ( ) NAMED_UNIT ( * ) SI_UNIT ( .MILLI., .METRE. ) );
#2415=CARTESIAN_POINT ( 'NONE',  ( 0.09506052544085819012, -61.50452850542925631, 4.999999999999997335 ) ) ;
#2417=CARTESIAN_POINT ( 'NONE',  ( 6.686770931921476979, -70.39547149457072805, -2.072711028461788896 ) ) ;
#2420=CARTESIAN_POINT ( 'NONE',  ( 3.015831842038147137, -64.69547149457075363, -3.989209796945492048 ) ) ;
#2421=CARTESIAN_POINT ( 'NONE',  ( 1.719659006605283924, -64.84547149457071669, -4.969112962950050338 ) ) ;
#2422=CARTESIAN_POINT ( 'NONE',  ( 2.493201789345273589, -92.55452850542926058, -1.934965279058294518 ) ) ;
#2425=CARTESIAN_POINT ( 'NONE',  ( -0.09506052544084110656, -69.00452850542926342, -4.999999999999997335 ) ) ;
#2427=CARTESIAN_POINT ( 'NONE',  ( 6.686770931921480532, -97.39547149457074227, -2.072711028461788896 ) ) ;
#2433=CARTESIAN_POINT ( 'NONE',  ( -1.529537955723670795, -73.35452850542922931, 5.030887037049979860 ) ) ;
#2434=CARTESIAN_POINT ( 'NONE',  ( -4.194503406049382654, -89.44547149457073942, -3.171033256558012159 ) ) ;
#2435=CARTESIAN_POINT ( 'NONE',  ( -2.862020680886495860, -64.20452850542926626, 4.100960146804039752 ) ) ;
#2436=CARTESIAN_POINT ( 'NONE',  ( 2.493201789345308672, -66.94547149457073942, 1.934965279058241006 ) ) ;
#2437=CARTESIAN_POINT ( 'NONE',  ( 6.628020296210642037, -83.40452850542925489, -2.253526892787612645 ) ) ;
#2438=CARTESIAN_POINT ( 'NONE',  ( 4.312004677471013459, -91.54547149457074795, -3.009306630940933314 ) ) ;
#2439=CARTESIAN_POINT ( 'NONE',  ( -4.194503406049319594, -70.05452850542923215, 3.171033256558100533 ) ) ;
#2440=CARTESIAN_POINT ( 'NONE',  ( 6.013306294175169597, -79.95452850542925205, 4.245374608440616093 ) ) ;
#2441=CARTESIAN_POINT ( 'NONE',  ( -2.882544866740855749, -89.89547149457074227, 0.8366430509619596778 ) ) ;
#2446=CARTESIAN_POINT ( 'NONE',  ( -5.257311121191322378, -87.75452850542923500, 0.09995255151729529053 ) ) ;
#2447=CARTESIAN_POINT ( 'NONE',  ( -2.882544866740878398, -69.60452850542924352, -0.8366430509618996147 ) ) ;
#2449=CARTESIAN_POINT ( 'NONE',  ( 2.862020680886516732, -95.70452850542926626, -4.100960146804039752 ) ) ;
#2450=CARTESIAN_POINT ( 'NONE',  ( -4.191402346623058328, -69.19547149457073942, 5.607243785695398941 ) ) ;
#2451=CARTESIAN_POINT ( 'NONE',  ( 4.194503406049403083, -81.94547149457073942, 3.171033256558012159 ) ) ;
#2452=CARTESIAN_POINT ( 'NONE',  ( 2.882544866740897049, -80.10452850542927195, 0.8366430509618999478 ) ) ;
#2456=CARTESIAN_POINT ( 'NONE',  ( 2.493201789345274033, -95.55452850542926058, -1.934965279058294518 ) ) ;
#2457=CARTESIAN_POINT ( 'NONE',  ( 2.179377348189629249, -75.64547149457072805, 7.030887037049939003 ) ) ;
#2460=CARTESIAN_POINT ( 'NONE',  ( 4.366652375515289286, -96.99999999999995737, 2.564342289837593380 ) ) ;
#2461=CARTESIAN_POINT ( 'NONE',  ( 4.784657899331176800, -67.39547149457074227, -1.454677039711874009 ) ) ;
#2462=CARTESIAN_POINT ( 'NONE',  ( -3.015831842038130706, -63.19547149457074653, 3.989209796945492048 ) ) ;
#2463=CARTESIAN_POINT ( 'NONE',  ( -1.686450176301563353, -94.20452850542928047, 2.482926158054133303 ) ) ;
#2465=CARTESIAN_POINT ( 'NONE',  ( 5.257311121191341918, -68.25452850542926342, -0.09995255151729465215 ) ) ;
#2466=CARTESIAN_POINT ( 'NONE',  ( -7.360235569667856304, -95.74547149457073658, -0.09995255151716124498 ) ) ;
#2474=CARTESIAN_POINT ( 'NONE',  ( 3.015831842038234178, -79.80452850542926058, 3.989209796945429432 ) ) ;
#2476=CARTESIAN_POINT ( 'NONE',  ( -5.257311121191323267, -86.74547149457072237, -0.09995255151718371311 ) ) ;
#2477=CARTESIAN_POINT ( 'NONE',  ( -1.719659006605374518, -60.15452850542926200, -4.969112962950015699 ) ) ;
#2478=CARTESIAN_POINT ( 'NONE',  ( 1.686450176301634851, -66.79547149457073374, 2.482926158054096000 ) ) ;
#2479=CARTESIAN_POINT ( 'NONE',  ( -5.895805022753386027, -76.05452850542926058, 4.407101234057909878 ) ) ;
#2480=CARTESIAN_POINT ( 'NONE',  ( -1.529537955723776044, -86.14547149457074227, -5.030887037049945221 ) ) ;
#2481=CARTESIAN_POINT ( 'NONE',  ( -1.529537955723671683, -64.35452850542924352, 5.030887037049979860 ) ) ;
#2482=CARTESIAN_POINT ( 'NONE',  ( -7.360235569667858968, -78.75452850542926342, 0.09995255151731782806 ) ) ;
#2483=CIRCLE ( 'NONE', #1953, 0.9999999999999948930 ) ;
#2484=CARTESIAN_POINT ( 'NONE',  ( 3.154386672714810658, -88.24547149457073658, 0.09995255151720662534 ) ) ;
#2490=CARTESIAN_POINT ( 'NONE',  ( 4.194503406049340022, -95.55452850542924637, -3.171033256558100977 ) ) ;
#2491=CARTESIAN_POINT ( 'NONE',  ( 3.154386672714806217, -59.25452850542926342, -0.09995255151727241993 ) ) ;
#2492=CARTESIAN_POINT ( 'NONE',  ( -5.257311121191321490, -93.75452850542926342, 0.09995255151729526277 ) ) ;
#2493=CARTESIAN_POINT ( 'NONE',  ( -5.895805022753479285, -71.44547149457072521, -4.407101234057782868 ) ) ;
#2494=CARTESIAN_POINT ( 'NONE',  ( 5.257311121191342806, -85.24547149457075079, 0.09995255151718437925 ) ) ;
#2495=CARTESIAN_POINT ( 'NONE',  ( -1.840261337453251933, -75.30452850542926058, -2.371175808195547852 ) ) ;
#2498=CARTESIAN_POINT ( 'NONE',  ( 3.154386672714809770, -86.25452850542924921, -0.09995255151727241993 ) ) ;
#2499=CARTESIAN_POINT ( 'NONE',  ( 6.013306294175077227, -64.54547149457073374, -4.245374608440741326 ) ) ;
#2500=CARTESIAN_POINT ( 'NONE',  ( 4.827973024309449634, -96.99999999999998579, 2.218963830005241444 ) ) ;
#2501=CARTESIAN_POINT ( 'NONE',  ( 0.09506052544075374588, -64.99547149457075079, -4.999999999999997335 ) ) ;
#2502=CARTESIAN_POINT ( 'NONE',  ( -2.862020680886582014, -62.29547149457074084, -4.100960146803977580 ) ) ;
#2503=CARTESIAN_POINT ( 'NONE',  ( -4.312004677471061420, -57.45452850542925916, -3.009306630940844052 ) ) ;
#2505=CARTESIAN_POINT ( 'NONE',  ( -4.194503406049319594, -67.05452850542926058, 3.171033256558100533 ) ) ;
#2506=CARTESIAN_POINT ( 'NONE',  ( 5.895805022753498825, -96.94547149457073942, 4.407101234057782868 ) ) ;
#2512=CARTESIAN_POINT ( 'NONE',  ( -4.784657899331190123, -75.60452850542925773, -1.454677039711773867 ) ) ;
#2513=CARTESIAN_POINT ( 'NONE',  ( 5.257311121191341918, -85.24547149457075079, 0.09995255151718437925 ) ) ;
#2514=CARTESIAN_POINT ( 'NONE',  ( 4.277672441867257369, -96.99999999999992895, 1.818343915288929136 ) ) ;
#2515=CARTESIAN_POINT ( 'NONE',  ( -3.154386672714790674, -74.74547149457073658, -0.09995255151720625064 ) ) ;
#2516=CARTESIAN_POINT ( 'NONE',  ( 5.895805022753406455, -77.55452850542926058, -4.407101234057908989 ) ) ;
#2517=CARTESIAN_POINT ( 'NONE',  ( -4.725907263620351628, -89.59547149457074511, -1.635492904037597617 ) ) ;
#2519=CARTESIAN_POINT ( 'NONE',  ( 0.09506052544088212930, -82.50452850542926342, 6.999999999999997335 ) ) ;
#2520=CARTESIAN_POINT ( 'NONE',  ( -1.069819614139472463, -90.34547149457073090, 2.969112962950044121 ) ) ;
#2527=CARTESIAN_POINT ( 'NONE',  ( 4.725907263620341858, -86.40452850542926910, -1.635492904037697981 ) ) ;
#2528=CARTESIAN_POINT ( 'NONE',  ( 3.154386672714807105, -62.25452850542926342, -0.09995255151727241993 ) ) ;
#2530=CARTESIAN_POINT ( 'NONE',  ( 1.719659006605392504, -94.65452850542921226, 4.969112962950016588 ) ) ;
#2531=CARTESIAN_POINT ( 'NONE',  ( 4.191402346623077868, -70.69547149457073942, -5.607243785695398941 ) ) ;
#2532=EDGE_CURVE ( 'NONE', #4976, #7927, #2483, .T. ) ;
#2533=CARTESIAN_POINT ( 'NONE',  ( -3.015831842038127153, -90.19547149457073942, 3.989209796945492048 ) ) ;
#2534=CARTESIAN_POINT ( 'NONE',  ( -2.823794231030020807, -78.90452850542925489, 1.017458915287783316 ) ) ;
#2536=( NAMED_UNIT ( * ) SI_UNIT ( $, .STERADIAN. ) SOLID_ANGLE_UNIT ( ) );
#2537=CARTESIAN_POINT ( 'NONE',  ( 1.840261337453272583, -88.80452850542926058, 2.371175808195547852 ) ) ;
#2538=CARTESIAN_POINT ( 'NONE',  ( 0.09506052544073236021, -61.99547149457073658, -6.999999999999997335 ) ) ;
#2540=CARTESIAN_POINT ( 'NONE',  ( -4.312004677470993919, -69.04547149457071953, 3.009306630940933314 ) ) ;
#2541=CARTESIAN_POINT ( 'NONE',  ( -4.725907263620356069, -59.59547149457074511, -1.635492904037597617 ) ) ;
#2542=CARTESIAN_POINT ( 'NONE',  ( 1.840261337453272805, -91.80452850542926058, 2.371175808195547852 ) ) ;
#2545=CIRCLE ( 'NONE', #4825, 0.9999999999999948930 ) ;
#2546=CARTESIAN_POINT ( 'NONE',  ( 3.015831842038232402, -64.80452850542926058, 3.989209796945429432 ) ) ;
#2547=CARTESIAN_POINT ( 'NONE',  ( 6.686770931921479644, -94.39547149457074227, -2.072711028461788896 ) ) ;
#2557=CARTESIAN_POINT ( 'NONE',  ( 1.719659006605391172, -76.65452850542922647, 4.969112962950016588 ) ) ;
#2558=CARTESIAN_POINT ( 'NONE',  ( -0.09506052544073466393, -81.49547149457075079, 4.999999999999997335 ) ) ;
#2559=CARTESIAN_POINT ( 'NONE',  ( 2.919221509273758119, -96.99999999999992895, -2.847688208160571666 ) ) ;
#2560=CARTESIAN_POINT ( 'NONE',  ( 2.610703060766944361, -70.54547149457074795, -1.773238653441125523 ) ) ;
#2561=CARTESIAN_POINT ( 'NONE',  ( -2.369498399071206407, -81.15452850542924068, -6.969112962950009482 ) ) ;
#2562=CARTESIAN_POINT ( 'NONE',  ( 4.784657899331178577, -82.39547149457074227, -1.454677039711874009 ) ) ;
#2563=CARTESIAN_POINT ( 'NONE',  ( -4.312004677471060532, -60.45452850542923784, -3.009306630940844052 ) ) ;
#2565=CARTESIAN_POINT ( 'NONE',  ( -2.179377348189461383, -79.35452850542927195, 7.030887037049988741 ) ) ;
#2566=CARTESIAN_POINT ( 'NONE',  ( -3.154386672714789341, -83.74547149457075079, -0.09995255151720625064 ) ) ;
#2569=CARTESIAN_POINT ( 'NONE',  ( -1.529537955723779374, -59.14547149457073516, -5.030887037049945221 ) ) ;
#2571=CARTESIAN_POINT ( 'NONE',  ( -4.312004677471057867, -78.45452850542925205, -3.009306630940843608 ) ) ;
#2572=CARTESIAN_POINT ( 'NONE',  ( -1.686450176301568016, -58.20452850542925916, 2.482926158054133303 ) ) ;
#2573=CARTESIAN_POINT ( 'NONE',  ( -6.686770931921508954, -57.60452850542926484, -2.072711028461647675 ) ) ;
#2574=CARTESIAN_POINT ( 'NONE',  ( -6.628020296210667794, -68.59547149457073090, -2.253526892787471869 ) ) ;
#2575=CARTESIAN_POINT ( 'NONE',  ( -4.312004677470991254, -90.04547149457073374, 3.009306630940933314 ) ) ;
#2576=CARTESIAN_POINT ( 'NONE',  ( 1.686450176301585335, -74.70452850542925205, -2.482926158054133303 ) ) ;
#2579=CARTESIAN_POINT ( 'NONE',  ( -2.493201789345250496, -88.05452850542926058, 1.934965279058294518 ) ) ;
#2580=CARTESIAN_POINT ( 'NONE',  ( -6.013306294175062128, -60.04547149457073374, 4.245374608440741326 ) ) ;
#2582=CARTESIAN_POINT ( 'NONE',  ( -3.015831842038130706, -63.19547149457074653, 3.989209796945492048 ) ) ;
#2583=CARTESIAN_POINT ( 'NONE',  ( -4.194503406049384431, -59.44547149457074653, -3.171033256558012159 ) ) ;
#2586=CARTESIAN_POINT ( 'NONE',  ( 4.784657899331207886, -59.10452850542925773, 1.454677039711774533 ) ) ;
#2587=CARTESIAN_POINT ( 'NONE',  ( 2.369498399071078953, -88.84547149457073090, -6.969112962950057444 ) ) ;
#2590=CARTESIAN_POINT ( 'NONE',  ( 1.529537955723689224, -71.85452850542925773, -5.030887037049978971 ) ) ;
#2597=CARTESIAN_POINT ( 'NONE',  ( 4.725907263620372945, -76.09547149457074511, 1.635492904037598283 ) ) ;
#2598=CARTESIAN_POINT ( 'NONE',  ( 2.480136385090595308, -96.99999999999992895, -3.206978988282922050 ) ) ;
#2599=CARTESIAN_POINT ( 'NONE',  ( 2.610703060766944361, -67.54547149457074795, -1.773238653441125523 ) ) ;
#2600=CARTESIAN_POINT ( 'NONE',  ( -7.360235569667858968, -72.75452850542926342, 0.09995255151731782806 ) ) ;
#2602=CARTESIAN_POINT ( 'NONE',  ( -4.194503406049384431, -80.44547149457073942, -3.171033256558012159 ) ) ;
#2605=CARTESIAN_POINT ( 'NONE',  ( -4.784657899331188347, -93.60452850542925773, -1.454677039711773867 ) ) ;
#2606=CARTESIAN_POINT ( 'NONE',  ( 2.179377348189480479, -65.85452850542924352, -7.030887037049986077 ) ) ;
#2607=CARTESIAN_POINT ( 'NONE',  ( 1.686450176301635961, -75.79547149457074795, 2.482926158054096000 ) ) ;
#2610=DIRECTION ( 'NONE',  ( -0.09506052544079829358, 0.9954714945707483498, 0.000000000000000000 ) ) ;
#2612=CARTESIAN_POINT ( 'NONE',  ( -4.725907263620319654, -87.90452850542926910, 1.635492904037698647 ) ) ;
#2614=CARTESIAN_POINT ( 'NONE',  ( 4.194503406049339134, -80.55452850542926058, -3.171033256558100977 ) ) ;
#2615=CARTESIAN_POINT ( 'NONE',  ( 1.840261337453222845, -97.69547149457076785, -2.371175808195584267 ) ) ;
#2618=CARTESIAN_POINT ( 'NONE',  ( -2.862020680886492752, -88.20452850542925205, 4.100960146804039752 ) ) ;
#2621=CARTESIAN_POINT ( 'NONE',  ( -4.037591185471546495, -62.29547149457074084, -5.718994135553860936 ) ) ;
#2622=CARTESIAN_POINT ( 'NONE',  ( -4.312004677470992142, -81.04547149457071953, 3.009306630940933314 ) ) ;
#2623=CARTESIAN_POINT ( 'NONE',  ( 3.154386672714808437, -71.25452850542926342, -0.09995255151727241993 ) ) ;
#2628=CARTESIAN_POINT ( 'NONE',  ( -1.686450176301564685, -85.20452850542925205, 2.482926158054133303 ) ) ;
#2629=CARTESIAN_POINT ( 'NONE',  ( 4.037591185471445243, -95.70452850542928047, -5.718994135553947977 ) ) ;
#2631=CARTESIAN_POINT ( 'NONE',  ( -0.09506052544083960776, -81.00452850542926342, -4.999999999999997335 ) ) ;
#2632=CARTESIAN_POINT ( 'NONE',  ( 4.037591185471565147, -96.79547149457073374, 5.718994135553860936 ) ) ;
#2636=CARTESIAN_POINT ( 'NONE',  ( 5.257311121191341918, -59.25452850542924210, -0.09995255151729465215 ) ) ;
#2638=CARTESIAN_POINT ( 'NONE',  ( 2.369498399071079398, -91.84547149457074511, -6.969112962950057444 ) ) ;
#2641=CARTESIAN_POINT ( 'NONE',  ( 4.312004677471074743, -70.95452850542925205, 3.009306630940844496 ) ) ;
#2644=CARTESIAN_POINT ( 'NONE',  ( -0.09506052544073541333, -75.49547149457073658, 4.999999999999997335 ) ) ;
#2645=CARTESIAN_POINT ( 'NONE',  ( 3.534712008015381102, -97.00000000000002842, -2.138372830837821148 ) ) ;
#2646=CARTESIAN_POINT ( 'NONE',  ( -2.823794231030041235, -65.59547149457073090, -1.017458915287723364 ) ) ;
#2647=CARTESIAN_POINT ( 'NONE',  ( -4.037591185471423927, -70.20452850542925205, 5.718994135553947977 ) ) ;
#2649=CARTESIAN_POINT ( 'NONE',  ( -1.529537955723777154, -77.14547149457074227, -5.030887037049945221 ) ) ;
#2650=CARTESIAN_POINT ( 'NONE',  ( 1.719659006605388507, -61.65452850542923358, 4.969112962950016588 ) ) ;
#2651=CARTESIAN_POINT ( 'NONE',  ( 4.194503406049339134, -86.55452850542926058, -3.171033256558100089 ) ) ;
#2652=CARTESIAN_POINT ( 'NONE',  ( 4.191402346623196884, -70.80452850542926058, 5.607243785695311900 ) ) ;
#2653=CARTESIAN_POINT ( 'NONE',  ( 1.840261337453220625, -76.69547149457073942, -2.371175808195584267 ) ) ;
#2657=CARTESIAN_POINT ( 'NONE',  ( -4.194503406049314265, -94.05452850542926058, 3.171033256558100533 ) ) ;
#2658=CARTESIAN_POINT ( 'NONE',  ( 2.862020680886516288, -92.70452850542926626, -4.100960146804039752 ) ) ;
#2660=CARTESIAN_POINT ( 'NONE',  ( -2.862020680886493196, -85.20452850542925205, 4.100960146804039752 ) ) ;
#2661=CARTESIAN_POINT ( 'NONE',  ( 1.840261337453268808, -61.80452850542926058, 2.371175808195547852 ) ) ;
#2662=CARTESIAN_POINT ( 'NONE',  ( -4.312004677471056091, -90.45452850542926626, -3.009306630940844052 ) ) ;
#2663=CARTESIAN_POINT ( 'NONE',  ( -7.360235569667860744, -59.74547149457073658, -0.09995255151716124498 ) ) ;
#2664=CARTESIAN_POINT ( 'NONE',  ( 2.493201789345270480, -68.55452850542926058, -1.934965279058294518 ) ) ;
#2669=CARTESIAN_POINT ( 'NONE',  ( -1.840261337453249935, -90.30452850542926058, -2.371175808195547852 ) ) ;
#2670=CARTESIAN_POINT ( 'NONE',  ( 2.369498399071227723, -94.65452850542924068, 6.969112962950009482 ) ) ;
#2672=B_SPLINE_CURVE_WITH_KNOTS ( 'NONE', 3,
 ( #3679, #4262, #2338, #553, #1873, #1746, #8152, #6835, #1067, #5610, #6960, #6876, #3089, #6373, #3173, #5649, #472, #4304, #3640, #6250, #6919, #6206, #1787, #2500, #8189, #1154, #8229, #430, #8111, #2460, #3003, #3722 ),
 .UNSPECIFIED., .F., .F.,
 ( 4, 2, 2, 2, 2, 2, 2, 2, 2, 2, 2, 2, 2, 2, 2, 4 ),
 ( 0.000000000000000000, 0.001531221420384391721, 0.002296832130576588124, 0.003062442840768784310, 0.004593664261153176248, 0.005359274971345372868, 0.006124885681537568620, 0.007656107101921958390, 0.009187328522306347292, 0.009952939232498542177, 0.01071854994269073533, 0.01148416065288293195, 0.01186696600797902852, 0.01205836868552707768, 0.01215407002430110225, 0.01224977136307512857 ),
 .UNSPECIFIED. ) ;
#2673=CARTESIAN_POINT ( 'NONE',  ( -4.312004677471057867, -78.45452850542925205, -3.009306630940844052 ) ) ;
#2674=CARTESIAN_POINT ( 'NONE',  ( 2.179377348189631469, -93.64547149457074227, 7.030887037049939003 ) ) ;
#2677=CARTESIAN_POINT ( 'NONE',  ( 0.09506052544077515931, -67.99547149457075079, -2.999999999999997780 ) ) ;
#2678=CARTESIAN_POINT ( 'NONE',  ( 2.862020680886511848, -59.70452850542925205, -4.100960146804039752 ) ) ;
#2679=CARTESIAN_POINT ( 'NONE',  ( 2.179377348189631469, -93.64547149457074227, 7.030887037049939003 ) ) ;
#2681=CARTESIAN_POINT ( 'NONE',  ( -0.09506052544083998246, -78.00452850542926342, -4.999999999999997335 ) ) ;
#2686=CARTESIAN_POINT ( 'NONE',  ( -2.369498399071058081, -69.34547149457073090, 6.969112962950058332 ) ) ;
#2687=CARTESIAN_POINT ( 'NONE',  ( 3.015831842038149357, -79.69547149457075363, -3.989209796945492048 ) ) ;
#2689=CARTESIAN_POINT ( 'NONE',  ( -2.823794231030042567, -59.59547149457074511, -1.017458915287723364 ) ) ;
#2691=CARTESIAN_POINT ( 'NONE',  ( -0.09506052544086217304, -69.00452850542926342, -6.999999999999997335 ) ) ;
#2693=CARTESIAN_POINT ( 'NONE',  ( 1.529537955723795584, -75.64547149457069963, 5.030887037049945221 ) ) ;
#2694=CARTESIAN_POINT ( 'NONE',  ( -4.725907263620320542, -84.90452850542925489, 1.635492904037698647 ) ) ;
#2695=CARTESIAN_POINT ( 'NONE',  ( -6.628020296210622497, -69.90452850542925489, 2.253526892787613978 ) ) ;
#2697=CARTESIAN_POINT ( 'NONE',  ( 0.09506052544077629729, -76.99547149457075079, -2.999999999999997780 ) ) ;
#2701=CARTESIAN_POINT ( 'NONE',  ( -0.09506052544083846978, -90.00452850542924921, -4.999999999999997335 ) ) ;
#2703=CARTESIAN_POINT ( 'NONE',  ( 4.725907263620340970, -83.40452850542925489, -1.635492904037697981 ) ) ;
#2704=CARTESIAN_POINT ( 'NONE',  ( -1.840261337453198864, -90.19547149457073942, 2.371175808195584267 ) ) ;
#2706=CARTESIAN_POINT ( 'NONE',  ( 1.529537955723692111, -89.85452850542925773, -5.030887037049978971 ) ) ;
#2707=CARTESIAN_POINT ( 'NONE',  ( 2.369498399071227723, -94.65452850542924068, 6.969112962950009482 ) ) ;
#2708=CARTESIAN_POINT ( 'NONE',  ( 3.154386672714807105, -65.25452850542926342, -0.09995255151727241993 ) ) ;
#2713=CARTESIAN_POINT ( 'NONE',  ( -3.154386672714789341, -81.75452850542926342, 0.09995255151727280851 ) ) ;
#2714=CARTESIAN_POINT ( 'NONE',  ( 2.369498399071225947, -85.65452850542926910, 6.969112962950009482 ) ) ;
#2716=CARTESIAN_POINT ( 'NONE',  ( -0.09506052544071189048, -93.49547149457075079, 6.999999999999997335 ) ) ;
#2719=CARTESIAN_POINT ( 'NONE',  ( 2.610703060766944361, -67.54547149457074795, -1.773238653441125523 ) ) ;
#2720=CARTESIAN_POINT ( 'NONE',  ( 4.725907263620339194, -59.40452850542926200, -1.635492904037697981 ) ) ;
#2722=CARTESIAN_POINT ( 'NONE',  ( 4.784657899331208775, -65.10452850542924352, 1.454677039711774533 ) ) ;
#2723=CARTESIAN_POINT ( 'NONE',  ( 4.191402346623079644, -85.69547149457073942, -5.607243785695398941 ) ) ;
#2725=CARTESIAN_POINT ( 'NONE',  ( 4.194503406049337357, -77.55452850542926058, -3.171033256558100089 ) ) ;
#2728=CARTESIAN_POINT ( 'NONE',  ( 4.312004677471012570, -79.54547149457074795, -3.009306630940933314 ) ) ;
#2731=CARTESIAN_POINT ( 'NONE',  ( 1.069819614139492447, -61.84547149457074511, -2.969112962950042789 ) ) ;
#2732=CARTESIAN_POINT ( 'NONE',  ( -4.037591185471423039, -73.20452850542925205, 5.718994135553947977 ) ) ;
#2734=CARTESIAN_POINT ( 'NONE',  ( 4.194503406049402194, -81.94547149457073942, 3.171033256558012159 ) ) ;
#2735=CARTESIAN_POINT ( 'NONE',  ( -0.09506052544083846978, -90.00452850542924921, -4.999999999999997335 ) ) ;
#2736=CARTESIAN_POINT ( 'NONE',  ( -7.360235569667858968, -66.75452850542926342, 0.09995255151731782806 ) ) ;
#2737=CARTESIAN_POINT ( 'NONE',  ( -2.493201789345290464, -80.44547149457073942, -1.934965279058240561 ) ) ;
#2740=CARTESIAN_POINT ( 'NONE',  ( 0.09506052544086235345, -94.50452850542926342, 4.999999999999997335 ) ) ;
#2741=CARTESIAN_POINT ( 'NONE',  ( -3.015831842038213750, -87.30452850542926058, -3.989209796945429432 ) ) ;
#2744=CARTESIAN_POINT ( 'NONE',  ( 4.194503406049338246, -77.55452850542926058, -3.171033256558100977 ) ) ;
#2745=CARTESIAN_POINT ( 'NONE',  ( -2.823794231030038571, -89.59547149457074511, -1.017458915287723364 ) ) ;
#2746=CARTESIAN_POINT ( 'NONE',  ( -5.257311121191322378, -87.75452850542922079, 0.09995255151729526277 ) ) ;
#2747=CARTESIAN_POINT ( 'NONE',  ( 6.686770931921525829, -95.10452850542925773, 2.072711028461649008 ) ) ;
#2749=CARTESIAN_POINT ( 'NONE',  ( 2.823794231030039459, -68.40452850542925489, -1.017458915287783316 ) ) ;
#2752=CARTESIAN_POINT ( 'NONE',  ( 1.069819614139557729, -82.65452850542926910, 2.969112962950023249 ) ) ;
#2754=CARTESIAN_POINT ( 'NONE',  ( 4.037591185471444355, -86.70452850542925205, -5.718994135553947977 ) ) ;
#2757=CARTESIAN_POINT ( 'NONE',  ( 0.09506052544073574639, -88.99547149457075079, -6.999999999999997335 ) ) ;
#2761=CARTESIAN_POINT ( 'NONE',  ( -1.840261337453201973, -66.19547149457073942, 2.371175808195584267 ) ) ;
#2764=CARTESIAN_POINT ( 'NONE',  ( 1.529537955723689224, -71.85452850542925773, -5.030887037049978971 ) ) ;
#2765=CARTESIAN_POINT ( 'NONE',  ( 5.895805022753496161, -81.94547149457073942, 4.407101234057782868 ) ) ;
#2767=CARTESIAN_POINT ( 'NONE',  ( 2.862020680886514068, -74.70452850542926626, -4.100960146804039752 ) ) ;
#2770=CARTESIAN_POINT ( 'NONE',  ( 1.719659006605285478, -73.84547149457074511, -4.969112962950050338 ) ) ;
#2772=CARTESIAN_POINT ( 'NONE',  ( 1.840261337453218848, -64.69547149457073942, -2.371175808195584267 ) ) ;
#2773=CARTESIAN_POINT ( 'NONE',  ( -6.013306294175152722, -66.45452850542925205, -4.245374608440613429 ) ) ;
#2776=CARTESIAN_POINT ( 'NONE',  ( -4.312004677471056979, -84.45452850542922363, -3.009306630940844052 ) ) ;
#2777=CARTESIAN_POINT ( 'NONE',  ( 6.628020296210639373, -71.40452850542924068, -2.253526892787612645 ) ) ;
#2778=CARTESIAN_POINT ( 'NONE',  ( -3.154386672714789341, -80.74547149457075079, -0.09995255151720625064 ) ) ;
#2781=CARTESIAN_POINT ( 'NONE',  ( 2.862020680886516288, -92.70452850542926626, -4.100960146804039752 ) ) ;
#2782=CARTESIAN_POINT ( 'NONE',  ( 5.257311121191341918, -83.25452850542926342, -0.09995255151729465215 ) ) ;
#2784=CARTESIAN_POINT ( 'NONE',  ( 1.719659006605390061, -70.65452850542926910, 4.969112962950015699 ) ) ;
#2785=CARTESIAN_POINT ( 'NONE',  ( 1.840261337453221513, -88.69547149457073942, -2.371175808195584267 ) ) ;
#2786=CARTESIAN_POINT ( 'NONE',  ( -0.09506052544083884448, -87.00452850542924921, -4.999999999999997335 ) ) ;
#2787=CARTESIAN_POINT ( 'NONE',  ( -2.179377348189459163, -94.35452850542925773, 7.030887037049988741 ) ) ;
#2788=CARTESIAN_POINT ( 'NONE',  ( 2.882544866740894829, -65.10452850542924352, 0.8366430509618999478 ) ) ;
#2793=CARTESIAN_POINT ( 'NONE',  ( -2.823794231030020807, -78.90452850542925489, 1.017458915287783316 ) ) ;
#2794=CARTESIAN_POINT ( 'NONE',  ( -0.09506052544085913381, -93.00452850542926342, -6.999999999999997335 ) ) ;
#2796=CARTESIAN_POINT ( 'NONE',  ( 4.037591185471563371, -84.79547149457074795, 5.718994135553860936 ) ) ;
#2798=( BOUNDED_CURVE ( )  B_SPLINE_CURVE ( 2, ( #3583, #6109, #1015, #2490, #7626, #3792, #8140, #4291, #1861, #1820, #5595, #1140, #3665, #5051, #3119, #7670, #5674, #1180, #1734, #3625, #4372, #3033, #1054, #6192, #6863, #1223, #6233, #6947, #1093, #5637, #459, #418, #8177, #4328, #2406, #4967, #7543, #6364, #6322, #1773, #8256, #4409, #3748, #6902, #3709, #6279, #6991, #581, #4251, #3163, #541, #497, #2991, #3075, #8218, #2446, #5008, #7581, #5718, #8297, #5557, #2368, #7504, #4931, #2527, #5090, #6821, #4579, #7711, #3332, #3377, #7843, #2660, #3957, #3999, #663, #751, #6442, #5758, #7798, #5218, #7163, #795, #621, #2703, #3246, #1386, #1346, #6529, #4452, #5176, #706, #6485, #1432, #1903, #3290, #5802, #5890, #6403, #2030, #4622, #31, #5849, #2614, #120, #1261, #5262, #3917, #4558, #5936, #7755, #77, #164, #1987, #7033, #3833, #3202, #2571, #4537, #7118, #2070, #6569, #7207, #2744, #5305, #5132, #1944, #4497, #7076, #1303, #3873, #6769, #3455, #364, #3417, #2112, #6731, #6652, #2863, #6139, #1555, #7888, #3491, #3570, #2941, #4043, #5981, #1004, #881, #4120, #4666, #6019, #7247, #1473, #6610, #837, #7968, #243, #8008, #5426, #4836, #2823, #2236, #5387, #4080, #205, #6688, #2193, #3530, #2784, #5343, #7414, #7928, #919, #1595, #6062, #4745, #962, #7329, #2154, #286, #4708, #4792, #7366, #7286, #1512, #4160, #1639, #6098, #325, #2904, #5469, #8048, #2275, #4199, #5585, #1722, #8129, #5547, #5040, #7569, #1044, #2359, #3108, #3063, #6853, #2395, #4921, #3737, #4361, #569, #6935, #2435, #4955, #408, #7532, #1806, #2981, #3655, #3614, #6223, #1084, #4242, #486, #6811, #6890, #6307, #529, #446, #5663, #7493, #8166, #4280, #8089, #8244, #3023, #1682, #5624, #5508, #2477, #6182, #8205, #4997, #6976, #1763, #4318, #2316, #1848, #4880, #1124, #7613, #3698, #1169, #4398, #6268, #1211, #3781, #7452, #6351, #7021, #3941 ),
 .UNSPECIFIED., .F., .T. ) 
 B_SPLINE_CURVE_WITH_KNOTS ( ( 3, 2, 2, 2, 2, 2, 2, 2, 2, 2, 2, 2, 2, 2, 2, 2, 2, 2, 2, 2, 2, 2, 2, 2, 2, 2, 2, 2, 2, 2, 2, 2, 2, 2, 2, 2, 2, 2, 2, 2, 2, 2, 2, 2, 2, 2, 2, 2, 2, 2, 2, 2, 2, 2, 2, 2, 2, 2, 2, 2, 2, 2, 2, 2, 2, 2, 2, 2, 2, 2, 2, 2, 2, 2, 2, 2, 2, 2, 2, 2, 2, 2, 2, 2, 2, 2, 2, 2, 2, 2, 2, 2, 2, 2, 2, 2, 2, 2, 2, 2, 2, 2, 2, 2, 2, 2, 2, 2, 2, 2, 2, 2, 2, 2, 2, 2, 2, 2, 2, 2, 2, 2, 2, 2, 2, 2, 2, 2, 2, 2, 3 ),
 ( 0.000000000000000000, 0.007692307692307692735, 0.01538461538461538547, 0.02307692307692307820, 0.03076923076923077094, 0.03846153846153846367, 0.04615384615384615641, 0.05384615384615384914, 0.06153846153846154188, 0.06923076923076923461, 0.07692307692307692735, 0.08461538461538462008, 0.09230769230769231282, 0.1000000000000000056, 0.1076923076923076983, 0.1153846153846153910, 0.1230769230769230838, 0.1307692307692307765, 0.1384615384615384692, 0.1461538461538461620, 0.1538461538461538547, 0.1615384615384615474, 0.1692307692307692402, 0.1769230769230769329, 0.1846153846153846256, 0.1923076923076923184, 0.2000000000000000111, 0.2076923076923077038, 0.2153846153846153966, 0.2230769230769230893, 0.2307692307692307820, 0.2384615384615384748, 0.2461538461538461675, 0.2538461538461538325, 0.2615384615384615530, 0.2692307692307692180, 0.2769230769230769384, 0.2846153846153846034, 0.2923076923076923239, 0.2999999999999999889, 0.3076923076923077094, 0.3153846153846153744, 0.3230769230769230949, 0.3307692307692307598, 0.3384615384615384803, 0.3461538461538461453, 0.3538461538461538658, 0.3615384615384615308, 0.3692307692307692513, 0.3769230769230769162, 0.3846153846153846367, 0.3923076923076923017, 0.4000000000000000222, 0.4076923076923076872, 0.4153846153846154077, 0.4230769230769230727, 0.4307692307692307931, 0.4384615384615384581, 0.4461538461538461786, 0.4538461538461538436, 0.4615384615384615641, 0.4692307692307692291, 0.4769230769230769496, 0.4846153846153846145, 0.4923076923076923350, 0.5000000000000000000, 0.5076923076923076650, 0.5153846153846153300, 0.5230769230769231060, 0.5307692307692307709, 0.5384615384615384359, 0.5461538461538461009, 0.5538461538461538769, 0.5615384615384615419, 0.5692307692307692069, 0.5769230769230768718, 0.5846153846153846478, 0.5923076923076923128, 0.5999999999999999778, 0.6076923076923076428, 0.6153846153846154188, 0.6230769230769230838, 0.6307692307692307487, 0.6384615384615384137, 0.6461538461538461897, 0.6538461538461538547, 0.6615384615384615197, 0.6692307692307691847, 0.6769230769230769607, 0.6846153846153846256, 0.6923076923076922906, 0.6999999999999999556, 0.7076923076923077316, 0.7153846153846153966, 0.7230769230769230616, 0.7307692307692307265, 0.7384615384615385025, 0.7461538461538461675, 0.7538461538461538325, 0.7615384615384614975, 0.7692307692307692735, 0.7769230769230769384, 0.7846153846153846034, 0.7923076923076922684, 0.8000000000000000444, 0.8076923076923077094, 0.8153846153846153744, 0.8230769230769230393, 0.8307692307692308153, 0.8384615384615384803, 0.8461538461538461453, 0.8538461538461538103, 0.8615384615384615863, 0.8692307692307692513, 0.8769230769230769162, 0.8846153846153845812, 0.8923076923076923572, 0.9000000000000000222, 0.9076923076923076872, 0.9153846153846153522, 0.9230769230769231282, 0.9307692307692307931, 0.9384615384615384581, 0.9461538461538461231, 0.9538461538461538991, 0.9615384615384615641, 0.9692307692307692291, 0.9769230769230768940, 0.9846153846153846700, 0.9923076923076923350, 1.000000000000000000 ),
 .UNSPECIFIED. ) 
 CURVE ( )  GEOMETRIC_REPRESENTATION_ITEM ( )  RATIONAL_B_SPLINE_CURVE ( ( 1.000000000000000000, 0.9510565162951535312, 1.000000000000000000, 0.9510565162951535312, 1.000000000000000000, 0.9510565162951535312, 1.000000000000000000, 0.9510565162951535312, 1.000000000000000000, 0.9510565162951535312, 1.000000000000000000, 0.9510565162951535312, 1.000000000000000000, 0.9510565162951535312, 1.000000000000000000, 0.9510565162951535312, 1.000000000000000000, 0.9510565162951535312, 1.000000000000000000, 0.9510565162951535312, 1.000000000000000000, 0.9510565162951535312, 1.000000000000000000, 0.9510565162951535312, 1.000000000000000000, 0.9510565162951535312, 1.000000000000000000, 0.9510565162951535312, 1.000000000000000000, 0.9510565162951535312, 1.000000000000000000, 0.9510565162951535312, 1.000000000000000000, 0.9510565162951535312, 1.000000000000000000, 0.9510565162951535312, 1.000000000000000000, 0.9510565162951535312, 1.000000000000000000, 0.9510565162951535312, 1.000000000000000000, 0.9510565162951535312, 1.000000000000000000, 0.9510565162951535312, 1.000000000000000000, 0.9510565162951535312, 1.000000000000000000, 0.9510565162951535312, 1.000000000000000000, 0.9510565162951535312, 1.000000000000000000, 0.9510565162951535312, 1.000000000000000000, 0.9510565162951535312, 1.000000000000000000, 0.9510565162951535312, 1.000000000000000000, 0.9510565162951535312, 1.000000000000000000, 0.9510565162951535312, 1.000000000000000000, 0.9510565162951535312, 1.000000000000000000, 0.9510565162951535312, 1.000000000000000000, 0.9510565162951535312, 1.000000000000000000, 0.9510565162951535312, 1.000000000000000000, 0.9510565162951535312, 1.000000000000000000, 0.9510565162951535312, 1.000000000000000000, 0.9510565162951535312, 1.000000000000000000, 0.9510565162951535312, 1.000000000000000000, 0.9510565162951535312, 1.000000000000000000, 0.9510565162951535312, 1.000000000000000000, 0.9510565162951535312, 1.000000000000000000, 0.9510565162951535312, 1.000000000000000000, 0.9510565162951535312, 1.000000000000000000, 0.9510565162951535312, 1.000000000000000000, 0.9510565162951535312, 1.000000000000000000, 0.9510565162951535312, 1.000000000000000000, 0.9510565162951535312, 1.000000000000000000, 0.9510565162951535312, 1.000000000000000000, 0.9510565162951535312, 1.000000000000000000, 0.9510565162951535312, 1.000000000000000000, 0.9510565162951535312, 1.000000000000000000, 0.9510565162951535312, 1.000000000000000000, 0.9510565162951535312, 1.000000000000000000, 0.9510565162951535312, 1.000000000000000000, 0.9510565162951535312, 1.000000000000000000, 0.9510565162951535312, 1.000000000000000000, 0.9510565162951535312, 1.000000000000000000, 0.9510565162951535312, 1.000000000000000000, 0.9510565162951535312, 1.000000000000000000, 0.9510565162951535312, 1.000000000000000000, 0.9510565162951535312, 1.000000000000000000, 0.9510565162951535312, 1.000000000000000000, 0.9510565162951535312, 1.000000000000000000, 0.9510565162951535312, 1.000000000000000000, 0.9510565162951535312, 1.000000000000000000, 0.9510565162951535312, 1.000000000000000000, 0.9510565162951535312, 1.000000000000000000, 0.9510565162951535312, 1.000000000000000000, 0.9510565162951535312, 1.000000000000000000, 0.9510565162951535312, 1.000000000000000000, 0.9510565162951535312, 1.000000000000000000, 0.9510565162951535312, 1.000000000000000000, 0.9510565162951535312, 1.000000000000000000, 0.9510565162951535312, 1.000000000000000000, 0.9510565162951535312, 1.000000000000000000, 0.9510565162951535312, 1.000000000000000000, 0.9510565162951535312, 1.000000000000000000, 0.9510565162951535312, 1.000000000000000000, 0.9510565162951535312, 1.000000000000000000, 0.9510565162951535312, 1.000000000000000000, 0.9510565162951535312, 1.000000000000000000, 0.9510565162951535312, 1.000000000000000000, 0.9510565162951535312, 1.000000000000000000, 0.9510565162951535312, 1.000000000000000000, 0.9510565162951535312, 1.000000000000000000, 0.9510565162951535312, 1.000000000000000000, 0.9510565162951535312, 1.000000000000000000, 0.9510565162951535312, 1.000000000000000000, 0.9510565162951535312, 1.000000000000000000, 0.9510565162951535312, 1.000000000000000000, 0.9510565162951535312, 1.000000000000000000, 0.9510565162951535312, 1.000000000000000000, 0.9510565162951535312, 1.000000000000000000, 0.9510565162951535312, 1.000000000000000000, 0.9510565162951535312, 1.000000000000000000, 0.9510565162951535312, 1.000000000000000000, 0.9510565162951535312, 1.000000000000000000, 0.9510565162951535312, 1.000000000000000000, 0.9510565162951535312, 1.000000000000000000, 0.9510565162951535312, 1.000000000000000000, 0.9510565162951535312, 1.000000000000000000, 0.9510565162951535312, 1.000000000000000000, 0.9510565162951535312, 1.000000000000000000, 0.9510565162951535312, 1.000000000000000000, 0.9510565162951535312, 1.000000000000000000, 0.9510565162951535312, 1.000000000000000000, 0.9510565162951535312, 1.000000000000000000, 0.9510565162951535312, 1.000000000000000000, 0.9510565162951535312, 1.000000000000000000, 0.9510565162951535312, 1.000000000000000000, 0.9510565162951535312, 1.000000000000000000, 0.9510565162951535312, 1.000000000000000000, 0.9510565162951535312, 1.000000000000000000, 0.9510565162951535312, 1.000000000000000000, 0.9510565162951535312, 1.000000000000000000, 0.9510565162951535312, 1.000000000000000000, 0.9510565162951535312, 1.000000000000000000, 0.9510565162951535312, 1.000000000000000000, 0.9510565162951535312, 1.000000000000000000, 0.9510565162951535312, 1.000000000000000000, 0.9510565162951535312, 1.000000000000000000, 0.9510565162951535312, 1.000000000000000000, 0.9510565162951535312, 1.000000000000000000, 0.9510565162951535312, 1.000000000000000000, 0.9510565162951535312, 1.000000000000000000, 0.9510565162951535312, 1.000000000000000000, 0.9510565162951535312, 1.000000000000000000, 0.9510565162951535312, 1.000000000000000000, 0.9510565162951535312, 1.000000000000000000, 0.9510565162951535312, 1.000000000000000000 ) ) 
 REPRESENTATION_ITEM ( '' )  );
#2800=CARTESIAN_POINT ( 'NONE',  ( -2.823794231030041235, -68.59547149457073090, -1.017458915287723364 ) ) ;
#2802=CARTESIAN_POINT ( 'NONE',  ( 4.784657899331208775, -71.10452850542925773, 1.454677039711774533 ) ) ;
#2803=CARTESIAN_POINT ( 'NONE',  ( -2.369498399071057193, -78.34547149457074511, 6.969112962950058332 ) ) ;
#2806=CARTESIAN_POINT ( 'NONE',  ( -4.725907263620323207, -63.90452850542925489, 1.635492904037698647 ) ) ;
#2808=CARTESIAN_POINT ( 'NONE',  ( -4.312004677470993030, -75.04547149457074795, 3.009306630940933758 ) ) ;
#2810=CARTESIAN_POINT ( 'NONE',  ( 4.312004677471013459, -97.54547149457070532, -3.009306630940933314 ) ) ;
#2811=CARTESIAN_POINT ( 'NONE',  ( -4.191402346623180897, -63.30452850542926058, -5.607243785695311900 ) ) ;
#2814=CARTESIAN_POINT ( 'NONE',  ( -4.784657899331190123, -81.60452850542925773, -1.454677039711773867 ) ) ;
#2815=CARTESIAN_POINT ( 'NONE',  ( 7.360235569667875843, -62.25452850542926342, -0.09995255151731691212 ) ) ;
#2816=CARTESIAN_POINT ( 'NONE',  ( 3.154386672714808437, -73.24547149457075079, 0.09995255151720662534 ) ) ;
#2819=FACE_OUTER_BOUND ( 'NONE', #870, .T. ) ;
#2820=CARTESIAN_POINT ( 'NONE',  ( -4.194503406049316929, -76.05452850542926058, 3.171033256558100533 ) ) ;
#2823=CARTESIAN_POINT ( 'NONE',  ( 1.529537955723689890, -71.85452850542925773, -5.030887037049978971 ) ) ;
#2824=CARTESIAN_POINT ( 'NONE',  ( 0.09506052544077742139, -85.99547149457075079, -2.999999999999997780 ) ) ;
#2826=CARTESIAN_POINT ( 'NONE',  ( -5.257311121191321490, -95.74547149457072237, -0.09995255151718371311 ) ) ;
#2827=CARTESIAN_POINT ( 'NONE',  ( -1.529537955723670795, -73.35452850542922931, 5.030887037049979860 ) ) ;
#2828=CARTESIAN_POINT ( 'NONE',  ( -4.037591185471424815, -58.20452850542925916, 5.718994135553947977 ) ) ;
#2829=CARTESIAN_POINT ( 'NONE',  ( 7.360235569667880284, -92.25452850542926342, -0.09995255151731691212 ) ) ;
#2830=CARTESIAN_POINT ( 'NONE',  ( 1.840261337453269919, -67.80452850542926058, 2.371175808195547852 ) ) ;
#2835=CARTESIAN_POINT ( 'NONE',  ( -2.493201789345251829, -76.05452850542926058, 1.934965279058294518 ) ) ;
#2836=CARTESIAN_POINT ( 'NONE',  ( 4.191402346623198660, -91.80452850542926058, 5.607243785695311900 ) ) ;
#2837=CARTESIAN_POINT ( 'NONE',  ( 0.09506052544073614885, -91.99547149457075079, -6.999999999999997335 ) ) ;
#2840=AXIS2_PLACEMENT_3D ( 'NONE', #8120, #5497, #1756 ) ;
#2841=CARTESIAN_POINT ( 'NONE',  ( 2.610703060766943029, -64.54547149457073374, -1.773238653441125523 ) ) ;
#2845=CARTESIAN_POINT ( 'NONE',  ( -1.529537955723671683, -64.35452850542924352, 5.030887037049979860 ) ) ;
#2846=CARTESIAN_POINT ( 'NONE',  ( -4.037591185471543831, -83.29547149457074795, -5.718994135553860936 ) ) ;
#2848=CARTESIAN_POINT ( 'NONE',  ( 1.719659006605285478, -73.84547149457074511, -4.969112962950050338 ) ) ;
#2849=CARTESIAN_POINT ( 'NONE',  ( -4.194503406049319594, -70.05452850542923215, 3.171033256558100533 ) ) ;
#2851=CARTESIAN_POINT ( 'NONE',  ( -1.529537955723777820, -71.14547149457071384, -5.030887037049945221 ) ) ;
#2853=CARTESIAN_POINT ( 'NONE',  ( -5.257311121191321490, -95.74547149457072237, -0.09995255151718371311 ) ) ;
#2854=CARTESIAN_POINT ( 'NONE',  ( 6.628020296210639373, -59.40452850542925489, -2.253526892787612645 ) ) ;
#2857=CARTESIAN_POINT ( 'NONE',  ( 2.862020680886514956, -80.70452850542925205, -4.100960146804039752 ) ) ;
#2860=CARTESIAN_POINT ( 'NONE',  ( -0.09506052544083884448, -87.00452850542924921, -4.999999999999997335 ) ) ;
#2861=CARTESIAN_POINT ( 'NONE',  ( -0.09506052544083960776, -81.00452850542926342, -4.999999999999997335 ) ) ;
#2863=CARTESIAN_POINT ( 'NONE',  ( -3.015831842038215083, -75.30452850542926058, -3.989209796945429432 ) ) ;
#2864=CARTESIAN_POINT ( 'NONE',  ( -2.823794231030039903, -80.59547149457075932, -1.017458915287723364 ) ) ;
#2865=CARTESIAN_POINT ( 'NONE',  ( -2.823794231030042567, -59.59547149457074511, -1.017458915287723364 ) ) ;
#2866=CARTESIAN_POINT ( 'NONE',  ( 5.257311121191341918, -74.25452850542924921, -0.09995255151729465215 ) ) ;
#2867=CARTESIAN_POINT ( 'NONE',  ( -6.628020296210620721, -84.90452850542926910, 2.253526892787613978 ) ) ;
#2868=CARTESIAN_POINT ( 'NONE',  ( -1.069819614139540409, -60.15452850542926200, -2.969112962950023249 ) ) ;
#2869=AXIS2_PLACEMENT_3D ( 'NONE', #4595, #7771, #2126 ) ;
#2873=CARTESIAN_POINT ( 'NONE',  ( -1.069819614139537967, -81.15452850542924068, -2.969112962950023249 ) ) ;
#2874=CARTESIAN_POINT ( 'NONE',  ( -2.179377348189460051, -85.35452850542924352, 7.030887037049988741 ) ) ;
#2875=CARTESIAN_POINT ( 'NONE',  ( 4.037591185471562483, -78.79547149457074795, 5.718994135553860936 ) ) ;
#2878=CARTESIAN_POINT ( 'NONE',  ( -2.823794231030020363, -81.90452850542925489, 1.017458915287783316 ) ) ;
#2883=CARTESIAN_POINT ( 'NONE',  ( -4.784657899331191899, -63.60452850542925063, -1.454677039711773867 ) ) ;
#2884=CARTESIAN_POINT ( 'NONE',  ( 7.360235569667878508, -82.24547149457073658, 0.09995255151716216091 ) ) ;
#2886=CARTESIAN_POINT ( 'NONE',  ( -0.09506052544073541333, -75.49547149457073658, 4.999999999999997335 ) ) ;
#2887=CARTESIAN_POINT ( 'NONE',  ( 3.015831842038148025, -70.69547149457073942, -3.989209796945492048 ) ) ;
#2889=CARTESIAN_POINT ( 'NONE',  ( 4.725907263620340082, -65.40452850542925489, -1.635492904037697981 ) ) ;
#2893=CARTESIAN_POINT ( 'NONE',  ( -2.862020680886581570, -68.29547149457074795, -4.100960146803977580 ) ) ;
#2895=CARTESIAN_POINT ( 'NONE',  ( -6.013306294175153610, -63.45452850542924494, -4.245374608440613429 ) ) ;
#2901=CARTESIAN_POINT ( 'NONE',  ( 2.862020680886515844, -89.70452850542926626, -4.100960146804039752 ) ) ;
#2902=CARTESIAN_POINT ( 'NONE',  ( 4.784657899331210551, -83.10452850542927195, 1.454677039711774533 ) ) ;
#2904=CARTESIAN_POINT ( 'NONE',  ( 0.09506052544085895339, -67.50452850542926342, 4.999999999999997335 ) ) ;
#2905=CARTESIAN_POINT ( 'NONE',  ( -1.069819614139473796, -84.34547149457075932, 2.969112962950044121 ) ) ;
#2906=CARTESIAN_POINT ( 'NONE',  ( 4.725907263620374721, -94.09547149457074511, 1.635492904037598283 ) ) ;
#2907=CARTESIAN_POINT ( 'NONE',  ( -4.725907263620321430, -72.90452850542925489, 1.635492904037698647 ) ) ;
#2908=CARTESIAN_POINT ( 'NONE',  ( -4.037591185471422150, -85.20452850542925205, 5.718994135553947977 ) ) ;
#2909=CARTESIAN_POINT ( 'NONE',  ( -2.823794231030023472, -57.90452850542925489, 1.017458915287783316 ) ) ;
#2913=CARTESIAN_POINT ( 'NONE',  ( -1.840261337453252821, -69.30452850542926058, -2.371175808195547852 ) ) ;
#2914=CARTESIAN_POINT ( 'NONE',  ( 2.369498399071225503, -79.65452850542925489, 6.969112962950009482 ) ) ;
#2915=CARTESIAN_POINT ( 'NONE',  ( 6.628020296210687334, -79.09547149457075932, 2.253526892787472757 ) ) ;
#2917=CARTESIAN_POINT ( 'NONE',  ( -1.719659006605263718, -93.34547149457073090, 4.969112962950051227 ) ) ;
#2918=CARTESIAN_POINT ( 'NONE',  ( -1.069819614139537522, -84.15452850542925489, -2.969112962950023249 ) ) ;
#2924=CARTESIAN_POINT ( 'NONE',  ( 4.784657899331207886, -62.10452850542925063, 1.454677039711774533 ) ) ;
#2925=CARTESIAN_POINT ( 'NONE',  ( 4.037591185471562483, -78.79547149457074795, 5.718994135553860936 ) ) ;
#2926=ORIENTED_EDGE ( 'NONE', *, *, #3884, .F. ) ;
#2927=CARTESIAN_POINT ( 'NONE',  ( -1.719659006605266383, -72.34547149457073090, 4.969112962950051227 ) ) ;
#2928=CARTESIAN_POINT ( 'NONE',  ( -4.194503406049384431, -71.44547149457075363, -3.171033256558012159 ) ) ;
#2929=CARTESIAN_POINT ( 'NONE',  ( 2.862020680886512292, -62.70452850542926626, -4.100960146804039752 ) ) ;
#2931=CARTESIAN_POINT ( 'NONE',  ( 4.784657899331176800, -67.39547149457074227, -1.454677039711874009 ) ) ;
#2934=CARTESIAN_POINT ( 'NONE',  ( -7.360235569667860744, -63.75452850542926342, 0.09995255151731782806 ) ) ;
#2939=CARTESIAN_POINT ( 'NONE',  ( 4.784657899331210551, -83.10452850542927195, 1.454677039711774533 ) ) ;
#2940=CARTESIAN_POINT ( 'NONE',  ( 5.257311121191341918, -74.25452850542924921, -0.09995255151729465215 ) ) ;
#2941=CARTESIAN_POINT ( 'NONE',  ( 4.725907263620340082, -74.40452850542925489, -1.635492904037697981 ) ) ;
#2942=CARTESIAN_POINT ( 'NONE',  ( -2.610703060766925709, -81.04547149457074795, 1.773238653441125745 ) ) ;
#2943=CARTESIAN_POINT ( 'NONE',  ( -0.09506052544073276267, -96.49547149457075079, 4.999999999999997335 ) ) ;
#2944=CARTESIAN_POINT ( 'NONE',  ( -0.09506052544084110656, -69.00452850542926342, -4.999999999999997335 ) ) ;
#2945=CARTESIAN_POINT ( 'NONE',  ( -4.191402346623177344, -87.30452850542926058, -5.607243785695311900 ) ) ;
#2946=CARTESIAN_POINT ( 'NONE',  ( -1.686450176301568016, -58.20452850542925916, 2.482926158054133303 ) ) ;
#2953=CARTESIAN_POINT ( 'NONE',  ( -2.823794231030022139, -69.90452850542925489, 1.017458915287783316 ) ) ;
#2955=CARTESIAN_POINT ( 'NONE',  ( -4.191402346623058328, -78.19547149457073942, 5.607243785695398941 ) ) ;
#2958=CARTESIAN_POINT ( 'NONE',  ( 4.302742873392585210, -96.99999999999947420, 2.548615363087012753 ) ) ;
#2959=CARTESIAN_POINT ( 'NONE',  ( -1.840261337453250823, -84.30452850542926058, -2.371175808195547852 ) ) ;
#2964=CARTESIAN_POINT ( 'NONE',  ( 2.862020680886511848, -59.70452850542925205, -4.100960146804039752 ) ) ;
#2965=CARTESIAN_POINT ( 'NONE',  ( 5.895805022753492608, -72.94547149457073942, 4.407101234057782868 ) ) ;
#2967=CARTESIAN_POINT ( 'NONE',  ( -4.194503406049383543, -71.44547149457073942, -3.171033256558012159 ) ) ;
#2968=CARTESIAN_POINT ( 'NONE',  ( -1.719659006605265716, -72.34547149457071669, 4.969112962950051227 ) ) ;
#2969=CARTESIAN_POINT ( 'NONE',  ( 1.529537955723688780, -62.85452850542925063, -5.030887037049978971 ) ) ;
#2971=CARTESIAN_POINT ( 'NONE',  ( 4.194503406049400418, -60.94547149457072521, 3.171033256558012159 ) ) ;
#2973=CARTESIAN_POINT ( 'NONE',  ( 3.015831842038236399, -94.80452850542924637, 3.989209796945429432 ) ) ;
#2979=CARTESIAN_POINT ( 'NONE',  ( 1.719659006605391616, -82.65452850542925489, 4.969112962950016588 ) ) ;
#2980=CARTESIAN_POINT ( 'NONE',  ( -4.725907263620351628, -92.59547149457074511, -1.635492904037597617 ) ) ;
#2981=CARTESIAN_POINT ( 'NONE',  ( -4.312004677471058756, -63.45452850542926626, -3.009306630940843608 ) ) ;
#2982=CARTESIAN_POINT ( 'NONE',  ( 1.686450176301636850, -84.79547149457074795, 2.482926158054096000 ) ) ;
#2983=CARTESIAN_POINT ( 'NONE',  ( 4.725907263620375609, -97.09547149457074511, 1.635492904037598283 ) ) ;
#2984=CARTESIAN_POINT ( 'NONE',  ( -1.529537955723671683, -67.35452850542925773, 5.030887037049979860 ) ) ;
#2985=CARTESIAN_POINT ( 'NONE',  ( 5.895805022753406455, -83.55452850542926058, -4.407101234057908989 ) ) ;
#2986=CARTESIAN_POINT ( 'NONE',  ( 2.823794231030062551, -97.09547149457074511, 1.017458915287723809 ) ) ;
#2991=CARTESIAN_POINT ( 'NONE',  ( -2.862020680886492752, -88.20452850542925205, 4.100960146804039752 ) ) ;
#2992=CARTESIAN_POINT ( 'NONE',  ( 2.823794231030039015, -65.40452850542925489, -1.017458915287783316 ) ) ;
#2993=CARTESIAN_POINT ( 'NONE',  ( -0.09506052544071416643, -75.49547149457075079, 6.999999999999997335 ) ) ;
#2996=CARTESIAN_POINT ( 'NONE',  ( 0.09506052544075714594, -91.99547149457073658, -4.999999999999997335 ) ) ;
#2997=CARTESIAN_POINT ( 'NONE',  ( 1.069819614139557729, -82.65452850542926910, 2.969112962950023249 ) ) ;
#3001=CARTESIAN_POINT ( 'NONE',  ( 4.312004677471073855, -61.95452850542923784, 3.009306630940844496 ) ) ;
#3002=CARTESIAN_POINT ( 'NONE',  ( -2.369498399071057637, -75.34547149457073090, 6.969112962950058332 ) ) ;
#3003=CARTESIAN_POINT ( 'NONE',  ( 4.331153185401124261, -96.99999999999995737, 2.564721935162156630 ) ) ;
#3005=CARTESIAN_POINT ( 'NONE',  ( 4.725907263620372945, -79.09547149457074511, 1.635492904037598283 ) ) ;
#3006=CARTESIAN_POINT ( 'NONE',  ( 2.862020680886599333, -72.79547149457074795, 4.100960146803977580 ) ) ;
#3007=CARTESIAN_POINT ( 'NONE',  ( 5.257311121191341918, -59.25452850542924210, -0.09995255151729465215 ) ) ;
#3010=CARTESIAN_POINT ( 'NONE',  ( 1.719659006605389617, -67.65452850542925489, 4.969112962950016588 ) ) ;
#3012=CARTESIAN_POINT ( 'NONE',  ( 0.09506052544075374588, -64.99547149457075079, -4.999999999999997335 ) ) ;
#3013=CARTESIAN_POINT ( 'NONE',  ( 1.529537955723692555, -92.85452850542925773, -5.030887037049978971 ) ) ;
#3021=CARTESIAN_POINT ( 'NONE',  ( 4.784657899331211439, -89.10452850542925773, 1.454677039711774533 ) ) ;
#3022=CARTESIAN_POINT ( 'NONE',  ( -0.09506052544073390065, -87.49547149457075079, 4.999999999999997335 ) ) ;
#3023=CARTESIAN_POINT ( 'NONE',  ( -5.257311121191325043, -60.75452850542925631, 0.09995255151729529053 ) ) ;
#3024=CARTESIAN_POINT ( 'NONE',  ( -1.840261337453200197, -78.19547149457073942, 2.371175808195584267 ) ) ;
#3025=CARTESIAN_POINT ( 'NONE',  ( 1.719659006605286811, -88.84547149457070248, -4.969112962950050338 ) ) ;
#3026=CARTESIAN_POINT ( 'NONE',  ( 5.257311121191341918, -65.25452850542926342, -0.09995255151729465215 ) ) ;
#3027=CARTESIAN_POINT ( 'NONE',  ( -0.09506052544086102118, -78.00452850542926342, -6.999999999999997335 ) ) ;
#3028=CARTESIAN_POINT ( 'NONE',  ( -1.069819614139541075, -57.15452850542926200, -2.969112962950023249 ) ) ;
#3033=CARTESIAN_POINT ( 'NONE',  ( 1.529537955723692555, -92.85452850542925773, -5.030887037049978971 ) ) ;
#3034=CARTESIAN_POINT ( 'NONE',  ( 1.069819614139555952, -67.65452850542925489, 2.969112962950023249 ) ) ;
#3035=CARTESIAN_POINT ( 'NONE',  ( 4.725907263620342746, -95.40452850542925489, -1.635492904037697981 ) ) ;
#3036=CARTESIAN_POINT ( 'NONE',  ( 4.191402346623078756, -79.69547149457075363, -5.607243785695398941 ) ) ;
#3037=CARTESIAN_POINT ( 'NONE',  ( 1.529537955723692999, -95.85452850542922931, -5.030887037049978971 ) ) ;
#3039=CARTESIAN_POINT ( 'NONE',  ( -2.862020680886579793, -83.29547149457074795, -4.100960146803977580 ) ) ;
#3040=CARTESIAN_POINT ( 'NONE',  ( 1.840261337453271917, -85.80452850542926058, 2.371175808195547852 ) ) ;
#3045=CARTESIAN_POINT ( 'NONE',  ( 2.862020680886512292, -62.70452850542926626, -4.100960146804039752 ) ) ;
#3046=CARTESIAN_POINT ( 'NONE',  ( -4.037591185471544719, -74.29547149457074795, -5.718994135553860936 ) ) ;
#3049=CARTESIAN_POINT ( 'NONE',  ( 4.725907263620372056, -70.09547149457074511, 1.635492904037598283 ) ) ;
#3050=CARTESIAN_POINT ( 'NONE',  ( 2.862020680886598889, -69.79547149457074795, 4.100960146803977580 ) ) ;
#3051=CARTESIAN_POINT ( 'NONE',  ( 0.09506052544085781542, -58.50452850542925631, 4.999999999999997335 ) ) ;
#3053=CARTESIAN_POINT ( 'NONE',  ( -4.312004677471058756, -66.45452850542925205, -3.009306630940844052 ) ) ;
#3054=CARTESIAN_POINT ( 'NONE',  ( -4.784657899331159925, -62.89547149457074227, 1.454677039711874675 ) ) ;
#3061=CARTESIAN_POINT ( 'NONE',  ( -5.257311121191324155, -75.75452850542922079, 0.09995255151729526277 ) ) ;
#3062=CARTESIAN_POINT ( 'NONE',  ( 0.09506052544075714594, -91.99547149457073658, -4.999999999999997335 ) ) ;
#3063=CARTESIAN_POINT ( 'NONE',  ( 4.725907263620340082, -65.40452850542925489, -1.635492904037697981 ) ) ;
#3064=CARTESIAN_POINT ( 'NONE',  ( 1.686450176301635961, -75.79547149457074795, 2.482926158054096000 ) ) ;
#3065=CARTESIAN_POINT ( 'NONE',  ( -7.360235569667858080, -81.75452850542926342, 0.09995255151731782806 ) ) ;
#3066=CARTESIAN_POINT ( 'NONE',  ( -4.312004677470992142, -87.04547149457074795, 3.009306630940933758 ) ) ;
#3067=CARTESIAN_POINT ( 'NONE',  ( -3.015831842038215971, -69.30452850542926058, -3.989209796945429432 ) ) ;
#3068=CARTESIAN_POINT ( 'NONE',  ( -0.09506052544086064648, -81.00452850542926342, -6.999999999999997335 ) ) ;
#3069=CARTESIAN_POINT ( 'NONE',  ( 3.154386672714811102, -91.24547149457073658, 0.09995255151720662534 ) ) ;
#3073=CARTESIAN_POINT ( 'NONE',  ( -0.09506052544073731458, -60.49547149457074369, 4.999999999999997335 ) ) ;
#3075=CARTESIAN_POINT ( 'NONE',  ( -4.194503406049316041, -88.05452850542924637, 3.171033256558101865 ) ) ;
#3076=CARTESIAN_POINT ( 'NONE',  ( -1.069819614139539521, -66.15452850542925489, -2.969112962950023249 ) ) ;
#3077=CARTESIAN_POINT ( 'NONE',  ( -2.369498399071207739, -57.15452850542926200, -6.969112962950009482 ) ) ;
#3078=CARTESIAN_POINT ( 'NONE',  ( -0.09506052544071491583, -69.49547149457075079, 6.999999999999997335 ) ) ;
#3080=CARTESIAN_POINT ( 'NONE',  ( 5.257311121191342806, -82.24547149457073658, 0.09995255151718437925 ) ) ;
#3081=CARTESIAN_POINT ( 'NONE',  ( -2.882544866740877065, -78.60452850542927195, -0.8366430509618996147 ) ) ;
#3084=CARTESIAN_POINT ( 'NONE',  ( -5.257311121191324155, -57.75452850542923500, 0.09995255151729526277 ) ) ;
#3087=CARTESIAN_POINT ( 'NONE',  ( -5.895805022753477509, -74.44547149457072521, -4.407101234057782868 ) ) ;
#3089=CARTESIAN_POINT ( 'NONE',  ( 4.919969012183922352, -96.99999999999991473, -3.234920223772670411 ) ) ;
#3090=CARTESIAN_POINT ( 'NONE',  ( 5.257311121191341030, -64.24547149457075079, 0.09995255151718437925 ) ) ;
#3091=CARTESIAN_POINT ( 'NONE',  ( 4.037591185471564259, -93.79547149457076216, 5.718994135553860936 ) ) ;
#3092=CARTESIAN_POINT ( 'NONE',  ( 2.823794231030042567, -92.40452850542925489, -1.017458915287783316 ) ) ;
#3096=CARTESIAN_POINT ( 'NONE',  ( 4.312004677471073855, -64.95452850542926626, 3.009306630940844496 ) ) ;
#3098=CARTESIAN_POINT ( 'NONE',  ( 6.013306294175080779, -97.54547149457074795, -4.245374608440741326 ) ) ;
#3105=CARTESIAN_POINT ( 'NONE',  ( -1.529537955723670350, -76.35452850542925773, 5.030887037049979860 ) ) ;
#3106=CARTESIAN_POINT ( 'NONE',  ( 3.015831842038150690, -91.69547149457073942, -3.989209796945492048 ) ) ;
#3108=CARTESIAN_POINT ( 'NONE',  ( 4.194503406049336469, -65.55452850542924637, -3.171033256558100977 ) ) ;
#3109=CARTESIAN_POINT ( 'NONE',  ( -1.840261337453200641, -75.19547149457073942, 2.371175808195584267 ) ) ;
#3110=CARTESIAN_POINT ( 'NONE',  ( -0.09506052544086064648, -81.00452850542926342, -6.999999999999997335 ) ) ;
#3111=CARTESIAN_POINT ( 'NONE',  ( 4.725907263620374721, -91.09547149457074511, 1.635492904037598283 ) ) ;
#3112=CARTESIAN_POINT ( 'NONE',  ( 2.862020680886512292, -62.70452850542926626, -4.100960146804039752 ) ) ;
#3113=CARTESIAN_POINT ( 'NONE',  ( 0.09506052544088100520, -73.50452850542924921, 6.999999999999997335 ) ) ;
#3114=CARTESIAN_POINT ( 'NONE',  ( -1.069819614139473796, -84.34547149457075932, 2.969112962950044121 ) ) ;
#3117=CARTESIAN_POINT ( 'NONE',  ( 0.09506052544075298261, -58.99547149457073658, -4.999999999999997335 ) ) ;
#3119=CARTESIAN_POINT ( 'NONE',  ( -4.725907263620318766, -93.90452850542925489, 1.635492904037698647 ) ) ;
#3120=CARTESIAN_POINT ( 'NONE',  ( -1.840261337453253487, -63.30452850542926058, -2.371175808195547852 ) ) ;
#3121=CARTESIAN_POINT ( 'NONE',  ( 0.09506052544087949252, -61.50452850542925631, 6.999999999999997335 ) ) ;
#3122=CARTESIAN_POINT ( 'NONE',  ( 2.179377348189628361, -69.64547149457072805, 7.030887037049939003 ) ) ;
#3123=CARTESIAN_POINT ( 'NONE',  ( 0.09506052544075639654, -85.99547149457075079, -4.999999999999997335 ) ) ;
#3124=CARTESIAN_POINT ( 'NONE',  ( -2.493201789345251829, -79.05452850542926058, 1.934965279058294518 ) ) ;
#3128=CARTESIAN_POINT ( 'NONE',  ( -2.882544866740875733, -87.60452850542924352, -0.8366430509618996147 ) ) ;
#3129=CARTESIAN_POINT ( 'NONE',  ( -4.191402346623060104, -66.19547149457073942, 5.607243785695398941 ) ) ;
#3132=CARTESIAN_POINT ( 'NONE',  ( -4.784657899331159925, -62.89547149457074227, 1.454677039711874675 ) ) ;
#3133=CARTESIAN_POINT ( 'NONE',  ( -4.037591185471542055, -95.29547149457076216, -5.718994135553860936 ) ) ;
#3134=CARTESIAN_POINT ( 'NONE',  ( 2.882544866740898826, -95.10452850542925773, 0.8366430509618999478 ) ) ;
#3136=CARTESIAN_POINT ( 'NONE',  ( -2.862020680886494972, -73.20452850542925205, 4.100960146804039752 ) ) ;
#3137=CARTESIAN_POINT ( 'NONE',  ( 4.194503406049400418, -63.94547149457075363, 3.171033256558012159 ) ) ;
#3145=CARTESIAN_POINT ( 'NONE',  ( -0.09506052544084034328, -75.00452850542924921, -4.999999999999997335 ) ) ;
#3147=CARTESIAN_POINT ( 'NONE',  ( -4.312004677470992142, -87.04547149457074795, 3.009306630940933758 ) ) ;
#3149=CARTESIAN_POINT ( 'NONE',  ( 4.387866329943309829, -96.99999999999997158, 0.7004174865519436910 ) ) ;
#3150=CARTESIAN_POINT ( 'NONE',  ( 1.069819614139493114, -67.84547149457071669, -2.969112962950042789 ) ) ;
#3151=CARTESIAN_POINT ( 'NONE',  ( 4.191402346623198660, -79.80452850542926058, 5.607243785695311900 ) ) ;
#3152=CARTESIAN_POINT ( 'NONE',  ( -4.194503406049383543, -86.44547149457071100, -3.171033256558012159 ) ) ;
#3154=CARTESIAN_POINT ( 'NONE',  ( 0.09506052544088137990, -76.50452850542926342, 6.999999999999997335 ) ) ;
#3157=CARTESIAN_POINT ( 'NONE',  ( 2.610703060766946138, -85.54547149457074795, -1.773238653441125523 ) ) ;
#3163=CARTESIAN_POINT ( 'NONE',  ( 1.719659006605392504, -88.65452850542926910, 4.969112962950015699 ) ) ;
#3164=CARTESIAN_POINT ( 'NONE',  ( -1.069819614139541075, -57.15452850542926200, -2.969112962950023249 ) ) ;
#3165=CARTESIAN_POINT ( 'NONE',  ( 4.194503406049340022, -95.55452850542921794, -3.171033256558100089 ) ) ;
#3166=CARTESIAN_POINT ( 'NONE',  ( -6.628020296210668683, -65.59547149457073090, -2.253526892787471869 ) ) ;
#3167=CARTESIAN_POINT ( 'NONE',  ( 4.194503406049403083, -87.94547149457071100, 3.171033256558012159 ) ) ;
#3168=CARTESIAN_POINT ( 'NONE',  ( -1.069819614139538855, -72.15452850542922647, -2.969112962950023249 ) ) ;
#3170=FILL_AREA_STYLE ('',( #6956 ) ) ;
#3171=CARTESIAN_POINT ( 'NONE',  ( -0.09506052544081743105, -90.00452850542926342, -2.999999999999997780 ) ) ;
#3172=CARTESIAN_POINT ( 'NONE',  ( -4.191402346623060104, -60.19547149457074653, 5.607243785695398941 ) ) ;
#3173=CARTESIAN_POINT ( 'NONE',  ( 5.461398254538926800, -97.00000000000000000, -2.077050515704315536 ) ) ;
#3174=CARTESIAN_POINT ( 'NONE',  ( 2.862020680886597557, -60.79547149457074084, 4.100960146803977580 ) ) ;
#3175=CARTESIAN_POINT ( 'NONE',  ( 0.09506052544075298261, -58.99547149457073658, -4.999999999999997335 ) ) ;
#3176=CARTESIAN_POINT ( 'NONE',  ( 3.154386672714811102, -92.25452850542926342, -0.09995255151727241993 ) ) ;
#3179=CARTESIAN_POINT ( 'NONE',  ( 3.015831842038233290, -70.80452850542926058, 3.989209796945429432 ) ) ;
#3181=CARTESIAN_POINT ( 'NONE',  ( -4.037591185471542943, -89.29547149457074795, -5.718994135553860936 ) ) ;
#3188=CARTESIAN_POINT ( 'NONE',  ( 5.257311121191341918, -77.25452850542926342, -0.09995255151729465215 ) ) ;
#3189=CARTESIAN_POINT ( 'NONE',  ( -1.719659006605265272, -75.34547149457074511, 4.969112962950051227 ) ) ;
#3191=CARTESIAN_POINT ( 'NONE',  ( 1.686450176301635295, -69.79547149457074795, 2.482926158054096000 ) ) ;
#3192=CARTESIAN_POINT ( 'NONE',  ( 2.369498399071225059, -76.65452850542925489, 6.969112962950009482 ) ) ;
#3193=CARTESIAN_POINT ( 'NONE',  ( 2.862020680886600221, -84.79547149457074795, 4.100960146803977580 ) ) ;
#3196=CARTESIAN_POINT ( 'NONE',  ( 6.628020296210642037, -80.40452850542925489, -2.253526892787612645 ) ) ;
#3197=CARTESIAN_POINT ( 'NONE',  ( -2.610703060766925265, -84.04547149457074795, 1.773238653441125745 ) ) ;
#3202=CARTESIAN_POINT ( 'NONE',  ( -4.784657899331190123, -78.60452850542925773, -1.454677039711773867 ) ) ;
#3203=CARTESIAN_POINT ( 'NONE',  ( 0.8796985632579643610, -96.64547149457075648, 3.030887037049952326 ) ) ;
#3205=CARTESIAN_POINT ( 'NONE',  ( -2.369498399071207739, -60.15452850542926200, -6.969112962950009482 ) ) ;
#3207=CARTESIAN_POINT ( 'NONE',  ( 4.037591185471561595, -72.79547149457074795, 5.718994135553860936 ) ) ;
#3208=CARTESIAN_POINT ( 'NONE',  ( -1.529537955723776044, -86.14547149457074227, -5.030887037049945221 ) ) ;
#3209=CARTESIAN_POINT ( 'NONE',  ( 2.823794231030039903, -74.40452850542925489, -1.017458915287783316 ) ) ;
#3212=CARTESIAN_POINT ( 'NONE',  ( -1.069819614139536412, -90.15452850542926910, -2.969112962950023249 ) ) ;
#3213=CARTESIAN_POINT ( 'NONE',  ( -6.628020296210668683, -62.59547149457074511, -2.253526892787471869 ) ) ;
#3216=CARTESIAN_POINT ( 'NONE',  ( -4.194503406049383543, -65.44547149457073942, -3.171033256558012159 ) ) ;
#3217=CARTESIAN_POINT ( 'NONE',  ( -4.725907263620355181, -62.59547149457074511, -1.635492904037597617 ) ) ;
#3222=CARTESIAN_POINT ( 'NONE',  ( -1.719659006605374074, -63.15452850542925489, -4.969112962950016588 ) ) ;
#3223=CARTESIAN_POINT ( 'NONE',  ( 6.013306294175080779, -91.54547149457074795, -4.245374608440741326 ) ) ;
#3225=CARTESIAN_POINT ( 'NONE',  ( 4.312004677471075631, -76.95452850542923784, 3.009306630940844496 ) ) ;
#3230=CARTESIAN_POINT ( 'NONE',  ( -4.194503406049384431, -80.44547149457073942, -3.171033256558012159 ) ) ;
#3231=CARTESIAN_POINT ( 'NONE',  ( 4.353213783654983793, -96.99999999999998579, 0.1443106696900772756 ) ) ;
#3232=CARTESIAN_POINT ( 'NONE',  ( 2.823794231030059443, -73.09547149457071669, 1.017458915287723809 ) ) ;
#3233=CARTESIAN_POINT ( 'NONE',  ( 4.191402346623197772, -73.80452850542926058, 5.607243785695311900 ) ) ;
#3235=CARTESIAN_POINT ( 'NONE',  ( -4.784657899331157260, -80.89547149457074227, 1.454677039711874675 ) ) ;
#3236=CARTESIAN_POINT ( 'NONE',  ( -1.529537955723671905, -61.35452850542925773, 5.030887037049979860 ) ) ;
#3238=CARTESIAN_POINT ( 'NONE',  ( 0.09506052544088061662, -70.50452850542926342, 6.999999999999997335 ) ) ;
#3239=CARTESIAN_POINT ( 'NONE',  ( -2.610703060766924821, -87.04547149457074795, 1.773238653441125745 ) ) ;
#3244=CARTESIAN_POINT ( 'NONE',  ( -3.015831842038213750, -90.30452850542926058, -3.989209796945429432 ) ) ;
#3246=CARTESIAN_POINT ( 'NONE',  ( 5.257311121191342806, -83.25452850542926342, -0.09995255151729466603 ) ) ;
#3247=CARTESIAN_POINT ( 'NONE',  ( -3.154386672714792006, -57.75452850542924921, 0.09995255151727280851 ) ) ;
#3249=CARTESIAN_POINT ( 'NONE',  ( -4.194503406049315153, -88.05452850542921794, 3.171033256558100533 ) ) ;
#3250=CARTESIAN_POINT ( 'NONE',  ( -4.037591185471544719, -74.29547149457074795, -5.718994135553860936 ) ) ;
#3251=CARTESIAN_POINT ( 'NONE',  ( 1.719659006605286145, -79.84547149457073090, -4.969112962950050338 ) ) ;
#3252=CARTESIAN_POINT ( 'NONE',  ( 1.686450176301584669, -71.70452850542925205, -2.482926158054133303 ) ) ;
#3256=CARTESIAN_POINT ( 'NONE',  ( -0.8796985632578778747, -88.35452850542924352, 3.030887037049973198 ) ) ;
#3257=CARTESIAN_POINT ( 'NONE',  ( -4.037591185471546495, -62.29547149457074084, -5.718994135553860936 ) ) ;
#3259=CARTESIAN_POINT ( 'NONE',  ( -4.312004677471057867, -72.45452850542922363, -3.009306630940844052 ) ) ;
#3260=CARTESIAN_POINT ( 'NONE',  ( -6.013306294175056799, -96.04547149457074795, 4.245374608440741326 ) ) ;
#3263=CARTESIAN_POINT ( 'NONE',  ( 4.784657899331207886, -62.10452850542925063, 1.454677039711774533 ) ) ;
#3264=CARTESIAN_POINT ( 'NONE',  ( 6.686770931921479644, -91.39547149457074227, -2.072711028461788896 ) ) ;
#3267=CARTESIAN_POINT ( 'NONE',  ( 2.862020680886513624, -71.70452850542925205, -4.100960146804039752 ) ) ;
#3273=CARTESIAN_POINT ( 'NONE',  ( -2.862020680886580681, -77.29547149457074795, -4.100960146803977580 ) ) ;
#3274=CARTESIAN_POINT ( 'NONE',  ( 4.226755616500139645, -97.00000000000000000, 2.333567455633055676 ) ) ;
#3275=CARTESIAN_POINT ( 'NONE',  ( 2.823794231030058111, -64.09547149457071669, 1.017458915287723809 ) ) ;
#3276=CARTESIAN_POINT ( 'NONE',  ( -4.037591185471423927, -67.20452850542925205, 5.718994135553947977 ) ) ;
#3278=CARTESIAN_POINT ( 'NONE',  ( -4.784657899331158148, -77.89547149457074227, 1.454677039711874675 ) ) ;
#3279=CARTESIAN_POINT ( 'NONE',  ( -4.784657899331192787, -57.60452850542925773, -1.454677039711773867 ) ) ;
#3280=CARTESIAN_POINT ( 'NONE',  ( 3.015831842038234623, -82.80452850542926058, 3.989209796945429432 ) ) ;
#3281=CARTESIAN_POINT ( 'NONE',  ( -4.037591185471424815, -64.20452850542925205, 5.718994135553947977 ) ) ;
#3282=CARTESIAN_POINT ( 'NONE',  ( -1.686450176301616644, -80.29547149457074795, -2.482926158054096000 ) ) ;
#3287=CARTESIAN_POINT ( 'NONE',  ( 4.312004677471078296, -91.95452850542925205, 3.009306630940844496 ) ) ;
#3288=CARTESIAN_POINT ( 'NONE',  ( 4.784657899331211439, -92.10452850542925773, 1.454677039711774533 ) ) ;
#3290=CARTESIAN_POINT ( 'NONE',  ( -5.257311121191323267, -81.75452850542926342, 0.09995255151729529053 ) ) ;
#3291=CARTESIAN_POINT ( 'NONE',  ( -3.154386672714787565, -95.74547149457073658, -0.09995255151720625064 ) ) ;
#3293=CARTESIAN_POINT ( 'NONE',  ( -2.862020680886493196, -85.20452850542925205, 4.100960146804039752 ) ) ;
#3297=CARTESIAN_POINT ( 'NONE',  ( -7.360235569667860744, -62.74547149457073658, -0.09995255151716124498 ) ) ;
#3298=CARTESIAN_POINT ( 'NONE',  ( -1.069819614139539521, -66.15452850542925489, -2.969112962950023249 ) ) ;
#3301=CARTESIAN_POINT ( 'NONE',  ( -2.882544866740875733, -90.60452850542925773, -0.8366430509618996147 ) ) ;
#3302=CARTESIAN_POINT ( 'NONE',  ( -0.09506052544085875911, -96.00452850542926342, -6.999999999999997335 ) ) ;
#3304=CARTESIAN_POINT ( 'NONE',  ( -1.719659006605371632, -81.15452850542922647, -4.969112962950016588 ) ) ;
#3305=CARTESIAN_POINT ( 'NONE',  ( 4.191402346623080533, -91.69547149457075363, -5.607243785695398941 ) ) ;
#3308=CARTESIAN_POINT ( 'NONE',  ( -1.719659006605374518, -60.15452850542926200, -4.969112962950016588 ) ) ;
#3309=APPLICATION_CONTEXT ( 'automotive_design' ) ;
#3310=CARTESIAN_POINT ( 'NONE',  ( -4.037591185471543831, -86.29547149457074795, -5.718994135553860936 ) ) ;
#3312=CARTESIAN_POINT ( 'NONE',  ( 3.015831842038233734, -76.80452850542926058, 3.989209796945429432 ) ) ;
#3316=CARTESIAN_POINT ( 'NONE',  ( 1.719659006605286367, -82.84547149457074511, -4.969112962950050338 ) ) ;
#3318=CARTESIAN_POINT ( 'NONE',  ( 0.09506052544077478461, -64.99547149457075079, -2.999999999999997780 ) ) ;
#3319=CARTESIAN_POINT ( 'NONE',  ( -2.369498399071207739, -66.15452850542925489, -6.969112962950009482 ) ) ;
#3321=CARTESIAN_POINT ( 'NONE',  ( -2.862020680886579793, -83.29547149457074795, -4.100960146803977580 ) ) ;
#3322=CARTESIAN_POINT ( 'NONE',  ( 4.312004677471073855, -58.95452850542925205, 3.009306630940844496 ) ) ;
#3323=CARTESIAN_POINT ( 'NONE',  ( 2.862020680886515400, -86.70452850542925205, -4.100960146804039752 ) ) ;
#3324=CARTESIAN_POINT ( 'NONE',  ( 4.037591185471441690, -71.70452850542925205, -5.718994135553947977 ) ) ;
#3326=CARTESIAN_POINT ( 'NONE',  ( 2.610703060766946138, -82.54547149457074795, -1.773238653441125523 ) ) ;
#3330=CARTESIAN_POINT ( 'NONE',  ( -1.719659006605371188, -84.15452850542925489, -4.969112962950016588 ) ) ;
#3332=CARTESIAN_POINT ( 'NONE',  ( 1.719659006605392060, -85.65452850542924068, 4.969112962950015699 ) ) ;
#3333=CARTESIAN_POINT ( 'NONE',  ( -1.069819614139472463, -90.34547149457073090, 2.969112962950044121 ) ) ;
#3335=CARTESIAN_POINT ( 'NONE',  ( 0.09506052544086121547, -85.50452850542926342, 4.999999999999997335 ) ) ;
#3336=CARTESIAN_POINT ( 'NONE',  ( -2.179377348189613262, -59.14547149457074227, -7.030887037049939003 ) ) ;
#3337=CARTESIAN_POINT ( 'NONE',  ( 0.8796985632578971925, -62.85452850542923642, -3.030887037049972310 ) ) ;
#3341=CARTESIAN_POINT ( 'NONE',  ( 2.610703060766983885, -73.95452850542925205, 1.773238653441072232 ) ) ;
#3342=CARTESIAN_POINT ( 'NONE',  ( -6.013306294175150946, -84.45452850542925205, -4.245374608440613429 ) ) ;
#3344=CARTESIAN_POINT ( 'NONE',  ( 6.628020296210689111, -85.09547149457075932, 2.253526892787472757 ) ) ;
#3347=CARTESIAN_POINT ( 'NONE',  ( 3.154386672714808437, -70.24547149457075079, 0.09995255151720662534 ) ) ;
#3350=CARTESIAN_POINT ( 'NONE',  ( 4.194503406049337357, -74.55452850542923215, -3.171033256558100089 ) ) ;
#3351=CARTESIAN_POINT ( 'NONE',  ( 4.191402346623081421, -94.69547149457076785, -5.607243785695398941 ) ) ;
#3353=CARTESIAN_POINT ( 'NONE',  ( -5.257311121191324155, -78.75452850542924921, 0.09995255151729526277 ) ) ;
#3360=CARTESIAN_POINT ( 'NONE',  ( -1.529537955723777154, -77.14547149457074227, -5.030887037049945221 ) ) ;
#3362=CARTESIAN_POINT ( 'NONE',  ( 3.154386672714807105, -64.24547149457075079, 0.09995255151720662534 ) ) ;
#3364=CARTESIAN_POINT ( 'NONE',  ( -6.013306294175152722, -69.45452850542925205, -4.245374608440613429 ) ) ;
#3366=CARTESIAN_POINT ( 'NONE',  ( -4.784657899331158148, -74.89547149457074227, 1.454677039711874675 ) ) ;
#3368=CARTESIAN_POINT ( 'NONE',  ( 4.784657899331211439, -89.10452850542925773, 1.454677039711774533 ) ) ;
#3369=CARTESIAN_POINT ( 'NONE',  ( -4.037591185471423927, -67.20452850542925205, 5.718994135553947977 ) ) ;
#3371=CARTESIAN_POINT ( 'NONE',  ( -2.882544866740857969, -77.89547149457074227, 0.8366430509619596778 ) ) ;
#3375=CARTESIAN_POINT ( 'NONE',  ( 5.257311121191342806, -86.25452850542924921, -0.09995255151729465215 ) ) ;
#3377=CARTESIAN_POINT ( 'NONE',  ( 0.09506052544086121547, -85.50452850542926342, 4.999999999999997335 ) ) ;
#3378=CARTESIAN_POINT ( 'NONE',  ( -0.09506052544075481447, -90.49547149457075079, 2.999999999999997780 ) ) ;
#3382=CARTESIAN_POINT ( 'NONE',  ( -4.784657899331189235, -90.60452850542925773, -1.454677039711773867 ) ) ;
#3383=CARTESIAN_POINT ( 'NONE',  ( 5.895805022753492608, -60.94547149457074653, 4.407101234057782868 ) ) ;
#3384=CARTESIAN_POINT ( 'NONE',  ( -2.882544866740878398, -69.60452850542924352, -0.8366430509618996147 ) ) ;
#3385=( GEOMETRIC_REPRESENTATION_CONTEXT ( 3 ) GLOBAL_UNCERTAINTY_ASSIGNED_CONTEXT ( ( #6117 ) ) GLOBAL_UNIT_ASSIGNED_CONTEXT ( ( #1409, #7864, #6671 ) ) REPRESENTATION_CONTEXT ( 'NONE', 'WORKASPACE' ) );
#3388=CARTESIAN_POINT ( 'NONE',  ( -2.823794231030021251, -75.90452850542925489, 1.017458915287783316 ) ) ;
#3389=CARTESIAN_POINT ( 'NONE',  ( -6.013306294175149169, -87.45452850542925205, -4.245374608440613429 ) ) ;
#3391=CARTESIAN_POINT ( 'NONE',  ( -0.09506052544071229293, -90.49547149457075079, 6.999999999999997335 ) ) ;
#3394=CARTESIAN_POINT ( 'NONE',  ( 1.840261337453219292, -67.69547149457073942, -2.371175808195584267 ) ) ;
#3395=CARTESIAN_POINT ( 'NONE',  ( -2.862020680886496748, -58.20452850542925916, 4.100960146804039752 ) ) ;
#3397=CARTESIAN_POINT ( 'NONE',  ( 4.194503406049335581, -68.55452850542926058, -3.171033256558100089 ) ) ;
#3398=CARTESIAN_POINT ( 'NONE',  ( 2.179377348189630137, -84.64547149457074227, 7.030887037049939003 ) ) ;
#3400=CARTESIAN_POINT ( 'NONE',  ( -4.194503406049316041, -79.05452850542921794, 3.171033256558100533 ) ) ;
#3402=CARTESIAN_POINT ( 'NONE',  ( -5.257311121191324155, -65.74547149457073658, -0.09995255151718371311 ) ) ;
#3404=CARTESIAN_POINT ( 'NONE',  ( -2.610703060766927930, -60.04547149457073374, 1.773238653441125745 ) ) ;
#3405=CARTESIAN_POINT ( 'NONE',  ( -6.686770931921506289, -66.60452850542924352, -2.072711028461647675 ) ) ;
#3408=CARTESIAN_POINT ( 'NONE',  ( -1.719659006605370744, -87.15452850542926910, -4.969112962950016588 ) ) ;
#3409=CARTESIAN_POINT ( 'NONE',  ( 4.191402346623195996, -64.80452850542926058, 5.607243785695311900 ) ) ;
#3410=CARTESIAN_POINT ( 'NONE',  ( -2.610703060766925709, -81.04547149457074795, 1.773238653441125745 ) ) ;
#3415=CARTESIAN_POINT ( 'NONE',  ( 1.529537955723692111, -89.85452850542925773, -5.030887037049978971 ) ) ;
#3417=CARTESIAN_POINT ( 'NONE',  ( -4.725907263620321430, -75.90452850542925489, 1.635492904037698647 ) ) ;
#3418=CARTESIAN_POINT ( 'NONE',  ( -1.686450176301614645, -95.29547149457076216, -2.482926158054096000 ) ) ;
#3419=CARTESIAN_POINT ( 'NONE',  ( -4.784657899331190123, -84.60452850542927195, -1.454677039711773867 ) ) ;
#3420=CARTESIAN_POINT ( 'NONE',  ( 6.686770931921476979, -64.39547149457074227, -2.072711028461788896 ) ) ;
#3422=CARTESIAN_POINT ( 'NONE',  ( 2.493201789345270480, -65.55452850542926058, -1.934965279058294518 ) ) ;
#3425=CARTESIAN_POINT ( 'NONE',  ( 2.493201789345271369, -77.55452850542926058, -1.934965279058294518 ) ) ;
#3427=CARTESIAN_POINT ( 'NONE',  ( 6.013306294175171374, -85.95452850542925205, 4.245374608440616093 ) ) ;
#3429=CARTESIAN_POINT ( 'NONE',  ( 7.360235569667878508, -85.24547149457075079, 0.09995255151716216091 ) ) ;
#3432=CARTESIAN_POINT ( 'NONE',  ( -1.069819614139475350, -72.34547149457073090, 2.969112962950044121 ) ) ;
#3436=CARTESIAN_POINT ( 'NONE',  ( 3.015831842038232846, -67.80452850542926058, 3.989209796945429432 ) ) ;
#3437=CARTESIAN_POINT ( 'NONE',  ( -7.360235569667858968, -77.74547149457073658, -0.09995255151716124498 ) ) ;
#3439=CARTESIAN_POINT ( 'NONE',  ( 2.862020680886512736, -65.70452850542925205, -4.100960146804039752 ) ) ;
#3442=CARTESIAN_POINT ( 'NONE',  ( -1.529537955723777820, -68.14547149457075648, -5.030887037049945221 ) ) ;
#3444=CARTESIAN_POINT ( 'NONE',  ( 2.882544866740875289, -61.39547149457074937, -0.8366430509619593447 ) ) ;
#3445=CARTESIAN_POINT ( 'NONE',  ( -7.360235569667860744, -60.75452850542924921, 0.09995255151731782806 ) ) ;
#3447=CARTESIAN_POINT ( 'NONE',  ( 1.719659006605392504, -88.65452850542925489, 4.969112962950016588 ) ) ;
#3448=CARTESIAN_POINT ( 'NONE',  ( -0.09506052544086292244, -63.00452850542925631, -6.999999999999997335 ) ) ;
#3449=CARTESIAN_POINT ( 'NONE',  ( -0.8796985632579421566, -83.14547149457072805, -3.030887037049952326 ) ) ;
#3453=CARTESIAN_POINT ( 'NONE',  ( -4.194503406049316041, -82.05452850542924637, 3.171033256558100533 ) ) ;
#3455=CARTESIAN_POINT ( 'NONE',  ( -2.862020680886494528, -76.20452850542926626, 4.100960146804039752 ) ) ;
#3456=CARTESIAN_POINT ( 'NONE',  ( -2.493201789345290020, -86.44547149457073942, -1.934965279058240561 ) ) ;
#3457=CARTESIAN_POINT ( 'NONE',  ( -4.725907263620350740, -95.59547149457074511, -1.635492904037597617 ) ) ;
#3458=CARTESIAN_POINT ( 'NONE',  ( 4.725907263620340082, -74.40452850542925489, -1.635492904037697981 ) ) ;
#3459=CARTESIAN_POINT ( 'NONE',  ( 2.179377348189484032, -92.85452850542924352, -7.030887037049986077 ) ) ;
#3460=CARTESIAN_POINT ( 'NONE',  ( -2.610703060766966122, -69.45452850542925205, -1.773238653441072232 ) ) ;
#3464=CARTESIAN_POINT ( 'NONE',  ( -0.09506052544081895761, -78.00452850542926342, -2.999999999999997780 ) ) ;
#3465=CARTESIAN_POINT ( 'NONE',  ( 6.013306294175171374, -91.95452850542925205, 4.245374608440616093 ) ) ;
#3466=CARTESIAN_POINT ( 'NONE',  ( -6.013306294175058575, -90.04547149457074795, 4.245374608440741326 ) ) ;
#3469=CARTESIAN_POINT ( 'NONE',  ( -0.8796985632579442660, -65.14547149457074227, -3.030887037049952326 ) ) ;
#3473=CARTESIAN_POINT ( 'NONE',  ( -5.257311121191324155, -69.75452850542926342, 0.09995255151729526277 ) ) ;
#3474=CARTESIAN_POINT ( 'NONE',  ( 7.360235569667878508, -85.24547149457075079, 0.09995255151716216091 ) ) ;
#3476=CARTESIAN_POINT ( 'NONE',  ( -4.784657899331191011, -66.60452850542924352, -1.454677039711773867 ) ) ;
#3478=CARTESIAN_POINT ( 'NONE',  ( -4.784657899331159037, -71.89547149457074227, 1.454677039711874675 ) ) ;
#3479=CARTESIAN_POINT ( 'NONE',  ( 0.7550207793516368060, -97.00000000000001421, -3.949353336951454629 ) ) ;
#3480=CARTESIAN_POINT ( 'NONE',  ( -4.194503406049381766, -95.44547149457071100, -3.171033256558012159 ) ) ;
#3481=CARTESIAN_POINT ( 'NONE',  ( 2.179377348189480035, -62.85452850542923642, -7.030887037049986077 ) ) ;
#3484=CARTESIAN_POINT ( 'NONE',  ( 4.784657899331210551, -80.10452850542925773, 1.454677039711774533 ) ) ;
#3488=CARTESIAN_POINT ( 'NONE',  ( -1.529537955723668352, -91.35452850542921510, 5.030887037049979860 ) ) ;
#3489=CARTESIAN_POINT ( 'NONE',  ( -4.784657899331190123, -75.60452850542925773, -1.454677039711773867 ) ) ;
#3491=CARTESIAN_POINT ( 'NONE',  ( 2.862020680886514068, -74.70452850542926626, -4.100960146804039752 ) ) ;
#3492=CARTESIAN_POINT ( 'NONE',  ( 0.09506052544077857325, -94.99547149457075079, -2.999999999999997780 ) ) ;
#3493=CARTESIAN_POINT ( 'NONE',  ( 2.610703060766943029, -61.54547149457074084, -1.773238653441125523 ) ) ;
#3494=CARTESIAN_POINT ( 'NONE',  ( -5.257311121191324155, -78.75452850542924921, 0.09995255151729526277 ) ) ;
#3495=CARTESIAN_POINT ( 'NONE',  ( -6.686770931921503625, -87.60452850542924352, -2.072711028461647675 ) ) ;
#3496=CARTESIAN_POINT ( 'NONE',  ( 1.686450176301638626, -96.79547149457073374, 2.482926158054096000 ) ) ;
#3502=CARTESIAN_POINT ( 'NONE',  ( -1.840261337453251267, -81.30452850542926058, -2.371175808195547852 ) ) ;
#3503=CARTESIAN_POINT ( 'NONE',  ( 5.895805022753407343, -86.55452850542926058, -4.407101234057908989 ) ) ;
#3504=CARTESIAN_POINT ( 'NONE',  ( 4.037591185471563371, -81.79547149457074795, 5.718994135553860936 ) ) ;
#3507=CARTESIAN_POINT ( 'NONE',  ( 3.750550224659021659, -96.89549487877602019, 3.480863915964662159 ) ) ;
#3508=CARTESIAN_POINT ( 'NONE',  ( 3.154386672714807549, -67.24547149457075079, 0.09995255151720662534 ) ) ;
#3509=PRODUCT_DEFINITION_CONTEXT ( 'detailed design', #3309, 'design' ) ;
#3513=CARTESIAN_POINT ( 'NONE',  ( 2.862020680886512736, -65.70452850542925205, -4.100960146804039752 ) ) ;
#3514=CARTESIAN_POINT ( 'NONE',  ( -4.037591185471544719, -77.29547149457074795, -5.718994135553860936 ) ) ;
#3516=CARTESIAN_POINT ( 'NONE',  ( -5.257311121191325043, -77.74547149457072237, -0.09995255151718372699 ) ) ;
#3517=CARTESIAN_POINT ( 'NONE',  ( 5.257311121191341918, -64.24547149457073658, 0.09995255151718437925 ) ) ;
#3518=CARTESIAN_POINT ( 'NONE',  ( -4.194503406049320482, -64.05452850542926058, 3.171033256558100533 ) ) ;
#3520=CARTESIAN_POINT ( 'NONE',  ( -2.862020680886581125, -71.29547149457074795, -4.100960146803977580 ) ) ;
#3522=CARTESIAN_POINT ( 'NONE',  ( 6.013306294175167821, -58.95452850542925916, 4.245374608440616093 ) ) ;
#3527=CARTESIAN_POINT ( 'NONE',  ( -4.725907263620320542, -84.90452850542925489, 1.635492904037698647 ) ) ;
#3528=CARTESIAN_POINT ( 'NONE',  ( 4.194503406049337357, -77.55452850542926058, -3.171033256558100089 ) ) ;
#3530=CARTESIAN_POINT ( 'NONE',  ( 3.015831842038233290, -70.80452850542926058, 3.989209796945429432 ) ) ;
#3531=CARTESIAN_POINT ( 'NONE',  ( 2.610703060766946138, -82.54547149457074795, -1.773238653441125523 ) ) ;
#3532=CARTESIAN_POINT ( 'NONE',  ( 0.8796985632579598091, -60.64547149457074227, 3.030887037049952326 ) ) ;
#3533=CARTESIAN_POINT ( 'NONE',  ( 4.312004677471075631, -73.95452850542926626, 3.009306630940844496 ) ) ;
#3534=CARTESIAN_POINT ( 'NONE',  ( 6.686770931921525829, -92.10452850542925773, 2.072711028461649008 ) ) ;
#3536=CARTESIAN_POINT ( 'NONE',  ( -1.840261337453254153, -57.30452850542924637, -2.371175808195547852 ) ) ;
#3540=CARTESIAN_POINT ( 'NONE',  ( -2.823794231030022583, -63.90452850542925489, 1.017458915287783316 ) ) ;
#3541=CARTESIAN_POINT ( 'NONE',  ( 6.628020296210642037, -80.40452850542925489, -2.253526892787612645 ) ) ;
#3542=CARTESIAN_POINT ( 'NONE',  ( 2.369498399071078509, -82.84547149457074511, -6.969112962950057444 ) ) ;
#3544=CARTESIAN_POINT ( 'NONE',  ( 1.529537955723797582, -93.64547149457074227, 5.030887037049945221 ) ) ;
#3545=CARTESIAN_POINT ( 'NONE',  ( -3.154386672714788453, -84.75452850542926342, 0.09995255151727280851 ) ) ;
#3550=CARTESIAN_POINT ( 'NONE',  ( 5.257311121191341918, -65.25452850542926342, -0.09995255151729465215 ) ) ;
#3551=CARTESIAN_POINT ( 'NONE',  ( 6.628020296210689111, -85.09547149457075932, 2.253526892787472757 ) ) ;
#3552=PRESENTATION_STYLE_ASSIGNMENT (( #7350 ) ) ;
#3554=CARTESIAN_POINT ( 'NONE',  ( -4.312004677470993030, -75.04547149457074795, 3.009306630940933314 ) ) ;
#3555=CARTESIAN_POINT ( 'NONE',  ( -1.529537955723777820, -71.14547149457071384, -5.030887037049945221 ) ) ;
#3557=CARTESIAN_POINT ( 'NONE',  ( 4.312004677471073855, -61.95452850542923784, 3.009306630940844496 ) ) ;
#3560=CARTESIAN_POINT ( 'NONE',  ( 4.312004677471011682, -73.54547149457073374, -3.009306630940933314 ) ) ;
#3562=CARTESIAN_POINT ( 'NONE',  ( 1.529537955723692999, -95.85452850542922931, -5.030887037049978971 ) ) ;
#3567=CARTESIAN_POINT ( 'NONE',  ( -4.784657899331189235, -87.60452850542925773, -1.454677039711773867 ) ) ;
#3568=CARTESIAN_POINT ( 'NONE',  ( 2.862020680886514068, -74.70452850542926626, -4.100960146804039752 ) ) ;
#3570=CARTESIAN_POINT ( 'NONE',  ( 4.194503406049338246, -74.55452850542924637, -3.171033256558100977 ) ) ;
#3571=CARTESIAN_POINT ( 'NONE',  ( 1.840261337453220625, -76.69547149457073942, -2.371175808195584267 ) ) ;
#3573=CARTESIAN_POINT ( 'NONE',  ( 3.015831842038151578, -97.69547149457075363, -3.989209796945492048 ) ) ;
#3575=CARTESIAN_POINT ( 'NONE',  ( 1.719659006605389173, -64.65452850542925489, 4.969112962950016588 ) ) ;
#3576=CARTESIAN_POINT ( 'NONE',  ( 7.360235569667880284, -86.25452850542924921, -0.09995255151731691212 ) ) ;
#3577=CARTESIAN_POINT ( 'NONE',  ( 0.8796985632578967484, -59.85452850542925773, -3.030887037049972310 ) ) ;
#3582=ADVANCED_BREP_SHAPE_REPRESENTATION ( '', ( #7136, #2840 ), #3385 ) ;
#3583=CARTESIAN_POINT ( 'NONE',  ( -0.09506052544083767875, -96.00452850542926342, -4.999999999999997335 ) ) ;
#3584=CARTESIAN_POINT ( 'NONE',  ( -1.686450176301566906, -67.20452850542925205, 2.482926158054133303 ) ) ;
#3585=CARTESIAN_POINT ( 'NONE',  ( 7.360235569667878508, -82.24547149457073658, 0.09995255151716216091 ) ) ;
#3588=CARTESIAN_POINT ( 'NONE',  ( -0.09506052544081780575, -87.00452850542926342, -2.999999999999997780 ) ) ;
#3592=CARTESIAN_POINT ( 'NONE',  ( 1.686450176301588000, -95.70452850542928047, -2.482926158054133303 ) ) ;
#3593=CARTESIAN_POINT ( 'NONE',  ( -6.013306294175061240, -72.04547149457074795, 4.245374608440741326 ) ) ;
#3597=CARTESIAN_POINT ( 'NONE',  ( -5.257311121191325043, -74.74547149457073658, -0.09995255151718372699 ) ) ;
#3598=CARTESIAN_POINT ( 'NONE',  ( 4.784657899331176800, -70.39547149457074227, -1.454677039711874009 ) ) ;
#3599=CARTESIAN_POINT ( 'NONE',  ( 4.784657899331207886, -62.10452850542925063, 1.454677039711774533 ) ) ;
#3602=CARTESIAN_POINT ( 'NONE',  ( -0.09506052544073692601, -63.49547149457074369, 4.999999999999997335 ) ) ;
#3605=CARTESIAN_POINT ( 'NONE',  ( 4.784657899331212327, -95.10452850542925773, 1.454677039711774533 ) ) ;
#3612=CARTESIAN_POINT ( 'NONE',  ( -4.312004677471056091, -90.45452850542926626, -3.009306630940844052 ) ) ;
#3613=CARTESIAN_POINT ( 'NONE',  ( 5.257311121191341918, -80.25452850542922079, -0.09995255151729465215 ) ) ;
#3614=CARTESIAN_POINT ( 'NONE',  ( -1.719659006605374074, -63.15452850542925489, -4.969112962950015699 ) ) ;
#3615=CARTESIAN_POINT ( 'NONE',  ( 3.154386672714809325, -76.24547149457073658, 0.09995255151720662534 ) ) ;
#3616=CARTESIAN_POINT ( 'NONE',  ( -0.8796985632579448211, -62.14547149457074937, -3.030887037049952326 ) ) ;
#3617=CARTESIAN_POINT ( 'NONE',  ( 4.725907263620340082, -71.40452850542925489, -1.635492904037697981 ) ) ;
#3618=CARTESIAN_POINT ( 'NONE',  ( 2.179377348189482699, -83.85452850542927195, -7.030887037049986077 ) ) ;
#3619=CARTESIAN_POINT ( 'NONE',  ( 1.686450176301583337, -59.70452850542925916, -2.482926158054133303 ) ) ;
#3625=CARTESIAN_POINT ( 'NONE',  ( -1.719659006605370744, -93.15452850542925489, -4.969112962950015699 ) ) ;
#3626=CARTESIAN_POINT ( 'NONE',  ( 1.069819614139556396, -70.65452850542925489, 2.969112962950023249 ) ) ;
#3628=CARTESIAN_POINT ( 'NONE',  ( 6.686770931921477867, -79.39547149457074227, -2.072711028461788896 ) ) ;
#3629=CARTESIAN_POINT ( 'NONE',  ( 0.09506052544086235345, -94.50452850542926342, 4.999999999999997335 ) ) ;
#3630=CARTESIAN_POINT ( 'NONE',  ( 5.257311121191343695, -94.24547149457072237, 0.09995255151718437925 ) ) ;
#3631=CARTESIAN_POINT ( 'NONE',  ( 1.686450176301586890, -89.70452850542925205, -2.482926158054133303 ) ) ;
#3638=CARTESIAN_POINT ( 'NONE',  ( 1.686450176301587334, -92.70452850542926626, -2.482926158054133303 ) ) ;
#3639=CARTESIAN_POINT ( 'NONE',  ( -4.191402346623058328, -72.19547149457073942, 5.607243785695398941 ) ) ;
#3640=CARTESIAN_POINT ( 'NONE',  ( 5.604172532792750516, -97.00000000000004263, 0.4687073228881366016 ) ) ;
#3642=CARTESIAN_POINT ( 'NONE',  ( -4.194503406049383543, -74.44547149457072521, -3.171033256558012159 ) ) ;
#3643=CARTESIAN_POINT ( 'NONE',  ( -2.862020680886582014, -65.29547149457073374, -4.100960146803977580 ) ) ;
#3644=CARTESIAN_POINT ( 'NONE',  ( -4.784657899331192787, -57.60452850542925773, -1.454677039711773867 ) ) ;
#3646=CARTESIAN_POINT ( 'NONE',  ( -4.784657899331160813, -59.89547149457074227, 1.454677039711874675 ) ) ;
#3647=CARTESIAN_POINT ( 'NONE',  ( -2.862020680886492308, -94.20452850542926626, 4.100960146804039752 ) ) ;
#3652=CARTESIAN_POINT ( 'NONE',  ( 0.09506052544086121547, -85.50452850542926342, 4.999999999999997335 ) ) ;
#3653=CARTESIAN_POINT ( 'NONE',  ( 1.529537955723796472, -87.64547149457071384, 5.030887037049945221 ) ) ;
#3654=ADVANCED_FACE ( 'NONE', ( #3932 ), #3974, .F. ) ;
#3655=CARTESIAN_POINT ( 'NONE',  ( -3.015831842038216859, -63.30452850542925347, -3.989209796945429432 ) ) ;
#3656=CARTESIAN_POINT ( 'NONE',  ( -1.840261337453199975, -81.19547149457073942, 2.371175808195584267 ) ) ;
#3657=CARTESIAN_POINT ( 'NONE',  ( -3.015831842038127597, -87.19547149457073942, 3.989209796945492048 ) ) ;
#3658=CARTESIAN_POINT ( 'NONE',  ( 4.194503406049335581, -65.55452850542923215, -3.171033256558100089 ) ) ;
#3659=CARTESIAN_POINT ( 'NONE',  ( -6.628020296210620721, -75.90452850542925489, 2.253526892787613978 ) ) ;
#3660=CARTESIAN_POINT ( 'NONE',  ( 2.823794231030062107, -94.09547149457074511, 1.017458915287723809 ) ) ;
#3665=CARTESIAN_POINT ( 'NONE',  ( -2.862020680886492308, -94.20452850542926626, 4.100960146804039752 ) ) ;
#3666=CARTESIAN_POINT ( 'NONE',  ( -2.823794231030021695, -72.90452850542925489, 1.017458915287783316 ) ) ;
#3667=CARTESIAN_POINT ( 'NONE',  ( 1.529537955723692555, -92.85452850542925773, -5.030887037049978971 ) ) ;
#3668=CARTESIAN_POINT ( 'NONE',  ( -6.628020296210667794, -74.59547149457071669, -2.253526892787471869 ) ) ;
#3669=CARTESIAN_POINT ( 'NONE',  ( 1.529537955723692555, -92.85452850542925773, -5.030887037049978971 ) ) ;
#3671=CARTESIAN_POINT ( 'NONE',  ( 1.719659006605287477, -91.84547149457074511, -4.969112962950050338 ) ) ;
#3672=CARTESIAN_POINT ( 'NONE',  ( 0.8796985632578997460, -83.85452850542927195, -3.030887037049972310 ) ) ;
#3676=CARTESIAN_POINT ( 'NONE',  ( 1.529537955723688336, -59.85452850542924352, -5.030887037049978971 ) ) ;
#3677=CARTESIAN_POINT ( 'NONE',  ( 0.09506052544073349819, -70.99547149457075079, -6.999999999999997335 ) ) ;
#3679=CARTESIAN_POINT ( 'NONE',  ( -5.108479284279210399E-14, -97.00000000000000000, -5.999999999999992006 ) ) ;
#3680=CARTESIAN_POINT ( 'NONE',  ( 2.862020680886598001, -63.79547149457074084, 4.100960146803977580 ) ) ;
#3681=CARTESIAN_POINT ( 'NONE',  ( 1.529537955723794695, -66.64547149457071384, 5.030887037049945221 ) ) ;
#3682=CARTESIAN_POINT ( 'NONE',  ( -2.493201789345250052, -91.05452850542926058, 1.934965279058294518 ) ) ;
#3686=CARTESIAN_POINT ( 'NONE',  ( -4.194503406049316929, -73.05452850542926058, 3.171033256558100533 ) ) ;
#3687=CARTESIAN_POINT ( 'NONE',  ( -1.529537955723778930, -59.14547149457072805, -5.030887037049945221 ) ) ;
#3696=CARTESIAN_POINT ( 'NONE',  ( 5.257311121191341918, -80.25452850542922079, -0.09995255151729465215 ) ) ;
#3697=CARTESIAN_POINT ( 'NONE',  ( 2.862020680886601109, -90.79547149457074795, 4.100960146803977580 ) ) ;
#3698=CARTESIAN_POINT ( 'NONE',  ( -1.529537955723672571, -58.35452850542925063, 5.030887037049979860 ) ) ;
#3699=CARTESIAN_POINT ( 'NONE',  ( 2.823794231030060775, -85.09547149457075932, 1.017458915287723809 ) ) ;
#3700=CARTESIAN_POINT ( 'NONE',  ( 6.013306294175169597, -76.95452850542926626, 4.245374608440616093 ) ) ;
#3701=CARTESIAN_POINT ( 'NONE',  ( 4.312004677471013459, -85.54547149457070532, -3.009306630940933314 ) ) ;
#3702=CARTESIAN_POINT ( 'NONE',  ( -5.257311121191324155, -63.75452850542925631, 0.09995255151729526277 ) ) ;
#3703=CARTESIAN_POINT ( 'NONE',  ( -2.369498399071206407, -78.15452850542924068, -6.969112962950009482 ) ) ;
#3704=CARTESIAN_POINT ( 'NONE',  ( 0.09506052544077779609, -88.99547149457075079, -2.999999999999997780 ) ) ;
#3709=CARTESIAN_POINT ( 'NONE',  ( 4.725907263620341858, -89.40452850542926910, -1.635492904037697981 ) ) ;
#3710=CARTESIAN_POINT ( 'NONE',  ( -3.154386672714791118, -66.75452850542926342, 0.09995255151727280851 ) ) ;
#3711=CARTESIAN_POINT ( 'NONE',  ( -2.179377348189463603, -58.35452850542927195, 7.030887037049988741 ) ) ;
#3712=CARTESIAN_POINT ( 'NONE',  ( -7.360235569667858968, -71.74547149457075079, -0.09995255151716124498 ) ) ;
#3714=CARTESIAN_POINT ( 'NONE',  ( 4.784657899331178577, -85.39547149457074227, -1.454677039711874009 ) ) ;
#3715=CARTESIAN_POINT ( 'NONE',  ( 3.154386672714809325, -77.25452850542924921, -0.09995255151727241993 ) ) ;
#3720=CARTESIAN_POINT ( 'NONE',  ( 2.610703060766986106, -94.95452850542926626, 1.773238653441072232 ) ) ;
#3721=CARTESIAN_POINT ( 'NONE',  ( -4.191402346623058328, -75.19547149457073942, 5.607243785695398941 ) ) ;
#3722=CARTESIAN_POINT ( 'NONE',  ( 4.302742873392585210, -96.99999999999947420, 2.548615363087012753 ) ) ;
#3723=CARTESIAN_POINT ( 'NONE',  ( -2.862020680886582014, -62.29547149457074084, -4.100960146803977580 ) ) ;
#3724=CARTESIAN_POINT ( 'NONE',  ( -0.09506052544071151578, -96.49547149457075079, 6.999999999999997335 ) ) ;
#3725=CARTESIAN_POINT ( 'NONE',  ( 1.719659006605388285, -58.65452850542924068, 4.969112962950016588 ) ) ;
#3728=CARTESIAN_POINT ( 'NONE',  ( 0.09506052544085895339, -67.50452850542926342, 4.999999999999997335 ) ) ;
#3729=CARTESIAN_POINT ( 'NONE',  ( -2.369498399071054529, -96.34547149457074511, 6.969112962950058332 ) ) ;
#3735=CARTESIAN_POINT ( 'NONE',  ( 4.194503406049338246, -80.55452850542926058, -3.171033256558100089 ) ) ;
#3736=CARTESIAN_POINT ( 'NONE',  ( 4.312004677471013459, -85.54547149457070532, -3.009306630940933314 ) ) ;
#3737=CARTESIAN_POINT ( 'NONE',  ( 3.015831842038232402, -64.80452850542926058, 3.989209796945429432 ) ) ;
#3738=CARTESIAN_POINT ( 'NONE',  ( 1.069819614139493558, -70.84547149457073090, -2.969112962950042789 ) ) ;
#3739=CARTESIAN_POINT ( 'NONE',  ( 0.09506052544088137990, -76.50452850542926342, 6.999999999999997335 ) ) ;
#3740=CARTESIAN_POINT ( 'NONE',  ( -3.015831842038127153, -90.19547149457073942, 3.989209796945492048 ) ) ;
#3741=CARTESIAN_POINT ( 'NONE',  ( -0.09506052544084186984, -63.00452850542925631, -4.999999999999997335 ) ) ;
#3742=CARTESIAN_POINT ( 'NONE',  ( -6.686770931921506289, -78.60452850542927195, -2.072711028461647675 ) ) ;
#3743=CARTESIAN_POINT ( 'NONE',  ( -2.610703060766923933, -90.04547149457074795, 1.773238653441125745 ) ) ;
#3748=CARTESIAN_POINT ( 'NONE',  ( 2.862020680886515844, -89.70452850542926626, -4.100960146804039752 ) ) ;
#3749=CARTESIAN_POINT ( 'NONE',  ( 2.882544866740894829, -62.10452850542925063, 0.8366430509618999478 ) ) ;
#3750=CARTESIAN_POINT ( 'NONE',  ( 0.09506052544087911782, -58.50452850542925631, 6.999999999999997335 ) ) ;
#3752=CARTESIAN_POINT ( 'NONE',  ( 7.360235569667877620, -73.24547149457075079, 0.09995255151716216091 ) ) ;
#3754=CARTESIAN_POINT ( 'NONE',  ( 2.862020680886599777, -81.79547149457073374, 4.100960146803977580 ) ) ;
#3755=CARTESIAN_POINT ( 'NONE',  ( 0.8796985632578988579, -74.85452850542925773, -3.030887037049972310 ) ) ;
#3760=CARTESIAN_POINT ( 'NONE',  ( -2.862020680886496748, -58.20452850542925916, 4.100960146804039752 ) ) ;
#3762=CARTESIAN_POINT ( 'NONE',  ( 4.191402346623077868, -67.69547149457073942, -5.607243785695398941 ) ) ;
#3764=CARTESIAN_POINT ( 'NONE',  ( 4.312004677471010794, -67.54547149457074795, -3.009306630940932425 ) ) ;
#3765=CARTESIAN_POINT ( 'NONE',  ( -5.257311121191324155, -62.74547149457075079, -0.09995255151718371311 ) ) ;
#3766=CARTESIAN_POINT ( 'NONE',  ( 0.8796985632579013004, -95.85452850542924352, -3.030887037049972310 ) ) ;
#3769=CARTESIAN_POINT ( 'NONE',  ( -5.257311121191324155, -72.75452850542924921, 0.09995255151729526277 ) ) ;
#3770=CARTESIAN_POINT ( 'NONE',  ( -6.628020296210665130, -95.59547149457074511, -2.253526892787471869 ) ) ;
#3779=CARTESIAN_POINT ( 'NONE',  ( 0.09506052544086046607, -79.50452850542926342, 4.999999999999997335 ) ) ;
#3780=CARTESIAN_POINT ( 'NONE',  ( 4.312004677471013459, -91.54547149457074795, -3.009306630940933314 ) ) ;
#3781=CARTESIAN_POINT ( 'NONE',  ( -4.784657899331192787, -57.60452850542925773, -1.454677039711773867 ) ) ;
#3782=CARTESIAN_POINT ( 'NONE',  ( -1.840261337453200863, -72.19547149457073942, 2.371175808195584267 ) ) ;
#3783=CARTESIAN_POINT ( 'NONE',  ( 7.360235569667877620, -77.25452850542924921, -0.09995255151731691212 ) ) ;
#3784=CARTESIAN_POINT ( 'NONE',  ( -2.862020680886579349, -89.29547149457074795, -4.100960146803977580 ) ) ;
#3785=CARTESIAN_POINT ( 'NONE',  ( -4.725907263620323207, -60.90452850542925489, 1.635492904037698647 ) ) ;
#3786=CARTESIAN_POINT ( 'NONE',  ( -5.895805022753386027, -82.05452850542926058, 4.407101234057909878 ) ) ;
#3787=CARTESIAN_POINT ( 'NONE',  ( 2.493201789345311337, -87.94547149457073942, 1.934965279058241006 ) ) ;
#3792=CARTESIAN_POINT ( 'NONE',  ( 5.257311121191344583, -95.25452850542926342, -0.09995255151729466603 ) ) ;
#3793=CARTESIAN_POINT ( 'NONE',  ( 2.882544866740880174, -97.39547149457074227, -0.8366430509619593447 ) ) ;
#3795=CARTESIAN_POINT ( 'NONE',  ( -1.529537955723667908, -94.35452850542922931, 5.030887037049979860 ) ) ;
#3796=CARTESIAN_POINT ( 'NONE',  ( 6.628020296210686446, -67.09547149457073090, 2.253526892787472757 ) ) ;
#3797=CARTESIAN_POINT ( 'NONE',  ( -1.529537955723775378, -89.14547149457074227, -5.030887037049945221 ) ) ;
#3798=CARTESIAN_POINT ( 'NONE',  ( -2.823794231030021695, -72.90452850542925489, 1.017458915287783316 ) ) ;
#3801=CARTESIAN_POINT ( 'NONE',  ( 3.154386672714811102, -92.25452850542926342, -0.09995255151727241993 ) ) ;
#3802=CARTESIAN_POINT ( 'NONE',  ( -4.037591185471546495, -65.29547149457073374, -5.718994135553860936 ) ) ;
#3804=CARTESIAN_POINT ( 'NONE',  ( 1.719659006605283702, -61.84547149457073800, -4.969112962950050338 ) ) ;
#3805=CARTESIAN_POINT ( 'NONE',  ( 4.191402346623081421, -97.69547149457076785, -5.607243785695398941 ) ) ;
#3806=CARTESIAN_POINT ( 'NONE',  ( -1.069819614139536190, -93.15452850542925489, -2.969112962950023249 ) ) ;
#3808=CARTESIAN_POINT ( 'NONE',  ( -4.725907263620322318, -69.90452850542925489, 1.635492904037698647 ) ) ;
#3809=CARTESIAN_POINT ( 'NONE',  ( 5.895805022753496161, -90.94547149457073942, 4.407101234057782868 ) ) ;
#3817=CARTESIAN_POINT ( 'NONE',  ( -4.312004677471057867, -78.45452850542925205, -3.009306630940844052 ) ) ;
#3819=CARTESIAN_POINT ( 'NONE',  ( 4.194503406049402194, -87.94547149457072521, 3.171033256558012159 ) ) ;
#3821=CARTESIAN_POINT ( 'NONE',  ( -1.069819614139474906, -75.34547149457073090, 2.969112962950044121 ) ) ;
#3822=CARTESIAN_POINT ( 'NONE',  ( 5.895805022753406455, -83.55452850542926058, -4.407101234057908989 ) ) ;
#3823=CARTESIAN_POINT ( 'NONE',  ( -5.257311121191323267, -86.74547149457072237, -0.09995255151718371311 ) ) ;
#3825=CARTESIAN_POINT ( 'NONE',  ( -2.179377348189460939, -82.35452850542927195, 7.030887037049988741 ) ) ;
#3827=CARTESIAN_POINT ( 'NONE',  ( 0.8796985632579634729, -90.64547149457075648, 3.030887037049952326 ) ) ;
#3833=CARTESIAN_POINT ( 'NONE',  ( -5.257311121191325043, -78.75452850542926342, 0.09995255151729529053 ) ) ;
#3834=CARTESIAN_POINT ( 'NONE',  ( 1.840261337453268586, -58.80452850542926058, 2.371175808195547852 ) ) ;
#3836=CARTESIAN_POINT ( 'NONE',  ( 3.015831842038235955, -91.80452850542926058, 3.989209796945429432 ) ) ;
#3837=CARTESIAN_POINT ( 'NONE',  ( 0.09506052544073349819, -70.99547149457075079, -6.999999999999997335 ) ) ;
#3838=CARTESIAN_POINT ( 'NONE',  ( -3.015831842038128041, -84.19547149457073942, 3.989209796945492048 ) ) ;
#3839=CARTESIAN_POINT ( 'NONE',  ( 2.610703060766983885, -73.95452850542925205, 1.773238653441072232 ) ) ;
#3840=CARTESIAN_POINT ( 'NONE',  ( -5.108479284279210399E-14, -97.00000000000000000, -5.999999999999992006 ) ) ;
#3841=SURFACE_STYLE_USAGE ( .BOTH. , #6873 ) ;
#3842=CARTESIAN_POINT ( 'NONE',  ( 1.069819614139558173, -85.65452850542926910, 2.969112962950023249 ) ) ;
#3843=CARTESIAN_POINT ( 'NONE',  ( 6.686770931921476979, -61.39547149457074937, -2.072711028461788896 ) ) ;
#3845=CARTESIAN_POINT ( 'NONE',  ( -4.194503406049383543, -68.44547149457073942, -3.171033256558012159 ) ) ;
#3846=CARTESIAN_POINT ( 'NONE',  ( 1.719659006605283480, -61.84547149457073090, -4.969112962950050338 ) ) ;
#3849=CARTESIAN_POINT ( 'NONE',  ( -3.015831842038216859, -63.30452850542925347, -3.989209796945429432 ) ) ;
#3850=CARTESIAN_POINT ( 'NONE',  ( -6.686770931921458327, -86.89547149457074227, 2.072711028461789784 ) ) ;
#3857=CARTESIAN_POINT ( 'NONE',  ( -1.719659006605372076, -75.15452850542925489, -4.969112962950016588 ) ) ;
#3858=CARTESIAN_POINT ( 'NONE',  ( -3.015831842038128929, -78.19547149457075363, 3.989209796945492048 ) ) ;
#3860=CARTESIAN_POINT ( 'NONE',  ( 1.840261337453219292, -67.69547149457073942, -2.371175808195584267 ) ) ;
#3861=CARTESIAN_POINT ( 'NONE',  ( 4.191402346623196884, -70.80452850542926058, 5.607243785695311900 ) ) ;
#3863=CARTESIAN_POINT ( 'NONE',  ( 2.862020680886599333, -78.79547149457074795, 4.100960146803977580 ) ) ;
#3864=CARTESIAN_POINT ( 'NONE',  ( -1.719659006605374518, -60.15452850542926200, -4.969112962950016588 ) ) ;
#3865=CARTESIAN_POINT ( 'NONE',  ( -1.529537955723668352, -91.35452850542921510, 5.030887037049979860 ) ) ;
#3866=CARTESIAN_POINT ( 'NONE',  ( 6.628020296210639373, -68.40452850542925489, -2.253526892787612645 ) ) ;
#3867=CARTESIAN_POINT ( 'NONE',  ( -2.610703060766923933, -93.04547149457074795, 1.773238653441125745 ) ) ;
#3871=CARTESIAN_POINT ( 'NONE',  ( -1.529537955723668574, -88.35452850542925773, 5.030887037049979860 ) ) ;
#3873=CARTESIAN_POINT ( 'NONE',  ( 0.09506052544086007750, -76.50452850542924921, 4.999999999999997335 ) ) ;
#3874=CARTESIAN_POINT ( 'NONE',  ( -1.069819614139540409, -60.15452850542926200, -2.969112962950023249 ) ) ;
#3877=CARTESIAN_POINT ( 'NONE',  ( 5.257311121191341918, -83.25452850542926342, -0.09995255151729465215 ) ) ;
#3878=CARTESIAN_POINT ( 'NONE',  ( 6.013306294175077227, -70.54547149457074795, -4.245374608440741326 ) ) ;
#3879=CARTESIAN_POINT ( 'NONE',  ( -5.257311121191323267, -83.74547149457075079, -0.09995255151718372699 ) ) ;
#3880=CARTESIAN_POINT ( 'NONE',  ( -3.154386672714789341, -78.75452850542926342, 0.09995255151727280851 ) ) ;
#3881=DIRECTION ( 'NONE',  ( -0.9954714945707483498, -0.09506052544079830746, 1.046913586349167774E-14 ) ) ;
#3883=CARTESIAN_POINT ( 'NONE',  ( 2.493201789345273589, -92.55452850542926058, -1.934965279058294518 ) ) ;
#3884=EDGE_CURVE ( 'NONE', #1590, #7927, #797, .T. ) ;
#3885=CARTESIAN_POINT ( 'NONE',  ( -5.895805022753479285, -65.44547149457075363, -4.407101234057782868 ) ) ;
#3887=CARTESIAN_POINT ( 'NONE',  ( 2.862020680886514956, -80.70452850542925205, -4.100960146804039752 ) ) ;
#3888=CARTESIAN_POINT ( 'NONE',  ( -4.312004677470995695, -60.04547149457074795, 3.009306630940933758 ) ) ;
#3893=CARTESIAN_POINT ( 'NONE',  ( -1.529537955723672349, -58.35452850542924352, 5.030887037049979860 ) ) ;
#3894=CARTESIAN_POINT ( 'NONE',  ( 2.179377348189631025, -90.64547149457075648, 7.030887037049939003 ) ) ;
#3897=CARTESIAN_POINT ( 'NONE',  ( -3.015831842038214639, -78.30452850542926058, -3.989209796945429432 ) ) ;
#3901=CARTESIAN_POINT ( 'NONE',  ( -1.719659006605264828, -81.34547149457074511, 4.969112962950051227 ) ) ;
#3903=CARTESIAN_POINT ( 'NONE',  ( -3.154386672714790674, -71.74547149457075079, -0.09995255151720625064 ) ) ;
#3904=CARTESIAN_POINT ( 'NONE',  ( 0.09506052544088100520, -73.50452850542924921, 6.999999999999997335 ) ) ;
#3906=CARTESIAN_POINT ( 'NONE',  ( 4.312004677471012570, -79.54547149457074795, -3.009306630940933314 ) ) ;
#3907=CARTESIAN_POINT ( 'NONE',  ( 3.015831842038231958, -58.80452850542925347, 3.989209796945429432 ) ) ;
#3908=CARTESIAN_POINT ( 'NONE',  ( 5.257311121191343695, -95.25452850542924921, -0.09995255151729465215 ) ) ;
#3910=CARTESIAN_POINT ( 'NONE',  ( -2.369498399071207739, -69.15452850542926910, -6.969112962950009482 ) ) ;
#3911=CARTESIAN_POINT ( 'NONE',  ( 1.069819614139494890, -79.84547149457074511, -2.969112962950042789 ) ) ;
#3914=CARTESIAN_POINT ( 'NONE',  ( 4.725907263620341858, -92.40452850542925489, -1.635492904037697981 ) ) ;
#3915=CARTESIAN_POINT ( 'NONE',  ( -4.312004677471056091, -90.45452850542926626, -3.009306630940844052 ) ) ;
#3917=CARTESIAN_POINT ( 'NONE',  ( 4.312004677471078296, -79.95452850542923784, 3.009306630940844052 ) ) ;
#3918=CARTESIAN_POINT ( 'NONE',  ( -2.882544866740878842, -63.60452850542924352, -0.8366430509618996147 ) ) ;
#3920=CARTESIAN_POINT ( 'NONE',  ( 5.257311121191342806, -86.25452850542924921, -0.09995255151729465215 ) ) ;
#3921=CARTESIAN_POINT ( 'NONE',  ( -2.369498399071058969, -63.34547149457073800, 6.969112962950058332 ) ) ;
#3923=CARTESIAN_POINT ( 'NONE',  ( -0.8796985632578808723, -64.35452850542924352, 3.030887037049973198 ) ) ;
#3924=CARTESIAN_POINT ( 'NONE',  ( 0.09506052544075790922, -97.99547149457075079, -4.999999999999997335 ) ) ;
#3926=CARTESIAN_POINT ( 'NONE',  ( 1.686450176301586890, -89.70452850542925205, -2.482926158054133303 ) ) ;
#3927=CARTESIAN_POINT ( 'NONE',  ( -7.360235569667860744, -65.74547149457073658, -0.09995255151716124498 ) ) ;
#3929=CARTESIAN_POINT ( 'NONE',  ( 1.529537955723690557, -80.85452850542925773, -5.030887037049978971 ) ) ;
#3930=CARTESIAN_POINT ( 'NONE',  ( -4.191402346623055664, -93.19547149457075363, 5.607243785695398941 ) ) ;
#3932=FACE_OUTER_BOUND ( 'NONE', #4143, .T. ) ;
#3933=CARTESIAN_POINT ( 'NONE',  ( 2.862020680886512292, -62.70452850542926626, -4.100960146804039752 ) ) ;
#3934=CARTESIAN_POINT ( 'NONE',  ( -6.628020296210666018, -86.59547149457075932, -2.253526892787471869 ) ) ;
#3937=CARTESIAN_POINT ( 'NONE',  ( 0.09506052544086007750, -76.50452850542924921, 4.999999999999997335 ) ) ;
#3940=CARTESIAN_POINT ( 'NONE',  ( 4.194503406049402194, -81.94547149457073942, 3.171033256558012159 ) ) ;
#3941=CARTESIAN_POINT ( 'NONE',  ( -0.09506052544084261924, -57.00452850542924921, -4.999999999999997335 ) ) ;
#3942=CARTESIAN_POINT ( 'NONE',  ( -1.686450176301619308, -59.29547149457074084, -2.482926158054096000 ) ) ;
#3943=CARTESIAN_POINT ( 'NONE',  ( -0.09506052544086251999, -66.00452850542926342, -6.999999999999997335 ) ) ;
#3945=ADVANCED_FACE ( 'NONE', ( #7579 ), #4370, .F. ) ;
#3946=CARTESIAN_POINT ( 'NONE',  ( 4.194503406049402194, -75.94547149457075363, 3.171033256558012159 ) ) ;
#3948=CARTESIAN_POINT ( 'NONE',  ( 1.529537955723692111, -89.85452850542925773, -5.030887037049978971 ) ) ;
#3949=CARTESIAN_POINT ( 'NONE',  ( -4.037591185471423927, -70.20452850542925205, 5.718994135553947977 ) ) ;
#3950=CARTESIAN_POINT ( 'NONE',  ( -3.154386672714790674, -74.74547149457073658, -0.09995255151720625064 ) ) ;
#3955=CARTESIAN_POINT ( 'NONE',  ( 2.862020680886515844, -89.70452850542926626, -4.100960146804039752 ) ) ;
#3957=CARTESIAN_POINT ( 'NONE',  ( -4.194503406049316929, -85.05452850542926058, 3.171033256558101865 ) ) ;
#3958=CARTESIAN_POINT ( 'NONE',  ( 2.610703060766947470, -91.54547149457074795, -1.773238653441125523 ) ) ;
#3961=CARTESIAN_POINT ( 'NONE',  ( -4.194503406049316041, -82.05452850542924637, 3.171033256558100533 ) ) ;
#3962=CARTESIAN_POINT ( 'NONE',  ( -6.686770931921461880, -59.89547149457074937, 2.072711028461789784 ) ) ;
#3964=CARTESIAN_POINT ( 'NONE',  ( -2.882544866740878842, -63.60452850542924352, -0.8366430509618996147 ) ) ;
#3968=CARTESIAN_POINT ( 'NONE',  ( 0.09506052544083881672, -76.50452850542926342, 2.999999999999997780 ) ) ;
#3969=CARTESIAN_POINT ( 'NONE',  ( -5.895805022753383362, -94.05452850542926058, 4.407101234057909878 ) ) ;
#3971=CARTESIAN_POINT ( 'NONE',  ( 2.862020680886514068, -74.70452850542926626, -4.100960146804039752 ) ) ;
#3972=CARTESIAN_POINT ( 'NONE',  ( -6.686770931921456551, -89.89547149457074227, 2.072711028461789784 ) ) ;
#3974=PLANE ( 'NONE',  #2869 ) ;
#3975=CARTESIAN_POINT ( 'NONE',  ( 0.8796985632579613634, -72.64547149457072805, 3.030887037049952326 ) ) ;
#3977=CARTESIAN_POINT ( 'NONE',  ( 4.725907263620339194, -62.40452850542925489, -1.635492904037697981 ) ) ;
#3978=CARTESIAN_POINT ( 'NONE',  ( 2.369498399071078509, -85.84547149457074511, -6.969112962950057444 ) ) ;
#3981=CARTESIAN_POINT ( 'NONE',  ( -2.862020680886494084, -79.20452850542925205, 4.100960146804039752 ) ) ;
#3984=CARTESIAN_POINT ( 'NONE',  ( 3.015831842038149802, -82.69547149457073942, -3.989209796945492048 ) ) ;
#3986=CARTESIAN_POINT ( 'NONE',  ( -0.8796985632579442660, -65.14547149457074227, -3.030887037049952326 ) ) ;
#3987=CARTESIAN_POINT ( 'NONE',  ( -7.360235569667858968, -69.75452850542926342, 0.09995255151731782806 ) ) ;
#3989=CARTESIAN_POINT ( 'NONE',  ( 4.784657899331177688, -79.39547149457074227, -1.454677039711874009 ) ) ;
#3991=CARTESIAN_POINT ( 'NONE',  ( 0.09506052544086160405, -88.50452850542924921, 4.999999999999997335 ) ) ;
#3992=CARTESIAN_POINT ( 'NONE',  ( 6.013306294175167821, -64.95452850542926626, 4.245374608440616093 ) ) ;
#3993=CARTESIAN_POINT ( 'NONE',  ( -2.493201789345290464, -77.44547149457073942, -1.934965279058240561 ) ) ;
#3996=CARTESIAN_POINT ( 'NONE',  ( 4.784657899331212327, -95.10452850542925773, 1.454677039711774533 ) ) ;
#3997=CARTESIAN_POINT ( 'NONE',  ( 0.09506052544086160405, -88.50452850542924921, 4.999999999999997335 ) ) ;
#3999=CARTESIAN_POINT ( 'NONE',  ( -4.725907263620320542, -84.90452850542925489, 1.635492904037698647 ) ) ;
#4000=CARTESIAN_POINT ( 'NONE',  ( 1.840261337453222179, -94.69547149457076785, -2.371175808195584267 ) ) ;
#4002=CARTESIAN_POINT ( 'NONE',  ( -3.015831842038213750, -90.30452850542926058, -3.989209796945429432 ) ) ;
#4003=CARTESIAN_POINT ( 'NONE',  ( -6.628020296210618056, -93.90452850542926910, 2.253526892787613978 ) ) ;
#4004=CARTESIAN_POINT ( 'NONE',  ( -2.493201789345253161, -67.05452850542926058, 1.934965279058294518 ) ) ;
#4008=CARTESIAN_POINT ( 'NONE',  ( 3.154386672714809325, -80.25452850542926342, -0.09995255151727241993 ) ) ;
#4009=CARTESIAN_POINT ( 'NONE',  ( -7.360235569667856304, -93.75452850542926342, 0.09995255151731782806 ) ) ;
#4011=CARTESIAN_POINT ( 'NONE',  ( 0.09506052544073539945, -85.99547149457075079, -6.999999999999997335 ) ) ;
#4014=CARTESIAN_POINT ( 'NONE',  ( 1.686450176301635295, -69.79547149457074795, 2.482926158054096000 ) ) ;
#4018=CARTESIAN_POINT ( 'NONE',  ( 0.09506052544085857869, -64.50452850542926342, 4.999999999999997335 ) ) ;
#4019=CARTESIAN_POINT ( 'NONE',  ( 4.037591185471563371, -84.79547149457074795, 5.718994135553860936 ) ) ;
#4021=CARTESIAN_POINT ( 'NONE',  ( 5.257311121191341918, -74.25452850542924921, -0.09995255151729465215 ) ) ;
#4027=CARTESIAN_POINT ( 'NONE',  ( 1.529537955723795584, -75.64547149457069963, 5.030887037049945221 ) ) ;
#4029=CARTESIAN_POINT ( 'NONE',  ( -0.8796985632579448211, -62.14547149457074937, -3.030887037049952326 ) ) ;
#4031=CARTESIAN_POINT ( 'NONE',  ( -6.628020296210620721, -72.90452850542925489, 2.253526892787613978 ) ) ;
#4034=CARTESIAN_POINT ( 'NONE',  ( -4.194503406049316041, -82.05452850542924637, 3.171033256558100533 ) ) ;
#4035=CARTESIAN_POINT ( 'NONE',  ( -6.013306294175152722, -66.45452850542925205, -4.245374608440613429 ) ) ;
#4037=CARTESIAN_POINT ( 'NONE',  ( -2.882544866740857081, -80.89547149457074227, 0.8366430509619596778 ) ) ;
#4040=CARTESIAN_POINT ( 'NONE',  ( 4.194503406049340022, -95.55452850542921794, -3.171033256558100089 ) ) ;
#4041=CARTESIAN_POINT ( 'NONE',  ( -1.529537955723668796, -85.35452850542924352, 5.030887037049979860 ) ) ;
#4043=CARTESIAN_POINT ( 'NONE',  ( 5.257311121191341030, -74.25452850542924921, -0.09995255151729466603 ) ) ;
#4044=CARTESIAN_POINT ( 'NONE',  ( -1.069819614139472463, -93.34547149457073090, 2.969112962950044121 ) ) ;
#4045=CARTESIAN_POINT ( 'NONE',  ( 1.719659006605392060, -85.65452850542922647, 4.969112962950016588 ) ) ;
#4046=CARTESIAN_POINT ( 'NONE',  ( 2.179377348189627916, -63.64547149457072805, 7.030887037049939003 ) ) ;
#4047=CARTESIAN_POINT ( 'NONE',  ( -0.09506052544082045641, -66.00452850542926342, -2.999999999999997780 ) ) ;
#4051=CARTESIAN_POINT ( 'NONE',  ( 0.09506052544083956612, -82.50452850542926342, 2.999999999999997780 ) ) ;
#4052=CARTESIAN_POINT ( 'NONE',  ( 2.179377348189484032, -92.85452850542924352, -7.030887037049986077 ) ) ;
#4053=CARTESIAN_POINT ( 'NONE',  ( -6.686770931921458327, -86.89547149457074227, 2.072711028461789784 ) ) ;
#4056=CARTESIAN_POINT ( 'NONE',  ( 1.069819614139492669, -64.84547149457071669, -2.969112962950042789 ) ) ;
#4059=CARTESIAN_POINT ( 'NONE',  ( -2.862020680886495416, -70.20452850542925205, 4.100960146804039752 ) ) ;
#4060=CARTESIAN_POINT ( 'NONE',  ( -6.013306294175060351, -78.04547149457074795, 4.245374608440741326 ) ) ;
#4063=CARTESIAN_POINT ( 'NONE',  ( -4.194503406049316929, -73.05452850542926058, 3.171033256558100533 ) ) ;
#4065=CARTESIAN_POINT ( 'NONE',  ( 1.719659006605285034, -70.84547149457074511, -4.969112962950050338 ) ) ;
#4067=CARTESIAN_POINT ( 'NONE',  ( -3.015831842038126709, -96.19547149457075363, 3.989209796945492048 ) ) ;
#4068=CARTESIAN_POINT ( 'NONE',  ( -5.895805022753386915, -61.05452850542925347, 4.407101234057909878 ) ) ;
#4072=CARTESIAN_POINT ( 'NONE',  ( 4.194503406049338246, -83.55452850542921794, -3.171033256558100089 ) ) ;
#4073=CARTESIAN_POINT ( 'NONE',  ( 6.686770931921522276, -62.10452850542925063, 2.072711028461649008 ) ) ;
#4074=CARTESIAN_POINT ( 'NONE',  ( 1.069819614139494446, -76.84547149457073090, -2.969112962950042789 ) ) ;
#4077=CARTESIAN_POINT ( 'NONE',  ( -5.257311121191321490, -93.75452850542926342, 0.09995255151729526277 ) ) ;
#4078=CARTESIAN_POINT ( 'NONE',  ( 1.719659006605391394, -79.65452850542925489, 4.969112962950016588 ) ) ;
#4080=CARTESIAN_POINT ( 'NONE',  ( 4.725907263620340082, -71.40452850542925489, -1.635492904037697981 ) ) ;
#4081=CARTESIAN_POINT ( 'NONE',  ( 1.069819614139496666, -94.84547149457073090, -2.969112962950042789 ) ) ;
#4082=CARTESIAN_POINT ( 'NONE',  ( 3.154386672714807105, -61.24547149457073658, 0.09995255151720662534 ) ) ;
#4083=CARTESIAN_POINT ( 'NONE',  ( -4.191402346623176456, -93.30452850542926058, -5.607243785695311900 ) ) ;
#4085=CARTESIAN_POINT ( 'NONE',  ( 1.069819614139555064, -61.65452850542925489, 2.969112962950023249 ) ) ;
#4089=CARTESIAN_POINT ( 'NONE',  ( -0.09506052544084261924, -57.00452850542924921, -4.999999999999997335 ) ) ;
#4091=CARTESIAN_POINT ( 'NONE',  ( 1.686450176301586001, -80.70452850542925205, -2.482926158054133303 ) ) ;
#4093=CARTESIAN_POINT ( 'NONE',  ( 6.013306294175171374, -88.95452850542925205, 4.245374608440616093 ) ) ;
#4095=CARTESIAN_POINT ( 'NONE',  ( 6.686770931921479644, -91.39547149457074227, -2.072711028461788896 ) ) ;
#4098=CARTESIAN_POINT ( 'NONE',  ( -1.686450176301618642, -65.29547149457073374, -2.482926158054096000 ) ) ;
#4102=CARTESIAN_POINT ( 'NONE',  ( 2.862020680886513624, -71.70452850542925205, -4.100960146804039752 ) ) ;
#4103=CARTESIAN_POINT ( 'NONE',  ( -5.895805022753477509, -80.44547149457073942, -4.407101234057782868 ) ) ;
#4105=CARTESIAN_POINT ( 'NONE',  ( -1.529537955723671239, -70.35452850542925773, 5.030887037049979860 ) ) ;
#4106=DIRECTION ( 'NONE',  ( -0.09506052544079829358, 0.9954714945707483498, 0.000000000000000000 ) ) ;
#4107=CARTESIAN_POINT ( 'NONE',  ( 5.257311121191341918, -73.24547149457072237, 0.09995255151718437925 ) ) ;
#4110=CARTESIAN_POINT ( 'NONE',  ( 3.015831842038151134, -94.69547149457075363, -3.989209796945492048 ) ) ;
#4111=CARTESIAN_POINT ( 'NONE',  ( -2.369498399071207739, -57.15452850542926200, -6.969112962950009482 ) ) ;
#4113=CARTESIAN_POINT ( 'NONE',  ( -0.09506052544083960776, -81.00452850542926342, -4.999999999999997335 ) ) ;
#4116=CARTESIAN_POINT ( 'NONE',  ( 1.529537955723692111, -89.85452850542925773, -5.030887037049978971 ) ) ;
#4117=CARTESIAN_POINT ( 'NONE',  ( 2.862020680886514956, -80.70452850542925205, -4.100960146804039752 ) ) ;
#4120=CARTESIAN_POINT ( 'NONE',  ( 1.719659006605390505, -73.65452850542924068, 4.969112962950015699 ) ) ;
#4121=CARTESIAN_POINT ( 'NONE',  ( 2.823794231030061219, -88.09547149457074511, 1.017458915287723809 ) ) ;
#4122=CARTESIAN_POINT ( 'NONE',  ( -0.09506052544073315125, -93.49547149457073658, 4.999999999999997335 ) ) ;
#4123=CARTESIAN_POINT ( 'NONE',  ( -0.09506052544083998246, -78.00452850542926342, -4.999999999999997335 ) ) ;
#4124=CARTESIAN_POINT ( 'NONE',  ( -7.360235569667856304, -87.75452850542924921, 0.09995255151731782806 ) ) ;
#4125=CARTESIAN_POINT ( 'NONE',  ( 2.610703060766981665, -58.95452850542925916, 1.773238653441072232 ) ) ;
#4130=CARTESIAN_POINT ( 'NONE',  ( 2.882544866740896161, -74.10452850542924352, 0.8366430509618999478 ) ) ;
#4131=CARTESIAN_POINT ( 'NONE',  ( -6.628020296210619833, -87.90452850542926910, 2.253526892787613978 ) ) ;
#4132=CARTESIAN_POINT ( 'NONE',  ( -2.369498399071056305, -81.34547149457074511, 6.969112962950058332 ) ) ;
#4134=CARTESIAN_POINT ( 'NONE',  ( -1.719659006605263274, -96.34547149457074511, 4.969112962950051227 ) ) ;
#4135=CARTESIAN_POINT ( 'NONE',  ( -2.823794231030041235, -71.59547149457071669, -1.017458915287723364 ) ) ;
#4141=CARTESIAN_POINT ( 'NONE',  ( 1.529537955723689002, -65.85452850542924352, -5.030887037049978971 ) ) ;
#4142=CARTESIAN_POINT ( 'NONE',  ( 4.191402346623078756, -76.69547149457073942, -5.607243785695398941 ) ) ;
#4143=EDGE_LOOP ( 'NONE', ( #911, #2243, #496 ) ) ;
#4144=CARTESIAN_POINT ( 'NONE',  ( -4.194503406049383543, -77.44547149457075363, -3.171033256558012159 ) ) ;
#4145=CARTESIAN_POINT ( 'NONE',  ( 1.529537955723795584, -78.64547149457074227, 5.030887037049945221 ) ) ;
#4146=CARTESIAN_POINT ( 'NONE',  ( 0.09506052544085857869, -64.50452850542926342, 4.999999999999997335 ) ) ;
#4148=CARTESIAN_POINT ( 'NONE',  ( 0.09506052544075488386, -73.99547149457075079, -4.999999999999997335 ) ) ;
#4151=CARTESIAN_POINT ( 'NONE',  ( 7.360235569667875843, -62.25452850542926342, -0.09995255151731691212 ) ) ;
#4157=CARTESIAN_POINT ( 'NONE',  ( -5.257311121191322378, -90.75452850542924921, 0.09995255151729526277 ) ) ;
#4158=CARTESIAN_POINT ( 'NONE',  ( -1.719659006605371632, -81.15452850542922647, -4.969112962950016588 ) ) ;
#4160=CARTESIAN_POINT ( 'NONE',  ( 4.784657899331208775, -68.10452850542925773, 1.454677039711774533 ) ) ;
#4161=CARTESIAN_POINT ( 'NONE',  ( -0.09506052544075556388, -84.49547149457075079, 2.999999999999997780 ) ) ;
#4162=CARTESIAN_POINT ( 'NONE',  ( -2.493201789345292241, -62.44547149457074653, -1.934965279058240561 ) ) ;
#4163=CARTESIAN_POINT ( 'NONE',  ( -2.862020680886494528, -76.20452850542926626, 4.100960146804039752 ) ) ;
#4165=CARTESIAN_POINT ( 'NONE',  ( -5.895805022753383362, -88.05452850542926058, 4.407101234057909878 ) ) ;
#4166=CARTESIAN_POINT ( 'NONE',  ( -0.09506052544075442590, -93.49547149457075079, 2.999999999999997780 ) ) ;
#4171=CARTESIAN_POINT ( 'NONE',  ( 1.686450176301584669, -71.70452850542925205, -2.482926158054133303 ) ) ;
#4172=CARTESIAN_POINT ( 'NONE',  ( 6.686770931921525829, -89.10452850542925773, 2.072711028461649008 ) ) ;
#4173=CARTESIAN_POINT ( 'NONE',  ( 6.013306294175077227, -76.54547149457074795, -4.245374608440741326 ) ) ;
#4177=CARTESIAN_POINT ( 'NONE',  ( 2.823794231030041235, -86.40452850542926910, -1.017458915287783316 ) ) ;
#4181=CARTESIAN_POINT ( 'NONE',  ( 1.529537955723689224, -68.85452850542921510, -5.030887037049978971 ) ) ;
#4182=CARTESIAN_POINT ( 'NONE',  ( -6.686770931921459216, -77.89547149457074227, 2.072711028461789784 ) ) ;
#4184=CARTESIAN_POINT ( 'NONE',  ( -4.725907263620353405, -77.59547149457074511, -1.635492904037597617 ) ) ;
#4185=CARTESIAN_POINT ( 'NONE',  ( -4.725907263620354293, -68.59547149457073090, -1.635492904037597617 ) ) ;
#4186=CARTESIAN_POINT ( 'NONE',  ( -5.257311121191324155, -66.75452850542923500, 0.09995255151729526277 ) ) ;
#4190=CARTESIAN_POINT ( 'NONE',  ( -1.719659006605265716, -72.34547149457071669, 4.969112962950051227 ) ) ;
#4191=CARTESIAN_POINT ( 'NONE',  ( -7.360235569667860744, -57.75452850542924921, 0.09995255151731782806 ) ) ;
#4196=CARTESIAN_POINT ( 'NONE',  ( -0.09506052544083846978, -90.00452850542924921, -4.999999999999997335 ) ) ;
#4197=CARTESIAN_POINT ( 'NONE',  ( 1.529537955723690557, -80.85452850542925773, -5.030887037049978971 ) ) ;
#4199=CARTESIAN_POINT ( 'NONE',  ( -4.725907263620322318, -66.90452850542925489, 1.635492904037698647 ) ) ;
#4200=CARTESIAN_POINT ( 'NONE',  ( 2.493201789345310448, -81.94547149457073942, 1.934965279058241006 ) ) ;
#4201=CARTESIAN_POINT ( 'NONE',  ( -4.312004677470991254, -93.04547149457074795, 3.009306630940933758 ) ) ;
#4202=CARTESIAN_POINT ( 'NONE',  ( 4.784657899331208775, -65.10452850542924352, 1.454677039711774533 ) ) ;
#4203=CARTESIAN_POINT ( 'NONE',  ( 2.179377348189483143, -86.85452850542924352, -7.030887037049986077 ) ) ;
#4204=CARTESIAN_POINT ( 'NONE',  ( -1.069819614139472463, -93.34547149457073090, 2.969112962950044121 ) ) ;
#4210=CARTESIAN_POINT ( 'NONE',  ( 2.882544866740895717, -71.10452850542924352, 0.8366430509618999478 ) ) ;
#4212=CARTESIAN_POINT ( 'NONE',  ( 5.895805022753496161, -75.94547149457073942, 4.407101234057782868 ) ) ;
#4214=CARTESIAN_POINT ( 'NONE',  ( 4.725907263620374721, -94.09547149457074511, 1.635492904037598283 ) ) ;
#4215=CARTESIAN_POINT ( 'NONE',  ( 1.069819614139558617, -88.65452850542926910, 2.969112962950023249 ) ) ;
#4221=CARTESIAN_POINT ( 'NONE',  ( -4.725907263620324095, -57.90452850542925489, 1.635492904037698647 ) ) ;
#4222=CARTESIAN_POINT ( 'NONE',  ( 4.037591185471560706, -66.79547149457073374, 5.718994135553860936 ) ) ;
#4224=( LENGTH_UNIT ( ) NAMED_UNIT ( * ) SI_UNIT ( .MILLI., .METRE. ) );
#4226=CARTESIAN_POINT ( 'NONE',  ( 4.784657899331177688, -76.39547149457074227, -1.454677039711874009 ) ) ;
#4227=CARTESIAN_POINT ( 'NONE',  ( 3.015831842038147581, -67.69547149457073942, -3.989209796945492048 ) ) ;
#4229=CARTESIAN_POINT ( 'NONE',  ( 4.194503406049334693, -62.55452850542925347, -3.171033256558100089 ) ) ;
#4232=CARTESIAN_POINT ( 'NONE',  ( 4.725907263620371168, -64.09547149457073090, 1.635492904037598283 ) ) ;
#4234=CARTESIAN_POINT ( 'NONE',  ( 5.257311121191343695, -95.25452850542924921, -0.09995255151729465215 ) ) ;
#4240=CARTESIAN_POINT ( 'NONE',  ( 4.312004677471076519, -82.95452850542925205, 3.009306630940844496 ) ) ;
#4241=CARTESIAN_POINT ( 'NONE',  ( 4.312004677471075631, -73.95452850542926626, 3.009306630940844496 ) ) ;
#4242=CARTESIAN_POINT ( 'NONE',  ( 2.862020680886512292, -62.70452850542926626, -4.100960146804039752 ) ) ;
#4243=CARTESIAN_POINT ( 'NONE',  ( 3.154386672714809770, -79.24547149457073658, 0.09995255151720662534 ) ) ;
#4244=CARTESIAN_POINT ( 'NONE',  ( 4.784657899331179465, -94.39547149457074227, -1.454677039711874009 ) ) ;
#4245=CARTESIAN_POINT ( 'NONE',  ( 0.09506052544085932809, -70.50452850542926342, 4.999999999999997335 ) ) ;
#4246=CARTESIAN_POINT ( 'NONE',  ( -0.09506052544086027178, -84.00452850542926342, -6.999999999999997335 ) ) ;
#4247=CARTESIAN_POINT ( 'NONE',  ( 1.069819614139554842, -58.65452850542925489, 2.969112962950023249 ) ) ;
#4251=CARTESIAN_POINT ( 'NONE',  ( 3.015831842038235511, -88.80452850542926058, 3.989209796945429432 ) ) ;
#4252=CARTESIAN_POINT ( 'NONE',  ( -0.8796985632578796510, -73.35452850542924352, 3.030887037049973198 ) ) ;
#4253=CARTESIAN_POINT ( 'NONE',  ( 6.628020296210687334, -76.09547149457073090, 2.253526892787472757 ) ) ;
#4254=CARTESIAN_POINT ( 'NONE',  ( -4.725907263620318766, -93.90452850542925489, 1.635492904037698647 ) ) ;
#4255=CARTESIAN_POINT ( 'NONE',  ( -2.862020680886578905, -92.29547149457074795, -4.100960146803977580 ) ) ;
#4256=CARTESIAN_POINT ( 'NONE',  ( -2.493201789345250496, -88.05452850542926058, 1.934965279058294518 ) ) ;
#4260=CARTESIAN_POINT ( 'NONE',  ( -1.719659006605374518, -60.15452850542926200, -4.969112962950016588 ) ) ;
#4261=CARTESIAN_POINT ( 'NONE',  ( -4.191402346623058328, -69.19547149457073942, 5.607243785695398941 ) ) ;
#4262=CARTESIAN_POINT ( 'NONE',  ( 0.5177642813940753763, -97.00000000000001421, -5.999999999999999112 ) ) ;
#4263=CARTESIAN_POINT ( 'NONE',  ( -3.015831842038129373, -75.19547149457073942, 3.989209796945492048 ) ) ;
#4264=CARTESIAN_POINT ( 'NONE',  ( -4.194503406049384431, -65.44547149457072521, -3.171033256558012159 ) ) ;
#4265=CARTESIAN_POINT ( 'NONE',  ( -2.882544866740875733, -90.60452850542925773, -0.8366430509618996147 ) ) ;
#4269=CARTESIAN_POINT ( 'NONE',  ( -5.257311121191324155, -59.74547149457072948, -0.09995255151718371311 ) ) ;
#4271=CARTESIAN_POINT ( 'NONE',  ( -5.257311121191321490, -93.75452850542926342, 0.09995255151729526277 ) ) ;
#4274=UNCERTAINTY_MEASURE_WITH_UNIT (LENGTH_MEASURE( 1.000000000000000082E-05 ), #2414, 'distance_accuracy_value', 'NONE');
#4278=CARTESIAN_POINT ( 'NONE',  ( -1.719659006605370744, -87.15452850542926910, -4.969112962950016588 ) ) ;
#4279=CARTESIAN_POINT ( 'NONE',  ( 2.862020680886600665, -87.79547149457074795, 4.100960146803977580 ) ) ;
#4280=CARTESIAN_POINT ( 'NONE',  ( -2.862020680886496304, -61.20452850542925205, 4.100960146804039752 ) ) ;
#4281=CARTESIAN_POINT ( 'NONE',  ( 1.069819614139494890, -79.84547149457074511, -2.969112962950042789 ) ) ;
#4282=CARTESIAN_POINT ( 'NONE',  ( 2.862020680886601109, -90.79547149457074795, 4.100960146803977580 ) ) ;
#4283=CARTESIAN_POINT ( 'NONE',  ( 1.529537955723689002, -65.85452850542924352, -5.030887037049978971 ) ) ;
#4284=CARTESIAN_POINT ( 'NONE',  ( -0.09506052544085988321, -87.00452850542926342, -6.999999999999997335 ) ) ;
#4285=CARTESIAN_POINT ( 'NONE',  ( 2.882544866740880174, -97.39547149457074227, -0.8366430509619593447 ) ) ;
#4291=CARTESIAN_POINT ( 'NONE',  ( 4.312004677471078296, -94.95452850542926626, 3.009306630940844052 ) ) ;
#4292=CARTESIAN_POINT ( 'NONE',  ( 2.610703060766982553, -64.95452850542926626, 1.773238653441072232 ) ) ;
#4293=CARTESIAN_POINT ( 'NONE',  ( -2.882544866740855749, -95.89547149457075648, 0.8366430509619596778 ) ) ;
#4294=CARTESIAN_POINT ( 'NONE',  ( -6.628020296210666018, -83.59547149457075932, -2.253526892787471869 ) ) ;
#4295=CARTESIAN_POINT ( 'NONE',  ( 4.194503406049340022, -95.55452850542921794, -3.171033256558100089 ) ) ;
#4296=CARTESIAN_POINT ( 'NONE',  ( 4.312004677471013459, -91.54547149457074795, -3.009306630940932425 ) ) ;
#4297=CARTESIAN_POINT ( 'NONE',  ( 2.610703060766984773, -85.95452850542925205, 1.773238653441072232 ) ) ;
#4302=CARTESIAN_POINT ( 'NONE',  ( -2.610703060766962569, -93.45452850542926626, -1.773238653441072232 ) ) ;
#4303=CARTESIAN_POINT ( 'NONE',  ( -2.179377348189612373, -68.14547149457074227, -7.030887037049939003 ) ) ;
#4304=CARTESIAN_POINT ( 'NONE',  ( 5.646814530099427465, -96.99999999999992895, 0.2111776093032153578 ) ) ;
#4305=CARTESIAN_POINT ( 'NONE',  ( 5.257311121191341030, -70.24547149457076500, 0.09995255151718437925 ) ) ;
#4306=CARTESIAN_POINT ( 'NONE',  ( -4.784657899331159037, -71.89547149457074227, 1.454677039711874675 ) ) ;
#4307=CARTESIAN_POINT ( 'NONE',  ( -5.257311121191324155, -57.75452850542923500, 0.09995255151729526277 ) ) ;
#4309=CARTESIAN_POINT ( 'NONE',  ( -1.719659006605372964, -72.15452850542921226, -4.969112962950016588 ) ) ;
#4310=CARTESIAN_POINT ( 'NONE',  ( 1.719659006605283480, -61.84547149457073090, -4.969112962950050338 ) ) ;
#4316=CARTESIAN_POINT ( 'NONE',  ( 3.015831842038233734, -73.80452850542926058, 3.989209796945429432 ) ) ;
#4317=CARTESIAN_POINT ( 'NONE',  ( -5.257311121191322378, -92.74547149457073658, -0.09995255151718371311 ) ) ;
#4318=CARTESIAN_POINT ( 'NONE',  ( 5.257311121191341030, -59.25452850542924921, -0.09995255151729466603 ) ) ;
#4319=CARTESIAN_POINT ( 'NONE',  ( -3.154386672714789785, -77.74547149457073658, -0.09995255151720625064 ) ) ;
#4320=CARTESIAN_POINT ( 'NONE',  ( 6.686770931921524941, -83.10452850542927195, 2.072711028461649008 ) ) ;
#4321=CARTESIAN_POINT ( 'NONE',  ( -4.725907263620352516, -83.59547149457074511, -1.635492904037597617 ) ) ;
#4322=CARTESIAN_POINT ( 'NONE',  ( 0.09506052544085857869, -64.50452850542926342, 4.999999999999997335 ) ) ;
#4323=CARTESIAN_POINT ( 'NONE',  ( -4.191402346623179120, -78.30452850542926058, -5.607243785695311900 ) ) ;
#4324=CARTESIAN_POINT ( 'NONE',  ( 1.840261337453221957, -91.69547149457075363, -2.371175808195584267 ) ) ;
#4328=CARTESIAN_POINT ( 'NONE',  ( -4.194503406049316041, -91.05452850542924637, 3.171033256558101865 ) ) ;
#4329=CARTESIAN_POINT ( 'NONE',  ( -1.069819614139539521, -69.15452850542926910, -2.969112962950023249 ) ) ;
#4330=CARTESIAN_POINT ( 'NONE',  ( 6.013306294175167821, -58.95452850542925916, 4.245374608440616093 ) ) ;
#4331=CARTESIAN_POINT ( 'NONE',  ( 4.037591185471560706, -66.79547149457073374, 5.718994135553860936 ) ) ;
#4332=CARTESIAN_POINT ( 'NONE',  ( -2.862020680886492308, -94.20452850542926626, 4.100960146804039752 ) ) ;
#4333=ADVANCED_FACE ( 'NONE', ( #2819 ), #5960, .T. ) ;
#4335=CARTESIAN_POINT ( 'NONE',  ( -4.194503406049381766, -89.44547149457073942, -3.171033256558012159 ) ) ;
#4336=CARTESIAN_POINT ( 'NONE',  ( -1.686450176301564685, -85.20452850542925205, 2.482926158054133303 ) ) ;
#4340=CARTESIAN_POINT ( 'NONE',  ( -1.069819614139536190, -93.15452850542925489, -2.969112962950023249 ) ) ;
#4341=CARTESIAN_POINT ( 'NONE',  ( -5.895805022753479285, -71.44547149457072521, -4.407101234057782868 ) ) ;
#4344=CARTESIAN_POINT ( 'NONE',  ( 4.194503406049400418, -63.94547149457074653, 3.171033256558012159 ) ) ;
#4345=CARTESIAN_POINT ( 'NONE',  ( 4.312004677471010794, -64.54547149457073374, -3.009306630940933314 ) ) ;
#4346=CARTESIAN_POINT ( 'NONE',  ( -1.719659006605374518, -60.15452850542926200, -4.969112962950016588 ) ) ;
#4349=AXIS2_PLACEMENT_3D ( 'NONE', #8125, #8241, #1718 ) ;
#4350=CARTESIAN_POINT ( 'NONE',  ( -3.015831842038215527, -72.30452850542926058, -3.989209796945429432 ) ) ;
#4351=CARTESIAN_POINT ( 'NONE',  ( -3.015831842038131150, -60.19547149457074653, 3.989209796945492048 ) ) ;
#4359=CARTESIAN_POINT ( 'NONE',  ( -4.194503406049316929, -73.05452850542926058, 3.171033256558100533 ) ) ;
#4360=CARTESIAN_POINT ( 'NONE',  ( 0.09506052544075677124, -88.99547149457073658, -4.999999999999997335 ) ) ;
#4361=CARTESIAN_POINT ( 'NONE',  ( 1.719659006605389395, -64.65452850542925489, 4.969112962950015699 ) ) ;
#4362=CARTESIAN_POINT ( 'NONE',  ( 2.493201789345309560, -72.94547149457073942, 1.934965279058241006 ) ) ;
#4363=CARTESIAN_POINT ( 'NONE',  ( 7.360235569667878508, -80.25452850542926342, -0.09995255151731691212 ) ) ;
#4364=CARTESIAN_POINT ( 'NONE',  ( -4.725907263620351628, -92.59547149457074511, -1.635492904037597617 ) ) ;
#4365=CARTESIAN_POINT ( 'NONE',  ( -1.719659006605372964, -72.15452850542921226, -4.969112962950016588 ) ) ;
#4366=CARTESIAN_POINT ( 'NONE',  ( 4.191402346623197772, -73.80452850542926058, 5.607243785695311900 ) ) ;
#4367=CARTESIAN_POINT ( 'NONE',  ( 2.823794231030061219, -88.09547149457074511, 1.017458915287723809 ) ) ;
#4370=PLANE ( 'NONE',  #4614 ) ;
#4372=CARTESIAN_POINT ( 'NONE',  ( -0.09506052544083808120, -93.00452850542926342, -4.999999999999997335 ) ) ;
#4373=CARTESIAN_POINT ( 'NONE',  ( -2.493201789345254049, -61.05452850542925347, 1.934965279058294518 ) ) ;
#4374=CARTESIAN_POINT ( 'NONE',  ( -0.09506052544083770650, -96.00452850542926342, -4.999999999999997335 ) ) ;
#4375=CARTESIAN_POINT ( 'NONE',  ( -2.369498399071058969, -66.34547149457073090, 6.969112962950058332 ) ) ;
#4376=CARTESIAN_POINT ( 'NONE',  ( -4.312004677470992142, -84.04547149457074795, 3.009306630940933314 ) ) ;
#4377=CARTESIAN_POINT ( 'NONE',  ( -0.8796985632578788739, -79.35452850542927195, 3.030887037049973198 ) ) ;
#4381=ORIENTED_EDGE ( 'NONE', *, *, #5622, .F. ) ;
#4382=CARTESIAN_POINT ( 'NONE',  ( 4.194503406049334693, -59.55452850542926058, -3.171033256558100089 ) ) ;
#4383=CARTESIAN_POINT ( 'NONE',  ( 2.369498399071075845, -67.84547149457071669, -6.969112962950057444 ) ) ;
#4385=CARTESIAN_POINT ( 'NONE',  ( 3.015831842038146693, -61.69547149457073942, -3.989209796945492048 ) ) ;
#4386=CARTESIAN_POINT ( 'NONE',  ( -2.862020680886582458, -59.29547149457074084, -4.100960146803977580 ) ) ;
#4387=CARTESIAN_POINT ( 'NONE',  ( -2.862020680886496748, -58.20452850542925916, 4.100960146804039752 ) ) ;
#4389=CARTESIAN_POINT ( 'NONE',  ( 4.784657899331208775, -71.10452850542925773, 1.454677039711774533 ) ) ;
#4390=CARTESIAN_POINT ( 'NONE',  ( -4.312004677470995695, -60.04547149457074795, 3.009306630940933758 ) ) ;
#4396=CARTESIAN_POINT ( 'NONE',  ( -4.725907263620320542, -81.90452850542925489, 1.635492904037698647 ) ) ;
#4397=CARTESIAN_POINT ( 'NONE',  ( 4.194503406049402194, -93.94547149457075363, 3.171033256558012159 ) ) ;
#4398=CARTESIAN_POINT ( 'NONE',  ( -4.194503406049321370, -58.05452850542925347, 3.171033256558101865 ) ) ;
#4399=CARTESIAN_POINT ( 'NONE',  ( 0.8796985632579618075, -75.64547149457072805, 3.030887037049952326 ) ) ;
#4400=CARTESIAN_POINT ( 'NONE',  ( -6.013306294175150946, -81.45452850542925205, -4.245374608440613429 ) ) ;
#4401=CARTESIAN_POINT ( 'NONE',  ( 4.725907263620374721, -88.09547149457074511, 1.635492904037598283 ) ) ;
#4403=CARTESIAN_POINT ( 'NONE',  ( -2.369498399071206851, -75.15452850542922647, -6.969112962950009482 ) ) ;
#4404=CARTESIAN_POINT ( 'NONE',  ( 1.069819614139495556, -85.84547149457074511, -2.969112962950042789 ) ) ;
#4407=CARTESIAN_POINT ( 'NONE',  ( -4.725907263620356069, -59.59547149457074511, -1.635492904037597617 ) ) ;
#4409=CARTESIAN_POINT ( 'NONE',  ( 1.529537955723692111, -89.85452850542925773, -5.030887037049978971 ) ) ;
#4410=CARTESIAN_POINT ( 'NONE',  ( -1.840261337453254153, -57.30452850542924637, -2.371175808195547852 ) ) ;
#4411=CARTESIAN_POINT ( 'NONE',  ( 6.628020296210639373, -59.40452850542925489, -2.253526892787612645 ) ) ;
#4412=CARTESIAN_POINT ( 'NONE',  ( 6.628020296210686446, -73.09547149457071669, 2.253526892787472757 ) ) ;
#4414=CARTESIAN_POINT ( 'NONE',  ( 2.862020680886600221, -84.79547149457074795, 4.100960146803977580 ) ) ;
#4415=CARTESIAN_POINT ( 'NONE',  ( -2.610703060766965233, -75.45452850542925205, -1.773238653441072232 ) ) ;
#4418=CARTESIAN_POINT ( 'NONE',  ( 2.610703060766986106, -91.95452850542925205, 1.773238653441072232 ) ) ;
#4420=CARTESIAN_POINT ( 'NONE',  ( 2.369498399071075401, -61.84547149457074511, -6.969112962950057444 ) ) ;
#4422=CARTESIAN_POINT ( 'NONE',  ( 4.194503406049400418, -60.94547149457073232, 3.171033256558012159 ) ) ;
#4423=CARTESIAN_POINT ( 'NONE',  ( 2.369498399071080286, -97.84547149457073090, -6.969112962950057444 ) ) ;
#4424=CARTESIAN_POINT ( 'NONE',  ( 2.862020680886511848, -59.70452850542925205, -4.100960146804039752 ) ) ;
#4427=CARTESIAN_POINT ( 'NONE',  ( -1.719659006605373408, -69.15452850542924068, -4.969112962950016588 ) ) ;
#4430=CARTESIAN_POINT ( 'NONE',  ( -6.628020296210665130, -89.59547149457074511, -2.253526892787471869 ) ) ;
#4439=CARTESIAN_POINT ( 'NONE',  ( -4.194503406049316041, -82.05452850542924637, 3.171033256558100533 ) ) ;
#4440=CARTESIAN_POINT ( 'NONE',  ( 2.862020680886601554, -93.79547149457074795, 4.100960146803977580 ) ) ;
#4441=CARTESIAN_POINT ( 'NONE',  ( 4.266483400374380786, -96.99999999999998579, 2.517034344952451264 ) ) ;
#4442=CARTESIAN_POINT ( 'NONE',  ( -3.154386672714791118, -68.74547149457075079, -0.09995255151720625064 ) ) ;
#4443=CARTESIAN_POINT ( 'NONE',  ( 2.369498399071225947, -82.65452850542926910, 6.969112962950009482 ) ) ;
#4444=CARTESIAN_POINT ( 'NONE',  ( 5.257311121191342806, -91.24547149457072237, 0.09995255151718437925 ) ) ;
#4446=CARTESIAN_POINT ( 'NONE',  ( 2.369498399071225947, -82.65452850542926910, 6.969112962950009482 ) ) ;
#4447=CARTESIAN_POINT ( 'NONE',  ( -1.840261337453198864, -90.19547149457073942, 2.371175808195584267 ) ) ;
#4452=CARTESIAN_POINT ( 'NONE',  ( 1.719659006605391616, -82.65452850542925489, 4.969112962950015699 ) ) ;
#4453=CARTESIAN_POINT ( 'NONE',  ( 2.493201789345312669, -96.94547149457073942, 1.934965279058241006 ) ) ;
#4454=CARTESIAN_POINT ( 'NONE',  ( -5.895805022753386915, -58.05452850542925347, 4.407101234057909878 ) ) ;
#4455=CARTESIAN_POINT ( 'NONE',  ( 2.179377348189629249, -72.64547149457072805, 7.030887037049939003 ) ) ;
#4456=CARTESIAN_POINT ( 'NONE',  ( 1.719659006605286811, -85.84547149457075932, -4.969112962950050338 ) ) ;
#4457=CARTESIAN_POINT ( 'NONE',  ( 0.09506052544083919142, -79.50452850542926342, 2.999999999999997780 ) ) ;
#4462=CARTESIAN_POINT ( 'NONE',  ( 2.882544866740898382, -92.10452850542925773, 0.8366430509618999478 ) ) ;
#4463=CARTESIAN_POINT ( 'NONE',  ( -2.369498399071058969, -63.34547149457073800, 6.969112962950058332 ) ) ;
#4467=CARTESIAN_POINT ( 'NONE',  ( 1.719659006605284590, -67.84547149457071669, -4.969112962950050338 ) ) ;
#4468=CARTESIAN_POINT ( 'NONE',  ( -3.015831842038131150, -60.19547149457074653, 3.989209796945492048 ) ) ;
#4471=CARTESIAN_POINT ( 'NONE',  ( 3.015831842038232846, -67.80452850542926058, 3.989209796945429432 ) ) ;
#4473=CARTESIAN_POINT ( 'NONE',  ( 7.360235569667880284, -88.24547149457073658, 0.09995255151716216091 ) ) ;
#4476=CIRCLE ( 'NONE', #4349, 0.9999999999999948930 ) ;
#4480=CARTESIAN_POINT ( 'NONE',  ( -0.09506052544083960776, -81.00452850542926342, -4.999999999999997335 ) ) ;
#4481=CARTESIAN_POINT ( 'NONE',  ( 4.194503406049402194, -78.94547149457071100, 3.171033256558012159 ) ) ;
#4483=CARTESIAN_POINT ( 'NONE',  ( -0.8796985632579439329, -68.14547149457074227, -3.030887037049952326 ) ) ;
#4484=CARTESIAN_POINT ( 'NONE',  ( 2.179377348189480479, -65.85452850542924352, -7.030887037049986077 ) ) ;
#4485=CARTESIAN_POINT ( 'NONE',  ( 4.312004677471012570, -76.54547149457071953, -3.009306630940933314 ) ) ;
#4486=CARTESIAN_POINT ( 'NONE',  ( 4.194503406049334693, -62.55452850542925347, -3.171033256558100089 ) ) ;
#4489=CARTESIAN_POINT ( 'NONE',  ( 6.628020296210641149, -77.40452850542925489, -2.253526892787612645 ) ) ;
#4491=CARTESIAN_POINT ( 'NONE',  ( 2.610703060766947470, -91.54547149457074795, -1.773238653441125523 ) ) ;
#4495=CARTESIAN_POINT ( 'NONE',  ( 4.784657899331211439, -89.10452850542925773, 1.454677039711774533 ) ) ;
#4497=CARTESIAN_POINT ( 'NONE',  ( 4.312004677471076519, -76.95452850542925205, 3.009306630940844052 ) ) ;
#4498=CARTESIAN_POINT ( 'NONE',  ( 1.686450176301583337, -59.70452850542925916, -2.482926158054133303 ) ) ;
#4500=CARTESIAN_POINT ( 'NONE',  ( 0.09506052544086160405, -88.50452850542924921, 4.999999999999997335 ) ) ;
#4501=CARTESIAN_POINT ( 'NONE',  ( -4.037591185471546495, -65.29547149457073374, -5.718994135553860936 ) ) ;
#4502=CARTESIAN_POINT ( 'NONE',  ( 0.09506052544075677124, -88.99547149457073658, -4.999999999999997335 ) ) ;
#4503=CARTESIAN_POINT ( 'NONE',  ( 1.840261337453271251, -79.80452850542926058, 2.371175808195547852 ) ) ;
#4506=CARTESIAN_POINT ( 'NONE',  ( -2.823794231030019031, -90.90452850542926910, 1.017458915287783316 ) ) ;
#4507=CARTESIAN_POINT ( 'NONE',  ( -2.369498399071059414, -60.34547149457074511, 6.969112962950058332 ) ) ;
#4509=CARTESIAN_POINT ( 'NONE',  ( -1.719659006605266827, -69.34547149457073090, 4.969112962950051227 ) ) ;
#4510=CARTESIAN_POINT ( 'NONE',  ( 7.360235569667880284, -97.24547149457075079, 0.09995255151716216091 ) ) ;
#4514=CARTESIAN_POINT ( 'NONE',  ( 0.09506052544073574639, -88.99547149457075079, -6.999999999999997335 ) ) ;
#4517=CARTESIAN_POINT ( 'NONE',  ( 4.312004677471075631, -73.95452850542926626, 3.009306630940844496 ) ) ;
#4521=CARTESIAN_POINT ( 'NONE',  ( -5.257311121191324155, -80.74547149457075079, -0.09995255151718371311 ) ) ;
#4523=CARTESIAN_POINT ( 'NONE',  ( 2.322632124362881356, -96.99999999999992895, -3.314508707690180689 ) ) ;
#4524=CARTESIAN_POINT ( 'NONE',  ( -2.610703060766926153, -75.04547149457074795, 1.773238653441125745 ) ) ;
#4525=CARTESIAN_POINT ( 'NONE',  ( -6.686770931921506289, -72.60452850542924352, -2.072711028461647675 ) ) ;
#4527=CARTESIAN_POINT ( 'NONE',  ( -3.015831842038128485, -81.19547149457073942, 3.989209796945492048 ) ) ;
#4528=CARTESIAN_POINT ( 'NONE',  ( -4.194503406049320482, -61.05452850542923926, 3.171033256558100533 ) ) ;
#4529=CARTESIAN_POINT ( 'NONE',  ( -4.194503406049315153, -91.05452850542923215, 3.171033256558100533 ) ) ;
#4530=CARTESIAN_POINT ( 'NONE',  ( 4.037591185471441690, -65.70452850542925205, -5.718994135553947977 ) ) ;
#4531=CARTESIAN_POINT ( 'NONE',  ( -1.840261337453200641, -75.19547149457073942, 2.371175808195584267 ) ) ;
#4534=CARTESIAN_POINT ( 'NONE',  ( -2.862020680886582458, -59.29547149457074084, -4.100960146803977580 ) ) ;
#4535=CARTESIAN_POINT ( 'NONE',  ( 1.719659006605392060, -85.65452850542922647, 4.969112962950016588 ) ) ;
#4537=CARTESIAN_POINT ( 'NONE',  ( -3.015831842038214639, -78.30452850542926058, -3.989209796945429432 ) ) ;
#4538=CARTESIAN_POINT ( 'NONE',  ( 3.154386672714811990, -97.24547149457075079, 0.09995255151720662534 ) ) ;
#4539=CARTESIAN_POINT ( 'NONE',  ( -5.257311121191322378, -90.75452850542924921, 0.09995255151729526277 ) ) ;
#4540=CARTESIAN_POINT ( 'NONE',  ( 0.09506052544073198551, -58.99547149457073658, -6.999999999999997335 ) ) ;
#4541=CARTESIAN_POINT ( 'NONE',  ( -2.862020680886580237, -80.29547149457074795, -4.100960146803977580 ) ) ;
#4542=CARTESIAN_POINT ( 'NONE',  ( 2.882544866740896161, -74.10452850542924352, 0.8366430509618999478 ) ) ;
#4546=CARTESIAN_POINT ( 'NONE',  ( -2.882544866740876177, -84.60452850542927195, -0.8366430509618996147 ) ) ;
#4547=CARTESIAN_POINT ( 'NONE',  ( 6.013306294175172262, -94.95452850542926626, 4.245374608440616093 ) ) ;
#4549=CARTESIAN_POINT ( 'NONE',  ( 4.725907263620340082, -77.40452850542925489, -1.635492904037697981 ) ) ;
#4550=CARTESIAN_POINT ( 'NONE',  ( 2.862020680886598001, -63.79547149457074084, 4.100960146803977580 ) ) ;
#4554=CARTESIAN_POINT ( 'NONE',  ( 0.09506052544085819012, -61.50452850542925631, 4.999999999999997335 ) ) ;
#4556=CARTESIAN_POINT ( 'NONE',  ( 4.191402346623080533, -88.69547149457073942, -5.607243785695398941 ) ) ;
#4558=CARTESIAN_POINT ( 'NONE',  ( 3.015831842038234178, -79.80452850542926058, 3.989209796945429432 ) ) ;
#4559=CARTESIAN_POINT ( 'NONE',  ( -0.09506052544084034328, -75.00452850542924921, -4.999999999999997335 ) ) ;
#4563=CARTESIAN_POINT ( 'NONE',  ( 3.015831842038148913, -76.69547149457075363, -3.989209796945492048 ) ) ;
#4565=CARTESIAN_POINT ( 'NONE',  ( 3.154386672714807105, -61.24547149457073658, 0.09995255151720662534 ) ) ;
#4566=CARTESIAN_POINT ( 'NONE',  ( 6.686770931921523164, -71.10452850542924352, 2.072711028461649008 ) ) ;
#4568=CARTESIAN_POINT ( 'NONE',  ( 4.312004677471013459, -82.54547149457074795, -3.009306630940933314 ) ) ;
#4569=CARTESIAN_POINT ( 'NONE',  ( 4.725907263620339194, -59.40452850542926200, -1.635492904037697981 ) ) ;
#4570=CARTESIAN_POINT ( 'NONE',  ( 4.194503406049339134, -89.55452850542926058, -3.171033256558100089 ) ) ;
#4572=CARTESIAN_POINT ( 'NONE',  ( 6.013306294175168709, -67.95452850542925205, 4.245374608440616093 ) ) ;
#4573=CARTESIAN_POINT ( 'NONE',  ( 2.493201789345310004, -75.94547149457073942, 1.934965279058241006 ) ) ;
#4577=CARTESIAN_POINT ( 'NONE',  ( -2.862020680886493196, -85.20452850542925205, 4.100960146804039752 ) ) ;
#4579=CARTESIAN_POINT ( 'NONE',  ( 4.312004677471078296, -85.95452850542926626, 3.009306630940844052 ) ) ;
#4580=CARTESIAN_POINT ( 'NONE',  ( 1.069819614139496000, -91.84547149457074511, -2.969112962950042789 ) ) ;
#4582=CARTESIAN_POINT ( 'NONE',  ( 4.784657899331211439, -86.10452850542925773, 1.454677039711774533 ) ) ;
#4584=CARTESIAN_POINT ( 'NONE',  ( -6.628020296210668683, -62.59547149457074511, -2.253526892787471869 ) ) ;
#4585=CARTESIAN_POINT ( 'NONE',  ( -2.493201789345253605, -64.05452850542924637, 1.934965279058294518 ) ) ;
#4588=CARTESIAN_POINT ( 'NONE',  ( -1.840261337453250823, -84.30452850542926058, -2.371175808195547852 ) ) ;
#4589=CARTESIAN_POINT ( 'NONE',  ( -2.179377348189459163, -94.35452850542925773, 7.030887037049988741 ) ) ;
#4592=CARTESIAN_POINT ( 'NONE',  ( 4.725907263620340970, -80.40452850542925489, -1.635492904037697981 ) ) ;
#4593=CARTESIAN_POINT ( 'NONE',  ( -6.013306294175058575, -87.04547149457074795, 4.245374608440741326 ) ) ;
#4595=CARTESIAN_POINT ( 'NONE',  ( -54.99999999999999289, -97.00000000000000000, 20.00000000000000000 ) ) ;
#4596=CARTESIAN_POINT ( 'NONE',  ( 1.840261337453219515, -70.69547149457073942, -2.371175808195584267 ) ) ;
#4597=CARTESIAN_POINT ( 'NONE',  ( -4.312004677471061420, -57.45452850542925916, -3.009306630940844052 ) ) ;
#4598=CARTESIAN_POINT ( 'NONE',  ( -2.179377348189609265, -86.14547149457072805, -7.030887037049939003 ) ) ;
#4601=CARTESIAN_POINT ( 'NONE',  ( 1.719659006605391394, -79.65452850542925489, 4.969112962950016588 ) ) ;
#4604=CARTESIAN_POINT ( 'NONE',  ( 5.257311121191341918, -79.24547149457075079, 0.09995255151718437925 ) ) ;
#4606=CARTESIAN_POINT ( 'NONE',  ( 2.823794231030057666, -61.09547149457074511, 1.017458915287723809 ) ) ;
#4607=CARTESIAN_POINT ( 'NONE',  ( 5.895805022753406455, -74.55452850542926058, -4.407101234057908989 ) ) ;
#4609=CARTESIAN_POINT ( 'NONE',  ( -3.015831842038129373, -75.19547149457073942, 3.989209796945492048 ) ) ;
#4611=CARTESIAN_POINT ( 'NONE',  ( -1.529537955723668574, -88.35452850542925773, 5.030887037049979860 ) ) ;
#4612=CARTESIAN_POINT ( 'NONE',  ( 2.179377348189481367, -71.85452850542924352, -7.030887037049986077 ) ) ;
#4613=CARTESIAN_POINT ( 'NONE',  ( -2.823794231030039903, -80.59547149457075932, -1.017458915287723364 ) ) ;
#4614=AXIS2_PLACEMENT_3D ( 'NONE', #3117, #5173, #6945 ) ;
#4619=CARTESIAN_POINT ( 'NONE',  ( -1.529537955723667908, -94.35452850542922931, 5.030887037049979860 ) ) ;
#4620=CARTESIAN_POINT ( 'NONE',  ( 4.312004677471078296, -85.95452850542925205, 3.009306630940844496 ) ) ;
#4622=CARTESIAN_POINT ( 'NONE',  ( -0.09506052544083960776, -81.00452850542926342, -4.999999999999997335 ) ) ;
#4623=CARTESIAN_POINT ( 'NONE',  ( -2.823794231030038571, -92.59547149457074511, -1.017458915287723364 ) ) ;
#4626=CARTESIAN_POINT ( 'NONE',  ( -3.015831842038213750, -87.30452850542926058, -3.989209796945429432 ) ) ;
#4627=CARTESIAN_POINT ( 'NONE',  ( -0.09506052544071605381, -60.49547149457073658, 6.999999999999997335 ) ) ;
#4628=CARTESIAN_POINT ( 'NONE',  ( 3.154386672714807105, -62.25452850542926342, -0.09995255151727241993 ) ) ;
#4633=CARTESIAN_POINT ( 'NONE',  ( -2.493201789345251829, -79.05452850542926058, 1.934965279058294518 ) ) ;
#4634=CARTESIAN_POINT ( 'NONE',  ( -4.191402346623177344, -90.30452850542926058, -5.607243785695311900 ) ) ;
#4637=CARTESIAN_POINT ( 'NONE',  ( 6.628020296210689111, -91.09547149457074511, 2.253526892787472757 ) ) ;
#4640=CARTESIAN_POINT ( 'NONE',  ( 1.686450176301635517, -72.79547149457074795, 2.482926158054096000 ) ) ;
#4642=CARTESIAN_POINT ( 'NONE',  ( 5.257311121191341918, -62.25452850542924921, -0.09995255151729465215 ) ) ;
#4644=CARTESIAN_POINT ( 'NONE',  ( -4.784657899331190123, -72.60452850542925773, -1.454677039711773867 ) ) ;
#4645=CARTESIAN_POINT ( 'NONE',  ( 7.360235569667877620, -76.24547149457073658, 0.09995255151716216091 ) ) ;
#4648=CARTESIAN_POINT ( 'NONE',  ( -4.194503406049316929, -76.05452850542926058, 3.171033256558100533 ) ) ;
#4651=CARTESIAN_POINT ( 'NONE',  ( -0.09506052544073503863, -78.49547149457073658, 4.999999999999997335 ) ) ;
#4653=CARTESIAN_POINT ( 'NONE',  ( -2.882544866740859746, -62.89547149457074227, 0.8366430509619596778 ) ) ;
#4654=CARTESIAN_POINT ( 'NONE',  ( 0.09506052544088061662, -70.50452850542926342, 6.999999999999997335 ) ) ;
#4656=CARTESIAN_POINT ( 'NONE',  ( -4.194503406049384431, -74.44547149457071100, -3.171033256558012159 ) ) ;
#4657=CARTESIAN_POINT ( 'NONE',  ( -0.09506052544083921918, -84.00452850542926342, -4.999999999999997335 ) ) ;
#4658=CARTESIAN_POINT ( 'NONE',  ( -2.369498399071207739, -66.15452850542925489, -6.969112962950009482 ) ) ;
#4659=CARTESIAN_POINT ( 'NONE',  ( 1.069819614139495112, -82.84547149457074511, -2.969112962950042789 ) ) ;
#4663=CARTESIAN_POINT ( 'NONE',  ( -4.725907263620318766, -93.90452850542925489, 1.635492904037698647 ) ) ;
#4664=CARTESIAN_POINT ( 'NONE',  ( 5.257311121191342806, -92.25452850542922079, -0.09995255151729465215 ) ) ;
#4666=CARTESIAN_POINT ( 'NONE',  ( 0.09506052544085971667, -73.50452850542924921, 4.999999999999997335 ) ) ;
#4667=CARTESIAN_POINT ( 'NONE',  ( 0.8796985632579631398, -87.64547149457075648, 3.030887037049952326 ) ) ;
#4668=CARTESIAN_POINT ( 'NONE',  ( -4.784657899331189235, -87.60452850542925773, -1.454677039711773867 ) ) ;
#4669=CARTESIAN_POINT ( 'NONE',  ( 2.179377348189484476, -95.85452850542924352, -7.030887037049986077 ) ) ;
#4670=CARTESIAN_POINT ( 'NONE',  ( 2.610703060766983441, -70.95452850542925205, 1.773238653441072232 ) ) ;
#4674=CARTESIAN_POINT ( 'NONE',  ( -2.493201789345251385, -82.05452850542926058, 1.934965279058294518 ) ) ;
#4675=CARTESIAN_POINT ( 'NONE',  ( -4.037591185471422150, -85.20452850542925205, 5.718994135553947977 ) ) ;
#4676=CARTESIAN_POINT ( 'NONE',  ( -0.09506052544071266763, -87.49547149457075079, 6.999999999999997335 ) ) ;
#4679=CARTESIAN_POINT ( 'NONE',  ( -2.610703060766926598, -72.04547149457074795, 1.773238653441125745 ) ) ;
#4682=CARTESIAN_POINT ( 'NONE',  ( 1.719659006605389839, -70.65452850542926910, 4.969112962950016588 ) ) ;
#4683=CARTESIAN_POINT ( 'NONE',  ( 7.360235569667877620, -79.24547149457073658, 0.09995255151716216091 ) ) ;
#4686=CARTESIAN_POINT ( 'NONE',  ( -2.862020680886494528, -76.20452850542926626, 4.100960146804039752 ) ) ;
#4691=CARTESIAN_POINT ( 'NONE',  ( 1.529537955723795140, -72.64547149457075648, 5.030887037049945221 ) ) ;
#4693=CARTESIAN_POINT ( 'NONE',  ( -0.09506052544073276267, -96.49547149457075079, 4.999999999999997335 ) ) ;
#4694=CARTESIAN_POINT ( 'NONE',  ( -4.037591185471424815, -61.20452850542925916, 5.718994135553947977 ) ) ;
#4698=CARTESIAN_POINT ( 'NONE',  ( 4.312004677471076519, -82.95452850542925205, 3.009306630940844496 ) ) ;
#4699=CARTESIAN_POINT ( 'NONE',  ( 6.013306294175168709, -70.95452850542925205, 4.245374608440616093 ) ) ;
#4700=ADVANCED_FACE ( 'NONE', ( #1271 ), #1310, .T. ) ;
#4702=CARTESIAN_POINT ( 'NONE',  ( -0.09506052544075634103, -78.49547149457075079, 2.999999999999997780 ) ) ;
#4706=CARTESIAN_POINT ( 'NONE',  ( -5.257311121191323267, -81.75452850542926342, 0.09995255151729526277 ) ) ;
#4707=VERTEX_POINT ( 'NONE', #3840 ) ;
#4708=CARTESIAN_POINT ( 'NONE',  ( 1.529537955723689446, -68.85452850542924352, -5.030887037049978971 ) ) ;
#4709=CARTESIAN_POINT ( 'NONE',  ( -2.610703060766924821, -87.04547149457074795, 1.773238653441125745 ) ) ;
#4710=CARTESIAN_POINT ( 'NONE',  ( -0.8796985632579451542, -59.14547149457074227, -3.030887037049952326 ) ) ;
#4711=CARTESIAN_POINT ( 'NONE',  ( -7.360235569667856304, -93.75452850542926342, 0.09995255151731782806 ) ) ;
#4712=CARTESIAN_POINT ( 'NONE',  ( -2.823794231030022139, -69.90452850542925489, 1.017458915287783316 ) ) ;
#4716=CARTESIAN_POINT ( 'NONE',  ( 1.840261337453270585, -73.80452850542926058, 2.371175808195547852 ) ) ;
#4717=CARTESIAN_POINT ( 'NONE',  ( -6.628020296210619833, -90.90452850542926910, 2.253526892787613978 ) ) ;
#4718=CARTESIAN_POINT ( 'NONE',  ( 6.013306294175080779, -85.54547149457074795, -4.245374608440741326 ) ) ;
#4721=CARTESIAN_POINT ( 'NONE',  ( 1.069819614139493558, -70.84547149457073090, -2.969112962950042789 ) ) ;
#4725=CARTESIAN_POINT ( 'NONE',  ( 0.09506052544085895339, -67.50452850542926342, 4.999999999999997335 ) ) ;
#4726=CARTESIAN_POINT ( 'NONE',  ( -4.191402346623057440, -81.19547149457073942, 5.607243785695398941 ) ) ;
#4729=CARTESIAN_POINT ( 'NONE',  ( -1.529537955723671683, -67.35452850542925773, 5.030887037049979860 ) ) ;
#4732=CARTESIAN_POINT ( 'NONE',  ( 4.725907263620372056, -70.09547149457074511, 1.635492904037598283 ) ) ;
#4734=CARTESIAN_POINT ( 'NONE',  ( -2.823794231030042123, -62.59547149457074511, -1.017458915287723364 ) ) ;
#4735=CARTESIAN_POINT ( 'NONE',  ( 0.09506052544087911782, -58.50452850542925631, 6.999999999999997335 ) ) ;
#4739=CARTESIAN_POINT ( 'NONE',  ( -1.719659006605370744, -90.15452850542922647, -4.969112962950016588 ) ) ;
#4740=CARTESIAN_POINT ( 'NONE',  ( 1.069819614139494002, -73.84547149457073090, -2.969112962950042789 ) ) ;
#4743=CARTESIAN_POINT ( 'NONE',  ( 3.015831842038233734, -76.80452850542926058, 3.989209796945429432 ) ) ;
#4744=ORIENTED_EDGE ( 'NONE', *, *, #3884, .T. ) ;
#4745=CARTESIAN_POINT ( 'NONE',  ( -4.784657899331191011, -69.60452850542925773, -1.454677039711773867 ) ) ;
#4746=CARTESIAN_POINT ( 'NONE',  ( 3.154386672714811102, -91.24547149457073658, 0.09995255151720662534 ) ) ;
#4747=CARTESIAN_POINT ( 'NONE',  ( -2.882544866740859746, -59.89547149457074937, 0.8366430509619596778 ) ) ;
#4748=CARTESIAN_POINT ( 'NONE',  ( -1.529537955723670350, -76.35452850542925773, 5.030887037049979860 ) ) ;
#4749=CARTESIAN_POINT ( 'NONE',  ( -7.360235569667856304, -90.75452850542924921, 0.09995255151731782806 ) ) ;
#4752=CARTESIAN_POINT ( 'NONE',  ( -2.610703060766966566, -66.45452850542925205, -1.773238653441072232 ) ) ;
#4757=DIRECTION ( 'NONE',  ( -1.051676107310939774E-14, -1.326812532709957139E-30, -1.000000000000000000 ) ) ;
#4758=CARTESIAN_POINT ( 'NONE',  ( 2.882544866740897049, -77.10452850542924352, 0.8366430509618999478 ) ) ;
#4760=CARTESIAN_POINT ( 'NONE',  ( 4.037591185471445243, -92.70452850542926626, -5.718994135553947977 ) ) ;
#4762=CARTESIAN_POINT ( 'NONE',  ( 5.895805022753496161, -78.94547149457073942, 4.407101234057782868 ) ) ;
#4765=CARTESIAN_POINT ( 'NONE',  ( 2.823794231030058111, -64.09547149457071669, 1.017458915287723809 ) ) ;
#4766=CIRCLE ( 'NONE', #2223, 0.9999999999999948930 ) ;
#4772=CARTESIAN_POINT ( 'NONE',  ( -1.529537955723671239, -70.35452850542925773, 5.030887037049979860 ) ) ;
#4773=CARTESIAN_POINT ( 'NONE',  ( 2.369498399071078065, -79.84547149457074511, -6.969112962950057444 ) ) ;
#4774=SURFACE_SIDE_STYLE ('',( #5406 ) ) ;
#4776=CARTESIAN_POINT ( 'NONE',  ( -2.862020680886580681, -74.29547149457074795, -4.100960146803977580 ) ) ;
#4777=CARTESIAN_POINT ( 'NONE',  ( 3.015831842038232402, -64.80452850542926058, 3.989209796945429432 ) ) ;
#4779=( BOUNDED_SURFACE ( )  B_SPLINE_SURFACE ( 3, 2, ( 
 ( #1697, #3037, #7067, #4295, #614, #3908, #697, #5750, #6238, #6867, #3629, #1097, #4332, #7469, #4254, #8143, #2605, #4934, #8332, #5561, #6908, #3669, #6824, #2372, #7547, #1144, #6283, #7702, #1978, #1295, #5794, #3865, #22, #4529, #6195, #5524, #8104, #7155, #1547, #4739, #2735, #3948, #7835, #4570, #5840, #5295, #3368, #829, #110, #3447, #3991, #4611, #2021, #6601, #68, #5377, #7879, #2062, #1378, #3408, #5252, #6519, #3323, #2651, #1504, #6559, #7789, #5971, #6682, #872, #743, #2104, #5881, #5208, #2694, #7198, #5335, #2776, #1423, #7918, #4657, #197, #2144, #4072, #5928, #786, #6011, #4698, #3280, #235, #155, #7239, #1462, #4034, #7278, #6642, #2814, #7960, #2185, #7319, #4113, #279, #2857, #5420, #6054, #913, #3484, #5958, #7185, #4601, #144, #5153, #3981, #3400, #7866, #3353, #5782, #820, #3897, #2007, #2681, #185, #1452, #2725, #7268, #5283, #2094, #3225, #3312, #7735, #3937, #732, #4686, #4648, #5868, #5239, #6549, #1495, #99, #10, #4559, #1967, #2767, #1368, #7097, #4021, #686, #4517, #1323, #6505, #7230, #7778, #775, #4063, #642, #5916, #7823, #5198, #6466, #7143, #2052, #2590, #3267, #5823, #5328, #57, #6593, #2641, #1411, #7909, #2135, #4105, #6716, #2849, #905, #6673, #6167, #351, #1666, #8075, #269, #4867, #7951, #2305, #7309, #2176, #4910, #8116, #6086, #1535, #5410, #4729, #859, #311, #947, #4186, #3476, #6799, #7353, #7990, #5366, #1626, #3439, #392, #2889, #2219, #6043, #6757, #4777, #1580, #4146, #6002, #7438, #3518, #2806, #228, #5456, #8035, #2262, #4818, #7397, #2969, #2929, #4229, #1030, #989, #3599, #3557, #5534, #6126, #5494, #7481, #2341, #1709, #6630, #475, #5573, #6838, #6295, #4346, #1836, #1110, #4424, #4985, #5613, #3007, #7601, #1070, #6376, #3725, #3051, #8155, #4387, #6254, #2384, #4307, #3644, #2503, #7559, #433, #6963 ),
 ( #6338, #3766, #8192, #556, #513, #1195, #3134, #5064, #6923, #4944, #1876, #1235, #2463, #8232, #5689, #7518, #8273, #7008, #7643, #3806, #6209, #597, #1749, #2422, #3092, #3176, #5731, #8312, #2542, #5106, #7684, #6879, #1157, #3682, #1791, #5652, #4265, #5024, #2332, #6240, #1655, #341, #3631, #6788, #2294, #1780, #1146, #6115, #4936, #4215, #5563, #1615, #6910, #4256, #8145, #4897, #1021, #7509, #2374, #465, #3588, #1739, #6077, #2252, #4177, #4807, #6869, #4297, #3040, #8106, #6198, #6748, #4336, #1100, #4855, #3545, #423, #2411, #2959, #2918, #7549, #3672, #6826, #5602, #8183, #7429, #4974, #6156, #978, #2997, #1059, #301, #7471, #5484, #2878, #5445, #8025, #381, #7383, #5526, #8063, #1700, #8263, #8302, #6952, #5680, #2452, #8223, #4503, #503, #4457, #4377, #1228, #3124, #2534, #3880, #3081, #7039, #5723, #7589, #5183, #5096, #2023, #7125, #5056, #3715, #5644, #5014, #6369, #626, #7676, #1993, #1908, #6450, #7632, #6328, #1268, #4415, #2495, #7762, #6285, #3755, #2576, #1867, #3209, #1825, #4542, #3839, #5765, #6409, #6997, #5137, #7716, #671, #3798, #1952, #1186, #547, #588, #3168, #7082, #1308, #3252, #5808, #37, #2623, #5392, #4670, #5854, #82, #6657, #756, #7213, #7932, #4712, #886, #3384, #3460, #127, #6024, #6534, #7892, #249, #2664, #2749, #1479, #5941, #1437, #2830, #5223, #1391, #711, #7973, #4004, #7804, #2198, #7251, #4752, #209, #3298, #4047, #7290, #2118, #3422, #1352, #2708, #2788, #5895, #2037, #6615, #841, #3923, #169, #4585, #6490, #7168, #3964, #6574, #2159, #5268, #5986, #3337, #7849, #5310, #2075, #4628, #803, #5348, #1517, #4085, #8095, #8015, #4842, #6737, #6144, #7499, #6694, #2321, #1010, #2868, #454, #3577, #3619, #2402, #331, #7334, #924, #4125, #1644, #4247, #370, #5591, #2946, #1730, #2909, #1600, #4885, #8054, #3536, #3028, #1560 ),
 ( #5514, #2280, #6187, #413, #4285, #5474, #2986, #8172, #3496, #5434, #6067, #8134, #5553, #6859, #7459, #1688, #2241, #292, #6817, #4797, #7372, #1089, #967, #7420, #2364, #4927, #3660, #1050, #6229, #6105, #4166, #4204, #6777, #3867, #1134, #6358, #5084, #1218, #5046, #7069, #6274, #5003, #4324, #4491, #7620, #3069, #1297, #8292, #5796, #3827, #6897, #2520, #4447, #3743, #2441, #7664, #6436, #1854, #1814, #656, #3704, #5752, #1769, #5711, #5631, #2484, #4367, #3787, #5127, #492, #1898, #6985, #8212, #3239, #575, #1255, #24, #6315, #4961, #7575, #6941, #4404, #7027, #3157, #7539, #6398, #7704, #536, #1175, #616, #5669, #3114, #8251, #3197, #8334, #2566, #1937, #2106, #6479, #3449, #788, #4659, #7201, #3326, #1465, #7241, #5337, #745, #6604, #6013, #7112, #699, #1340, #3410, #4037, #2778, #4613, #2737, #3282, #6644, #5930, #3911, #5843, #7920, #2024, #112, #831, #5973, #2147, #1425, #4702, #1380, #7280, #7791, #3371, #1506, #71, #3993, #5297, #6562, #2697, #4074, #2653, #5210, #1980, #874, #5255, #4573, #2607, #157, #5170, #199, #4531, #7882, #7748, #3950, #7157, #6522, #5883, #7837, #2064, #4740, #2187, #7962, #237, #2816, #5381, #7301, #4640, #3975, #5996, #3432, #1569, #4679, #766, #7982, #4135, #5234, #5952, #895, #7222, #4721, #4596, #1446, #7260, #3347, #2085, #7179, #4014, #1404, #218, #7817, #2209, #7903, #6584, #6544, #2800, #814, #5906, #138, #2677, #6666, #3394, #2719, #5359, #3508, #6035, #5277, #1488, #7859, #2048, #178, #2761, #2168, #7942, #5320, #1528, #2127, #4098, #3469, #260, #4056, #6624, #2841, #5401, #851, #4765, #7345, #6703, #936, #93, #6690, #964, #921, #6141, #1515, #5471, #4162, #6021, #3616, #6734, #6771, #5550, #3493, #2156, #4082, #7288, #4794, #7417, #3532, #410, #6100, #2318, #6064, #4747, #8050, #2865, #288, #6184, #4710, #2195 ),
 ( #5428, #1007, #3573, #4882, #8011, #366, #2983, #6655, #245, #884, #2943, #5510, #7454, #327, #2277, #2826, #3457, #4838, #5389, #7970, #1684, #1557, #2238, #8092, #4244, #6813, #2906, #1046, #7368, #7331, #4122, #1641, #1597, #4201, #1172, #8247, #4364, #8208, #1894, #1086, #8169, #7495, #7661, #2438, #6226, #4444, #3111, #5000, #4282, #5708, #5081, #6311, #3740, #7616, #6855, #5666, #2517, #5628, #3784, #6938, #1851, #3025, #1127, #1809, #7024, #572, #4401, #6395, #6980, #1214, #2361, #7572, #3657, #3066, #532, #3823, #6354, #3152, #8288, #2480, #1251, #5043, #4923, #3701, #448, #612, #489, #5588, #3193, #2398, #4958, #7535, #8131, #1724, #6894, #1766, #4321, #6271, #3321, #6475, #1976, #1293, #1334, #4568, #2562, #7700, #20, #2734, #5165, #108, #5792, #7153, #4527, #5123, #3235, #5838, #7108, #2602, #7744, #5292, #7833, #785, #7196, #3906, #3989, #7065, #1420, #6432, #3863, #4145, #7237, #5206, #651, #695, #3278, #8330, #7787, #66, #5878, #2649, #5926, #2018, #1376, #4485, #741, #1932, #7877, #3946, #6517, #2693, #5250, #2061, #4609, #6557, #3366, #152, #2103, #4656, #1579, #946, #6715, #5748, #2340, #8034, #310, #1625, #6125, #5571, #3006, #4866, #8154, #2968, #6208, #432, #4306, #350, #474, #2928, #2383, #3555, #4908, #8074, #2887, #988, #3598, #2304, #5493, #7437, #3050, #4943, #6878, #7517, #1665, #1748, #4817, #1109, #4185, #7395, #1790, #4984, #5533, #6756, #4227, #6798, #6085, #8115, #6166, #1069, #1029, #3681, #391, #7480, #2261, #6837, #5455, #5612, #1708, #4264, #3643, #6252, #8191, #2421, #7558, #4345, #6921, #3517, #5651, #7047, #4550, #7089, #8231, #8311, #2462, #6294, #7599, #3765, #3217, #633, #2502, #5774, #596, #3846, #6415, #1960, #1234, #5023, #1316, #6459, #7683, #5105, #4, #1835, #4468, #3888, #7007, #5146, #2541, #2583, #4386, #5063, #3175 ),
 ( #6962, #4423, #3805, #5191, #7725, #4510, #680, #1277, #2632, #6375, #3724, #7642, #1194, #3260, #1875, #6337, #5816, #555, #3133, #5688, #5730, #46, #8271, #7769, #2000, #1156, #512, #1916, #3091, #2674, #2716, #5949, #3930, #721, #7939, #5992, #7298, #811, #7257, #5231, #2837, #2123, #3305, #5861, #4095, #6541, #4637, #5355, #2165, #6663, #3391, #892, #5903, #3466, #3972, #5317, #6032, #90, #175, #1485, #2757, #7219, #256, #7813, #7175, #6498, #5398, #1443, #2045, #7979, #4676, #2205, #215, #4593, #4053, #6621, #134, #1401, #848, #7134, #4011, #763, #1361, #4718, #7900, #3429, #3344, #5274, #2796, #7855, #2082, #1525, #6581, #6237, #1017, #5441, #4294, #462, #1566, #2290, #5560, #3542, #1056, #933, #975, #3585, #8022, #6744, #3504, #6074, #8142, #4132, #5523, #2249, #6112, #6152, #338, #420, #6700, #8103, #6785, #298, #3036, #378, #3628, #8180, #2915, #4762, #2875, #4804, #7426, #1696, #2955, #5599, #2329, #4933, #5481, #7380, #4893, #8060, #4851, #7341, #1611, #4173, #6194, #1652, #4253, #4212, #7468, #6823, #2993, #2371, #7506, #1736, #6866, #1096, #3668, #6407, #3250, #6907, #6282, #1143, #1226, #1906, #5642, #3752, #4412, #7714, #3207, #4455, #668, #7037, #1266, #4971, #5054, #3712, #5678, #2493, #6446, #624, #3837, #5761, #2531, #3878, #7629, #7546, #6326, #501, #5135, #3122, #3078, #2686, #2450, #8221, #5012, #8261, #2574, #1184, #5721, #5806, #2409, #8300, #1865, #6950, #7586, #545, #3796, #1777, #4331, #1823, #1950, #4375, #5093, #6995, #6367, #586, #3166, #7674, #4501, #7080, #1306, #81, #7931, #2116, #3420, #1477, #2036, #6614, #1350, #4046, #710, #3921, #6656, #1516, #7848, #3297, #4584, #6489, #2621, #2074, #125, #5940, #5222, #208, #755, #1390, #7122, #3383, #5180, #2158, #4627, #7167, #5853, #168, #3962, #2663, #7802, #7760, #840, #3336, #4540 ),
 ( #6533, #4669, #7891, #5894, #7250, #7211, #2747, #5309, #5985, #2707, #5267, #2787, #5346, #6573, #4003, #4711, #1436, #7289, #4083, #801, #885, #3459, #35, #1991, #7498, #2829, #3534, #6816, #4796, #2320, #2197, #2240, #2279, #923, #8013, #4749, #7333, #1048, #5391, #6773, #6692, #7370, #4841, #1599, #1686, #7972, #1009, #8052, #1559, #1727, #7419, #4884, #1088, #4165, #6023, #4124, #3495, #330, #2945, #1643, #4284, #4203, #6186, #6736, #290, #3576, #966, #6102, #6858, #247, #6066, #7456, #2908, #5513, #2867, #5431, #6143, #8094, #368, #5473, #4246, #3618, #412, #2985, #5552, #8133, #2363, #4925, #2401, #4446, #2519, #3825, #5668, #3786, #7538, #7703, #6982, #8171, #4960, #615, #3068, #1174, #1897, #7026, #3196, #8249, #5751, #2440, #8333, #491, #1853, #2565, #1768, #5045, #6357, #2482, #3742, #5126, #4323, #3703, #3027, #1936, #6313, #6896, #4489, #1217, #7068, #5083, #5590, #574, #3154, #5002, #1129, #5710, #3659, #535, #5630, #6228, #1254, #4403, #8291, #450, #7574, #7663, #8211, #6273, #6397, #1811, #4366, #6940, #3113, #7619, #2105, #6435, #2063, #1979, #5841, #111, #69, #5296, #654, #4612, #3324, #5168, #2777, #5882, #5929, #4699, #2652, #1296, #3238, #5795, #3949, #6560, #2695, #7919, #5254, #1463, #5209, #3910, #7199, #2022, #7790, #5336, #3866, #1337, #156, #4572, #787, #7747, #2145, #7836, #3369, #1424, #7156, #2736, #7880, #4035, #1379, #4658, #23, #2606, #4530, #7111, #7240, #6603, #830, #3992, #3409, #6478, #698, #5972, #3281, #6520, #198, #744, #873, #5378, #7961, #2186, #3448, #7279, #6012, #1505, #236, #2815, #4073, #6643, #8258, #6994, #3121, #6949, #623, #8179, #6904, #6235, #6406, #1183, #4970, #3205, #1864, #7713, #5720, #461, #4411, #6366, #5641, #4330, #1225, #5760, #3750, #3711, #2828, #4454, #7628, #584, #2573, #8220, #8299, #3077, #2408 ),
 ( #4374, #7673, #2449, #3165, #3035, #5010, #5677, #1775, #7583, #2530, #5598, #3795, #544, #7545, #5134, #2492, #5092, #1947, #1822, #6865, #1142, #3667, #6325, #1905, #5053, #1095, #7036, #1263, #3836, #6281, #500, #5221, #709, #207, #7930, #4539, #3382, #2662, #4002, #34, #5345, #2706, #6572, #754, #7801, #5939, #799, #7249, #2034, #166, #4500, #667, #2618, #3249, #5308, #2746, #4668, #6532, #4626, #5179, #2786, #7846, #5805, #7759, #1475, #3920, #4582, #7890, #2115, #4045, #3335, #6613, #3293, #839, #1349, #5265, #3419, #1990, #5893, #7210, #123, #7166, #5984, #7121, #6488, #3877, #7079, #1389, #5852, #1305, #2073, #6445, #80, #3961, #1435, #1360, #7812, #5190, #1558, #3304, #2631, #3929, #3887, #8012, #4592, #5815, #7332, #4839, #7369, #45, #246, #7768, #6458, #1999, #6497, #3494, #922, #2673, #6065, #762, #4123, #6691, #2239, #1400, #4549, #1598, #6735, #7971, #5390, #289, #7133, #4748, #4163, #7174, #5430, #5230, #720, #965, #2044, #5860, #4795, #89, #3971, #6540, #3458, #2866, #6022, #3533, #8051, #5472, #6101, #2827, #2196, #329, #2907, #2278, #679, #3259, #1315, #4365, #6815, #1767, #7455, #449, #3617, #6772, #4883, #7497, #6185, #1685, #4245, #6939, #1128, #2439, #490, #1047, #5629, #367, #3067, #8093, #2944, #5667, #533, #6856, #2319, #411, #5511, #1642, #1087, #1726, #4959, #2984, #7573, #8132, #5551, #6142, #2400, #7418, #8248, #2362, #4924, #4283, #7536, #3658, #6227, #3026, #4202, #8209, #5589, #3575, #4322, #2481, #5001, #8170, #6895, #3702, #1008, #6272, #1810, #1173, #3741, #6312, #3112, #4486, #7745, #1977, #5839, #5124, #1215, #2650, #2020, #3236, #652, #4528, #3785, #21, #7788, #2563, #696, #3864, #7109, #8290, #6396, #7066, #4569, #67, #1335, #3322, #3907, #6476, #7618, #7701, #6355, #8331, #1934, #742, #3279, #5207, #7154, #5166, #6518 ) ),
 .UNSPECIFIED., .T., .F., .T. ) 
 B_SPLINE_SURFACE_WITH_KNOTS ( ( 4, 3, 4 ),
 ( 3, 2, 2, 2, 2, 2, 2, 2, 2, 2, 2, 2, 2, 2, 2, 2, 2, 2, 2, 2, 2, 2, 2, 2, 2, 2, 2, 2, 2, 2, 2, 2, 2, 2, 2, 2, 2, 2, 2, 2, 2, 2, 2, 2, 2, 2, 2, 2, 2, 2, 2, 2, 2, 2, 2, 2, 2, 2, 2, 2, 2, 2, 2, 2, 2, 2, 2, 2, 2, 2, 2, 2, 2, 2, 2, 2, 2, 2, 2, 2, 2, 2, 2, 2, 2, 2, 2, 2, 2, 2, 2, 2, 2, 2, 2, 2, 2, 2, 2, 2, 2, 2, 2, 2, 2, 2, 2, 2, 2, 2, 2, 2, 2, 2, 2, 2, 2, 2, 2, 2, 2, 2, 2, 2, 2, 2, 2, 2, 2, 2, 3 ),
 ( 0.000000000000000000, 0.5000000000000000000, 1.000000000000000000 ),
 ( 0.000000000000000000, 0.007692307692307692735, 0.01538461538461538547, 0.02307692307692307820, 0.03076923076923077094, 0.03846153846153846367, 0.04615384615384615641, 0.05384615384615384914, 0.06153846153846154188, 0.06923076923076923461, 0.07692307692307692735, 0.08461538461538462008, 0.09230769230769231282, 0.1000000000000000056, 0.1076923076923076983, 0.1153846153846153910, 0.1230769230769230838, 0.1307692307692307765, 0.1384615384615384692, 0.1461538461538461620, 0.1538461538461538547, 0.1615384615384615474, 0.1692307692307692402, 0.1769230769230769329, 0.1846153846153846256, 0.1923076923076923184, 0.2000000000000000111, 0.2076923076923077038, 0.2153846153846153966, 0.2230769230769230893, 0.2307692307692307820, 0.2384615384615384748, 0.2461538461538461675, 0.2538461538461538325, 0.2615384615384615530, 0.2692307692307692180, 0.2769230769230769384, 0.2846153846153846034, 0.2923076923076923239, 0.2999999999999999889, 0.3076923076923077094, 0.3153846153846153744, 0.3230769230769230949, 0.3307692307692307598, 0.3384615384615384803, 0.3461538461538461453, 0.3538461538461538658, 0.3615384615384615308, 0.3692307692307692513, 0.3769230769230769162, 0.3846153846153846367, 0.3923076923076923017, 0.4000000000000000222, 0.4076923076923076872, 0.4153846153846154077, 0.4230769230769230727, 0.4307692307692307931, 0.4384615384615384581, 0.4461538461538461786, 0.4538461538461538436, 0.4615384615384615641, 0.4692307692307692291, 0.4769230769230769496, 0.4846153846153846145, 0.4923076923076923350, 0.5000000000000000000, 0.5076923076923076650, 0.5153846153846153300, 0.5230769230769231060, 0.5307692307692307709, 0.5384615384615384359, 0.5461538461538461009, 0.5538461538461538769, 0.5615384615384615419, 0.5692307692307692069, 0.5769230769230768718, 0.5846153846153846478, 0.5923076923076923128, 0.5999999999999999778, 0.6076923076923076428, 0.6153846153846154188, 0.6230769230769230838, 0.6307692307692307487, 0.6384615384615384137, 0.6461538461538461897, 0.6538461538461538547, 0.6615384615384615197, 0.6692307692307691847, 0.6769230769230769607, 0.6846153846153846256, 0.6923076923076922906, 0.6999999999999999556, 0.7076923076923077316, 0.7153846153846153966, 0.7230769230769230616, 0.7307692307692307265, 0.7384615384615385025, 0.7461538461538461675, 0.7538461538461538325, 0.7615384615384614975, 0.7692307692307692735, 0.7769230769230769384, 0.7846153846153846034, 0.7923076923076922684, 0.8000000000000000444, 0.8076923076923077094, 0.8153846153846153744, 0.8230769230769230393, 0.8307692307692308153, 0.8384615384615384803, 0.8461538461538461453, 0.8538461538461538103, 0.8615384615384615863, 0.8692307692307692513, 0.8769230769230769162, 0.8846153846153845812, 0.8923076923076923572, 0.9000000000000000222, 0.9076923076923076872, 0.9153846153846153522, 0.9230769230769231282, 0.9307692307692307931, 0.9384615384615384581, 0.9461538461538461231, 0.9538461538461538991, 0.9615384615384615641, 0.9692307692307692291, 0.9769230769230768940, 0.9846153846153846700, 0.9923076923076923350, 1.000000000000000000 ),
 .UNSPECIFIED. ) 
 GEOMETRIC_REPRESENTATION_ITEM ( )  RATIONAL_B_SPLINE_SURFACE ( (
 ( 1.000000000000000000, 0.9510565162951535312, 1.000000000000000000, 0.9510565162951535312, 1.000000000000000000, 0.9510565162951535312, 1.000000000000000000, 0.9510565162951535312, 1.000000000000000000, 0.9510565162951535312, 1.000000000000000000, 0.9510565162951535312, 1.000000000000000000, 0.9510565162951535312, 1.000000000000000000, 0.9510565162951535312, 1.000000000000000000, 0.9510565162951535312, 1.000000000000000000, 0.9510565162951535312, 1.000000000000000000, 0.9510565162951535312, 1.000000000000000000, 0.9510565162951535312, 1.000000000000000000, 0.9510565162951535312, 1.000000000000000000, 0.9510565162951535312, 1.000000000000000000, 0.9510565162951535312, 1.000000000000000000, 0.9510565162951535312, 1.000000000000000000, 0.9510565162951535312, 1.000000000000000000, 0.9510565162951535312, 1.000000000000000000, 0.9510565162951535312, 1.000000000000000000, 0.9510565162951535312, 1.000000000000000000, 0.9510565162951535312, 1.000000000000000000, 0.9510565162951535312, 1.000000000000000000, 0.9510565162951535312, 1.000000000000000000, 0.9510565162951535312, 1.000000000000000000, 0.9510565162951535312, 1.000000000000000000, 0.9510565162951535312, 1.000000000000000000, 0.9510565162951535312, 1.000000000000000000, 0.9510565162951535312, 1.000000000000000000, 0.9510565162951535312, 1.000000000000000000, 0.9510565162951535312, 1.000000000000000000, 0.9510565162951535312, 1.000000000000000000, 0.9510565162951535312, 1.000000000000000000, 0.9510565162951535312, 1.000000000000000000, 0.9510565162951535312, 1.000000000000000000, 0.9510565162951535312, 1.000000000000000000, 0.9510565162951535312, 1.000000000000000000, 0.9510565162951535312, 1.000000000000000000, 0.9510565162951535312, 1.000000000000000000, 0.9510565162951535312, 1.000000000000000000, 0.9510565162951535312, 1.000000000000000000, 0.9510565162951535312, 1.000000000000000000, 0.9510565162951535312, 1.000000000000000000, 0.9510565162951535312, 1.000000000000000000, 0.9510565162951535312, 1.000000000000000000, 0.9510565162951535312, 1.000000000000000000, 0.9510565162951535312, 1.000000000000000000, 0.9510565162951535312, 1.000000000000000000, 0.9510565162951535312, 1.000000000000000000, 0.9510565162951535312, 1.000000000000000000, 0.9510565162951535312, 1.000000000000000000, 0.9510565162951535312, 1.000000000000000000, 0.9510565162951535312, 1.000000000000000000, 0.9510565162951535312, 1.000000000000000000, 0.9510565162951535312, 1.000000000000000000, 0.9510565162951535312, 1.000000000000000000, 0.9510565162951535312, 1.000000000000000000, 0.9510565162951535312, 1.000000000000000000, 0.9510565162951535312, 1.000000000000000000, 0.9510565162951535312, 1.000000000000000000, 0.9510565162951535312, 1.000000000000000000, 0.9510565162951535312, 1.000000000000000000, 0.9510565162951535312, 1.000000000000000000, 0.9510565162951535312, 1.000000000000000000, 0.9510565162951535312, 1.000000000000000000, 0.9510565162951535312, 1.000000000000000000, 0.9510565162951535312, 1.000000000000000000, 0.9510565162951535312, 1.000000000000000000, 0.9510565162951535312, 1.000000000000000000, 0.9510565162951535312, 1.000000000000000000, 0.9510565162951535312, 1.000000000000000000, 0.9510565162951535312, 1.000000000000000000, 0.9510565162951535312, 1.000000000000000000, 0.9510565162951535312, 1.000000000000000000, 0.9510565162951535312, 1.000000000000000000, 0.9510565162951535312, 1.000000000000000000, 0.9510565162951535312, 1.000000000000000000, 0.9510565162951535312, 1.000000000000000000, 0.9510565162951535312, 1.000000000000000000, 0.9510565162951535312, 1.000000000000000000, 0.9510565162951535312, 1.000000000000000000, 0.9510565162951535312, 1.000000000000000000, 0.9510565162951535312, 1.000000000000000000, 0.9510565162951535312, 1.000000000000000000, 0.9510565162951535312, 1.000000000000000000, 0.9510565162951535312, 1.000000000000000000, 0.9510565162951535312, 1.000000000000000000, 0.9510565162951535312, 1.000000000000000000, 0.9510565162951535312, 1.000000000000000000, 0.9510565162951535312, 1.000000000000000000, 0.9510565162951535312, 1.000000000000000000, 0.9510565162951535312, 1.000000000000000000, 0.9510565162951535312, 1.000000000000000000, 0.9510565162951535312, 1.000000000000000000, 0.9510565162951535312, 1.000000000000000000, 0.9510565162951535312, 1.000000000000000000, 0.9510565162951535312, 1.000000000000000000, 0.9510565162951535312, 1.000000000000000000, 0.9510565162951535312, 1.000000000000000000, 0.9510565162951535312, 1.000000000000000000, 0.9510565162951535312, 1.000000000000000000, 0.9510565162951535312, 1.000000000000000000, 0.9510565162951535312, 1.000000000000000000, 0.9510565162951535312, 1.000000000000000000, 0.9510565162951535312, 1.000000000000000000, 0.9510565162951535312, 1.000000000000000000, 0.9510565162951535312, 1.000000000000000000, 0.9510565162951535312, 1.000000000000000000, 0.9510565162951535312, 1.000000000000000000, 0.9510565162951535312, 1.000000000000000000, 0.9510565162951535312, 1.000000000000000000, 0.9510565162951535312, 1.000000000000000000, 0.9510565162951535312, 1.000000000000000000, 0.9510565162951535312, 1.000000000000000000, 0.9510565162951535312, 1.000000000000000000, 0.9510565162951535312, 1.000000000000000000, 0.9510565162951535312, 1.000000000000000000, 0.9510565162951535312, 1.000000000000000000, 0.9510565162951535312, 1.000000000000000000, 0.9510565162951535312, 1.000000000000000000, 0.9510565162951535312, 1.000000000000000000, 0.9510565162951535312, 1.000000000000000000, 0.9510565162951535312, 1.000000000000000000, 0.9510565162951535312, 1.000000000000000000, 0.9510565162951535312, 1.000000000000000000, 0.9510565162951535312, 1.000000000000000000, 0.9510565162951535312, 1.000000000000000000, 0.9510565162951535312, 1.000000000000000000, 0.9510565162951535312, 1.000000000000000000, 0.9510565162951535312, 1.000000000000000000, 0.9510565162951535312, 1.000000000000000000),
 ( 0.3333333333333333703, 0.3170188387650512141, 0.3333333333333333703, 0.3170188387650512141, 0.3333333333333333703, 0.3170188387650512141, 0.3333333333333333703, 0.3170188387650512141, 0.3333333333333333703, 0.3170188387650512141, 0.3333333333333333703, 0.3170188387650512141, 0.3333333333333333703, 0.3170188387650512141, 0.3333333333333333703, 0.3170188387650512141, 0.3333333333333333703, 0.3170188387650512141, 0.3333333333333333703, 0.3170188387650512141, 0.3333333333333333703, 0.3170188387650512141, 0.3333333333333333703, 0.3170188387650512141, 0.3333333333333333703, 0.3170188387650512141, 0.3333333333333333703, 0.3170188387650512141, 0.3333333333333333703, 0.3170188387650512141, 0.3333333333333333703, 0.3170188387650512141, 0.3333333333333333703, 0.3170188387650512141, 0.3333333333333333703, 0.3170188387650512141, 0.3333333333333333703, 0.3170188387650512141, 0.3333333333333333703, 0.3170188387650512141, 0.3333333333333333703, 0.3170188387650512141, 0.3333333333333333703, 0.3170188387650512141, 0.3333333333333333703, 0.3170188387650512141, 0.3333333333333333703, 0.3170188387650512141, 0.3333333333333333703, 0.3170188387650512141, 0.3333333333333333703, 0.3170188387650512141, 0.3333333333333333703, 0.3170188387650512141, 0.3333333333333333703, 0.3170188387650512141, 0.3333333333333333703, 0.3170188387650512141, 0.3333333333333333703, 0.3170188387650512141, 0.3333333333333333703, 0.3170188387650512141, 0.3333333333333333703, 0.3170188387650512141, 0.3333333333333333703, 0.3170188387650512141, 0.3333333333333333703, 0.3170188387650512141, 0.3333333333333333703, 0.3170188387650512141, 0.3333333333333333703, 0.3170188387650512141, 0.3333333333333333703, 0.3170188387650512141, 0.3333333333333333703, 0.3170188387650512141, 0.3333333333333333703, 0.3170188387650512141, 0.3333333333333333703, 0.3170188387650512141, 0.3333333333333333703, 0.3170188387650512141, 0.3333333333333333703, 0.3170188387650512141, 0.3333333333333333703, 0.3170188387650512141, 0.3333333333333333703, 0.3170188387650512141, 0.3333333333333333703, 0.3170188387650512141, 0.3333333333333333703, 0.3170188387650512141, 0.3333333333333333703, 0.3170188387650512141, 0.3333333333333333703, 0.3170188387650512141, 0.3333333333333333703, 0.3170188387650512141, 0.3333333333333333703, 0.3170188387650512141, 0.3333333333333333703, 0.3170188387650512141, 0.3333333333333333703, 0.3170188387650512141, 0.3333333333333333703, 0.3170188387650512141, 0.3333333333333333703, 0.3170188387650512141, 0.3333333333333333703, 0.3170188387650512141, 0.3333333333333333703, 0.3170188387650512141, 0.3333333333333333703, 0.3170188387650512141, 0.3333333333333333703, 0.3170188387650512141, 0.3333333333333333703, 0.3170188387650512141, 0.3333333333333333703, 0.3170188387650512141, 0.3333333333333333703, 0.3170188387650512141, 0.3333333333333333703, 0.3170188387650512141, 0.3333333333333333703, 0.3170188387650512141, 0.3333333333333333703, 0.3170188387650512141, 0.3333333333333333703, 0.3170188387650512141, 0.3333333333333333703, 0.3170188387650512141, 0.3333333333333333703, 0.3170188387650512141, 0.3333333333333333703, 0.3170188387650512141, 0.3333333333333333703, 0.3170188387650512141, 0.3333333333333333703, 0.3170188387650512141, 0.3333333333333333703, 0.3170188387650512141, 0.3333333333333333703, 0.3170188387650512141, 0.3333333333333333703, 0.3170188387650512141, 0.3333333333333333703, 0.3170188387650512141, 0.3333333333333333703, 0.3170188387650512141, 0.3333333333333333703, 0.3170188387650512141, 0.3333333333333333703, 0.3170188387650512141, 0.3333333333333333703, 0.3170188387650512141, 0.3333333333333333703, 0.3170188387650512141, 0.3333333333333333703, 0.3170188387650512141, 0.3333333333333333703, 0.3170188387650512141, 0.3333333333333333703, 0.3170188387650512141, 0.3333333333333333703, 0.3170188387650512141, 0.3333333333333333703, 0.3170188387650512141, 0.3333333333333333703, 0.3170188387650512141, 0.3333333333333333703, 0.3170188387650512141, 0.3333333333333333703, 0.3170188387650512141, 0.3333333333333333703, 0.3170188387650512141, 0.3333333333333333703, 0.3170188387650512141, 0.3333333333333333703, 0.3170188387650512141, 0.3333333333333333703, 0.3170188387650512141, 0.3333333333333333703, 0.3170188387650512141, 0.3333333333333333703, 0.3170188387650512141, 0.3333333333333333703, 0.3170188387650512141, 0.3333333333333333703, 0.3170188387650512141, 0.3333333333333333703, 0.3170188387650512141, 0.3333333333333333703, 0.3170188387650512141, 0.3333333333333333703, 0.3170188387650512141, 0.3333333333333333703, 0.3170188387650512141, 0.3333333333333333703, 0.3170188387650512141, 0.3333333333333333703, 0.3170188387650512141, 0.3333333333333333703, 0.3170188387650512141, 0.3333333333333333703, 0.3170188387650512141, 0.3333333333333333703, 0.3170188387650512141, 0.3333333333333333703, 0.3170188387650512141, 0.3333333333333333703, 0.3170188387650512141, 0.3333333333333333703, 0.3170188387650512141, 0.3333333333333333703, 0.3170188387650512141, 0.3333333333333333703, 0.3170188387650512141, 0.3333333333333333703, 0.3170188387650512141, 0.3333333333333333703, 0.3170188387650512141, 0.3333333333333333703, 0.3170188387650512141, 0.3333333333333333703, 0.3170188387650512141, 0.3333333333333333703, 0.3170188387650512141, 0.3333333333333333703, 0.3170188387650512141, 0.3333333333333333703, 0.3170188387650512141, 0.3333333333333333703, 0.3170188387650512141, 0.3333333333333333703, 0.3170188387650512141, 0.3333333333333333703, 0.3170188387650512141, 0.3333333333333333703, 0.3170188387650512141, 0.3333333333333333703, 0.3170188387650512141, 0.3333333333333333703, 0.3170188387650512141, 0.3333333333333333703, 0.3170188387650512141, 0.3333333333333333703, 0.3170188387650512141, 0.3333333333333333703, 0.3170188387650512141, 0.3333333333333333703, 0.3170188387650512141, 0.3333333333333333703, 0.3170188387650512141, 0.3333333333333333703, 0.3170188387650512141, 0.3333333333333333703, 0.3170188387650512141, 0.3333333333333333703, 0.3170188387650512141, 0.3333333333333333703),
 ( 0.3333333333333333703, 0.3170188387650512141, 0.3333333333333333703, 0.3170188387650512141, 0.3333333333333333703, 0.3170188387650512141, 0.3333333333333333703, 0.3170188387650512141, 0.3333333333333333703, 0.3170188387650512141, 0.3333333333333333703, 0.3170188387650512141, 0.3333333333333333703, 0.3170188387650512141, 0.3333333333333333703, 0.3170188387650512141, 0.3333333333333333703, 0.3170188387650512141, 0.3333333333333333703, 0.3170188387650512141, 0.3333333333333333703, 0.3170188387650512141, 0.3333333333333333703, 0.3170188387650512141, 0.3333333333333333703, 0.3170188387650512141, 0.3333333333333333703, 0.3170188387650512141, 0.3333333333333333703, 0.3170188387650512141, 0.3333333333333333703, 0.3170188387650512141, 0.3333333333333333703, 0.3170188387650512141, 0.3333333333333333703, 0.3170188387650512141, 0.3333333333333333703, 0.3170188387650512141, 0.3333333333333333703, 0.3170188387650512141, 0.3333333333333333703, 0.3170188387650512141, 0.3333333333333333703, 0.3170188387650512141, 0.3333333333333333703, 0.3170188387650512141, 0.3333333333333333703, 0.3170188387650512141, 0.3333333333333333703, 0.3170188387650512141, 0.3333333333333333703, 0.3170188387650512141, 0.3333333333333333703, 0.3170188387650512141, 0.3333333333333333703, 0.3170188387650512141, 0.3333333333333333703, 0.3170188387650512141, 0.3333333333333333703, 0.3170188387650512141, 0.3333333333333333703, 0.3170188387650512141, 0.3333333333333333703, 0.3170188387650512141, 0.3333333333333333703, 0.3170188387650512141, 0.3333333333333333703, 0.3170188387650512141, 0.3333333333333333703, 0.3170188387650512141, 0.3333333333333333703, 0.3170188387650512141, 0.3333333333333333703, 0.3170188387650512141, 0.3333333333333333703, 0.3170188387650512141, 0.3333333333333333703, 0.3170188387650512141, 0.3333333333333333703, 0.3170188387650512141, 0.3333333333333333703, 0.3170188387650512141, 0.3333333333333333703, 0.3170188387650512141, 0.3333333333333333703, 0.3170188387650512141, 0.3333333333333333703, 0.3170188387650512141, 0.3333333333333333703, 0.3170188387650512141, 0.3333333333333333703, 0.3170188387650512141, 0.3333333333333333703, 0.3170188387650512141, 0.3333333333333333703, 0.3170188387650512141, 0.3333333333333333703, 0.3170188387650512141, 0.3333333333333333703, 0.3170188387650512141, 0.3333333333333333703, 0.3170188387650512141, 0.3333333333333333703, 0.3170188387650512141, 0.3333333333333333703, 0.3170188387650512141, 0.3333333333333333703, 0.3170188387650512141, 0.3333333333333333703, 0.3170188387650512141, 0.3333333333333333703, 0.3170188387650512141, 0.3333333333333333703, 0.3170188387650512141, 0.3333333333333333703, 0.3170188387650512141, 0.3333333333333333703, 0.3170188387650512141, 0.3333333333333333703, 0.3170188387650512141, 0.3333333333333333703, 0.3170188387650512141, 0.3333333333333333703, 0.3170188387650512141, 0.3333333333333333703, 0.3170188387650512141, 0.3333333333333333703, 0.3170188387650512141, 0.3333333333333333703, 0.3170188387650512141, 0.3333333333333333703, 0.3170188387650512141, 0.3333333333333333703, 0.3170188387650512141, 0.3333333333333333703, 0.3170188387650512141, 0.3333333333333333703, 0.3170188387650512141, 0.3333333333333333703, 0.3170188387650512141, 0.3333333333333333703, 0.3170188387650512141, 0.3333333333333333703, 0.3170188387650512141, 0.3333333333333333703, 0.3170188387650512141, 0.3333333333333333703, 0.3170188387650512141, 0.3333333333333333703, 0.3170188387650512141, 0.3333333333333333703, 0.3170188387650512141, 0.3333333333333333703, 0.3170188387650512141, 0.3333333333333333703, 0.3170188387650512141, 0.3333333333333333703, 0.3170188387650512141, 0.3333333333333333703, 0.3170188387650512141, 0.3333333333333333703, 0.3170188387650512141, 0.3333333333333333703, 0.3170188387650512141, 0.3333333333333333703, 0.3170188387650512141, 0.3333333333333333703, 0.3170188387650512141, 0.3333333333333333703, 0.3170188387650512141, 0.3333333333333333703, 0.3170188387650512141, 0.3333333333333333703, 0.3170188387650512141, 0.3333333333333333703, 0.3170188387650512141, 0.3333333333333333703, 0.3170188387650512141, 0.3333333333333333703, 0.3170188387650512141, 0.3333333333333333703, 0.3170188387650512141, 0.3333333333333333703, 0.3170188387650512141, 0.3333333333333333703, 0.3170188387650512141, 0.3333333333333333703, 0.3170188387650512141, 0.3333333333333333703, 0.3170188387650512141, 0.3333333333333333703, 0.3170188387650512141, 0.3333333333333333703, 0.3170188387650512141, 0.3333333333333333703, 0.3170188387650512141, 0.3333333333333333703, 0.3170188387650512141, 0.3333333333333333703, 0.3170188387650512141, 0.3333333333333333703, 0.3170188387650512141, 0.3333333333333333703, 0.3170188387650512141, 0.3333333333333333703, 0.3170188387650512141, 0.3333333333333333703, 0.3170188387650512141, 0.3333333333333333703, 0.3170188387650512141, 0.3333333333333333703, 0.3170188387650512141, 0.3333333333333333703, 0.3170188387650512141, 0.3333333333333333703, 0.3170188387650512141, 0.3333333333333333703, 0.3170188387650512141, 0.3333333333333333703, 0.3170188387650512141, 0.3333333333333333703, 0.3170188387650512141, 0.3333333333333333703, 0.3170188387650512141, 0.3333333333333333703, 0.3170188387650512141, 0.3333333333333333703, 0.3170188387650512141, 0.3333333333333333703, 0.3170188387650512141, 0.3333333333333333703, 0.3170188387650512141, 0.3333333333333333703, 0.3170188387650512141, 0.3333333333333333703, 0.3170188387650512141, 0.3333333333333333703, 0.3170188387650512141, 0.3333333333333333703, 0.3170188387650512141, 0.3333333333333333703, 0.3170188387650512141, 0.3333333333333333703, 0.3170188387650512141, 0.3333333333333333703, 0.3170188387650512141, 0.3333333333333333703, 0.3170188387650512141, 0.3333333333333333703, 0.3170188387650512141, 0.3333333333333333703, 0.3170188387650512141, 0.3333333333333333703, 0.3170188387650512141, 0.3333333333333333703, 0.3170188387650512141, 0.3333333333333333703, 0.3170188387650512141, 0.3333333333333333703, 0.3170188387650512141, 0.3333333333333333703),
 ( 1.000000000000000000, 0.9510565162951535312, 1.000000000000000000, 0.9510565162951535312, 1.000000000000000000, 0.9510565162951535312, 1.000000000000000000, 0.9510565162951535312, 1.000000000000000000, 0.9510565162951535312, 1.000000000000000000, 0.9510565162951535312, 1.000000000000000000, 0.9510565162951535312, 1.000000000000000000, 0.9510565162951535312, 1.000000000000000000, 0.9510565162951535312, 1.000000000000000000, 0.9510565162951535312, 1.000000000000000000, 0.9510565162951535312, 1.000000000000000000, 0.9510565162951535312, 1.000000000000000000, 0.9510565162951535312, 1.000000000000000000, 0.9510565162951535312, 1.000000000000000000, 0.9510565162951535312, 1.000000000000000000, 0.9510565162951535312, 1.000000000000000000, 0.9510565162951535312, 1.000000000000000000, 0.9510565162951535312, 1.000000000000000000, 0.9510565162951535312, 1.000000000000000000, 0.9510565162951535312, 1.000000000000000000, 0.9510565162951535312, 1.000000000000000000, 0.9510565162951535312, 1.000000000000000000, 0.9510565162951535312, 1.000000000000000000, 0.9510565162951535312, 1.000000000000000000, 0.9510565162951535312, 1.000000000000000000, 0.9510565162951535312, 1.000000000000000000, 0.9510565162951535312, 1.000000000000000000, 0.9510565162951535312, 1.000000000000000000, 0.9510565162951535312, 1.000000000000000000, 0.9510565162951535312, 1.000000000000000000, 0.9510565162951535312, 1.000000000000000000, 0.9510565162951535312, 1.000000000000000000, 0.9510565162951535312, 1.000000000000000000, 0.9510565162951535312, 1.000000000000000000, 0.9510565162951535312, 1.000000000000000000, 0.9510565162951535312, 1.000000000000000000, 0.9510565162951535312, 1.000000000000000000, 0.9510565162951535312, 1.000000000000000000, 0.9510565162951535312, 1.000000000000000000, 0.9510565162951535312, 1.000000000000000000, 0.9510565162951535312, 1.000000000000000000, 0.9510565162951535312, 1.000000000000000000, 0.9510565162951535312, 1.000000000000000000, 0.9510565162951535312, 1.000000000000000000, 0.9510565162951535312, 1.000000000000000000, 0.9510565162951535312, 1.000000000000000000, 0.9510565162951535312, 1.000000000000000000, 0.9510565162951535312, 1.000000000000000000, 0.9510565162951535312, 1.000000000000000000, 0.9510565162951535312, 1.000000000000000000, 0.9510565162951535312, 1.000000000000000000, 0.9510565162951535312, 1.000000000000000000, 0.9510565162951535312, 1.000000000000000000, 0.9510565162951535312, 1.000000000000000000, 0.9510565162951535312, 1.000000000000000000, 0.9510565162951535312, 1.000000000000000000, 0.9510565162951535312, 1.000000000000000000, 0.9510565162951535312, 1.000000000000000000, 0.9510565162951535312, 1.000000000000000000, 0.9510565162951535312, 1.000000000000000000, 0.9510565162951535312, 1.000000000000000000, 0.9510565162951535312, 1.000000000000000000, 0.9510565162951535312, 1.000000000000000000, 0.9510565162951535312, 1.000000000000000000, 0.9510565162951535312, 1.000000000000000000, 0.9510565162951535312, 1.000000000000000000, 0.9510565162951535312, 1.000000000000000000, 0.9510565162951535312, 1.000000000000000000, 0.9510565162951535312, 1.000000000000000000, 0.9510565162951535312, 1.000000000000000000, 0.9510565162951535312, 1.000000000000000000, 0.9510565162951535312, 1.000000000000000000, 0.9510565162951535312, 1.000000000000000000, 0.9510565162951535312, 1.000000000000000000, 0.9510565162951535312, 1.000000000000000000, 0.9510565162951535312, 1.000000000000000000, 0.9510565162951535312, 1.000000000000000000, 0.9510565162951535312, 1.000000000000000000, 0.9510565162951535312, 1.000000000000000000, 0.9510565162951535312, 1.000000000000000000, 0.9510565162951535312, 1.000000000000000000, 0.9510565162951535312, 1.000000000000000000, 0.9510565162951535312, 1.000000000000000000, 0.9510565162951535312, 1.000000000000000000, 0.9510565162951535312, 1.000000000000000000, 0.9510565162951535312, 1.000000000000000000, 0.9510565162951535312, 1.000000000000000000, 0.9510565162951535312, 1.000000000000000000, 0.9510565162951535312, 1.000000000000000000, 0.9510565162951535312, 1.000000000000000000, 0.9510565162951535312, 1.000000000000000000, 0.9510565162951535312, 1.000000000000000000, 0.9510565162951535312, 1.000000000000000000, 0.9510565162951535312, 1.000000000000000000, 0.9510565162951535312, 1.000000000000000000, 0.9510565162951535312, 1.000000000000000000, 0.9510565162951535312, 1.000000000000000000, 0.9510565162951535312, 1.000000000000000000, 0.9510565162951535312, 1.000000000000000000, 0.9510565162951535312, 1.000000000000000000, 0.9510565162951535312, 1.000000000000000000, 0.9510565162951535312, 1.000000000000000000, 0.9510565162951535312, 1.000000000000000000, 0.9510565162951535312, 1.000000000000000000, 0.9510565162951535312, 1.000000000000000000, 0.9510565162951535312, 1.000000000000000000, 0.9510565162951535312, 1.000000000000000000, 0.9510565162951535312, 1.000000000000000000, 0.9510565162951535312, 1.000000000000000000, 0.9510565162951535312, 1.000000000000000000, 0.9510565162951535312, 1.000000000000000000, 0.9510565162951535312, 1.000000000000000000, 0.9510565162951535312, 1.000000000000000000, 0.9510565162951535312, 1.000000000000000000, 0.9510565162951535312, 1.000000000000000000, 0.9510565162951535312, 1.000000000000000000, 0.9510565162951535312, 1.000000000000000000, 0.9510565162951535312, 1.000000000000000000, 0.9510565162951535312, 1.000000000000000000, 0.9510565162951535312, 1.000000000000000000, 0.9510565162951535312, 1.000000000000000000, 0.9510565162951535312, 1.000000000000000000, 0.9510565162951535312, 1.000000000000000000, 0.9510565162951535312, 1.000000000000000000, 0.9510565162951535312, 1.000000000000000000, 0.9510565162951535312, 1.000000000000000000, 0.9510565162951535312, 1.000000000000000000, 0.9510565162951535312, 1.000000000000000000, 0.9510565162951535312, 1.000000000000000000, 0.9510565162951535312, 1.000000000000000000),
 ( 0.3333333333333333703, 0.3170188387650512141, 0.3333333333333333703, 0.3170188387650512141, 0.3333333333333333703, 0.3170188387650512141, 0.3333333333333333703, 0.3170188387650512141, 0.3333333333333333703, 0.3170188387650512141, 0.3333333333333333703, 0.3170188387650512141, 0.3333333333333333703, 0.3170188387650512141, 0.3333333333333333703, 0.3170188387650512141, 0.3333333333333333703, 0.3170188387650512141, 0.3333333333333333703, 0.3170188387650512141, 0.3333333333333333703, 0.3170188387650512141, 0.3333333333333333703, 0.3170188387650512141, 0.3333333333333333703, 0.3170188387650512141, 0.3333333333333333703, 0.3170188387650512141, 0.3333333333333333703, 0.3170188387650512141, 0.3333333333333333703, 0.3170188387650512141, 0.3333333333333333703, 0.3170188387650512141, 0.3333333333333333703, 0.3170188387650512141, 0.3333333333333333703, 0.3170188387650512141, 0.3333333333333333703, 0.3170188387650512141, 0.3333333333333333703, 0.3170188387650512141, 0.3333333333333333703, 0.3170188387650512141, 0.3333333333333333703, 0.3170188387650512141, 0.3333333333333333703, 0.3170188387650512141, 0.3333333333333333703, 0.3170188387650512141, 0.3333333333333333703, 0.3170188387650512141, 0.3333333333333333703, 0.3170188387650512141, 0.3333333333333333703, 0.3170188387650512141, 0.3333333333333333703, 0.3170188387650512141, 0.3333333333333333703, 0.3170188387650512141, 0.3333333333333333703, 0.3170188387650512141, 0.3333333333333333703, 0.3170188387650512141, 0.3333333333333333703, 0.3170188387650512141, 0.3333333333333333703, 0.3170188387650512141, 0.3333333333333333703, 0.3170188387650512141, 0.3333333333333333703, 0.3170188387650512141, 0.3333333333333333703, 0.3170188387650512141, 0.3333333333333333703, 0.3170188387650512141, 0.3333333333333333703, 0.3170188387650512141, 0.3333333333333333703, 0.3170188387650512141, 0.3333333333333333703, 0.3170188387650512141, 0.3333333333333333703, 0.3170188387650512141, 0.3333333333333333703, 0.3170188387650512141, 0.3333333333333333703, 0.3170188387650512141, 0.3333333333333333703, 0.3170188387650512141, 0.3333333333333333703, 0.3170188387650512141, 0.3333333333333333703, 0.3170188387650512141, 0.3333333333333333703, 0.3170188387650512141, 0.3333333333333333703, 0.3170188387650512141, 0.3333333333333333703, 0.3170188387650512141, 0.3333333333333333703, 0.3170188387650512141, 0.3333333333333333703, 0.3170188387650512141, 0.3333333333333333703, 0.3170188387650512141, 0.3333333333333333703, 0.3170188387650512141, 0.3333333333333333703, 0.3170188387650512141, 0.3333333333333333703, 0.3170188387650512141, 0.3333333333333333703, 0.3170188387650512141, 0.3333333333333333703, 0.3170188387650512141, 0.3333333333333333703, 0.3170188387650512141, 0.3333333333333333703, 0.3170188387650512141, 0.3333333333333333703, 0.3170188387650512141, 0.3333333333333333703, 0.3170188387650512141, 0.3333333333333333703, 0.3170188387650512141, 0.3333333333333333703, 0.3170188387650512141, 0.3333333333333333703, 0.3170188387650512141, 0.3333333333333333703, 0.3170188387650512141, 0.3333333333333333703, 0.3170188387650512141, 0.3333333333333333703, 0.3170188387650512141, 0.3333333333333333703, 0.3170188387650512141, 0.3333333333333333703, 0.3170188387650512141, 0.3333333333333333703, 0.3170188387650512141, 0.3333333333333333703, 0.3170188387650512141, 0.3333333333333333703, 0.3170188387650512141, 0.3333333333333333703, 0.3170188387650512141, 0.3333333333333333703, 0.3170188387650512141, 0.3333333333333333703, 0.3170188387650512141, 0.3333333333333333703, 0.3170188387650512141, 0.3333333333333333703, 0.3170188387650512141, 0.3333333333333333703, 0.3170188387650512141, 0.3333333333333333703, 0.3170188387650512141, 0.3333333333333333703, 0.3170188387650512141, 0.3333333333333333703, 0.3170188387650512141, 0.3333333333333333703, 0.3170188387650512141, 0.3333333333333333703, 0.3170188387650512141, 0.3333333333333333703, 0.3170188387650512141, 0.3333333333333333703, 0.3170188387650512141, 0.3333333333333333703, 0.3170188387650512141, 0.3333333333333333703, 0.3170188387650512141, 0.3333333333333333703, 0.3170188387650512141, 0.3333333333333333703, 0.3170188387650512141, 0.3333333333333333703, 0.3170188387650512141, 0.3333333333333333703, 0.3170188387650512141, 0.3333333333333333703, 0.3170188387650512141, 0.3333333333333333703, 0.3170188387650512141, 0.3333333333333333703, 0.3170188387650512141, 0.3333333333333333703, 0.3170188387650512141, 0.3333333333333333703, 0.3170188387650512141, 0.3333333333333333703, 0.3170188387650512141, 0.3333333333333333703, 0.3170188387650512141, 0.3333333333333333703, 0.3170188387650512141, 0.3333333333333333703, 0.3170188387650512141, 0.3333333333333333703, 0.3170188387650512141, 0.3333333333333333703, 0.3170188387650512141, 0.3333333333333333703, 0.3170188387650512141, 0.3333333333333333703, 0.3170188387650512141, 0.3333333333333333703, 0.3170188387650512141, 0.3333333333333333703, 0.3170188387650512141, 0.3333333333333333703, 0.3170188387650512141, 0.3333333333333333703, 0.3170188387650512141, 0.3333333333333333703, 0.3170188387650512141, 0.3333333333333333703, 0.3170188387650512141, 0.3333333333333333703, 0.3170188387650512141, 0.3333333333333333703, 0.3170188387650512141, 0.3333333333333333703, 0.3170188387650512141, 0.3333333333333333703, 0.3170188387650512141, 0.3333333333333333703, 0.3170188387650512141, 0.3333333333333333703, 0.3170188387650512141, 0.3333333333333333703, 0.3170188387650512141, 0.3333333333333333703, 0.3170188387650512141, 0.3333333333333333703, 0.3170188387650512141, 0.3333333333333333703, 0.3170188387650512141, 0.3333333333333333703, 0.3170188387650512141, 0.3333333333333333703, 0.3170188387650512141, 0.3333333333333333703, 0.3170188387650512141, 0.3333333333333333703, 0.3170188387650512141, 0.3333333333333333703, 0.3170188387650512141, 0.3333333333333333703, 0.3170188387650512141, 0.3333333333333333703, 0.3170188387650512141, 0.3333333333333333703, 0.3170188387650512141, 0.3333333333333333703, 0.3170188387650512141, 0.3333333333333333703),
 ( 0.3333333333333333703, 0.3170188387650512141, 0.3333333333333333703, 0.3170188387650512141, 0.3333333333333333703, 0.3170188387650512141, 0.3333333333333333703, 0.3170188387650512141, 0.3333333333333333703, 0.3170188387650512141, 0.3333333333333333703, 0.3170188387650512141, 0.3333333333333333703, 0.3170188387650512141, 0.3333333333333333703, 0.3170188387650512141, 0.3333333333333333703, 0.3170188387650512141, 0.3333333333333333703, 0.3170188387650512141, 0.3333333333333333703, 0.3170188387650512141, 0.3333333333333333703, 0.3170188387650512141, 0.3333333333333333703, 0.3170188387650512141, 0.3333333333333333703, 0.3170188387650512141, 0.3333333333333333703, 0.3170188387650512141, 0.3333333333333333703, 0.3170188387650512141, 0.3333333333333333703, 0.3170188387650512141, 0.3333333333333333703, 0.3170188387650512141, 0.3333333333333333703, 0.3170188387650512141, 0.3333333333333333703, 0.3170188387650512141, 0.3333333333333333703, 0.3170188387650512141, 0.3333333333333333703, 0.3170188387650512141, 0.3333333333333333703, 0.3170188387650512141, 0.3333333333333333703, 0.3170188387650512141, 0.3333333333333333703, 0.3170188387650512141, 0.3333333333333333703, 0.3170188387650512141, 0.3333333333333333703, 0.3170188387650512141, 0.3333333333333333703, 0.3170188387650512141, 0.3333333333333333703, 0.3170188387650512141, 0.3333333333333333703, 0.3170188387650512141, 0.3333333333333333703, 0.3170188387650512141, 0.3333333333333333703, 0.3170188387650512141, 0.3333333333333333703, 0.3170188387650512141, 0.3333333333333333703, 0.3170188387650512141, 0.3333333333333333703, 0.3170188387650512141, 0.3333333333333333703, 0.3170188387650512141, 0.3333333333333333703, 0.3170188387650512141, 0.3333333333333333703, 0.3170188387650512141, 0.3333333333333333703, 0.3170188387650512141, 0.3333333333333333703, 0.3170188387650512141, 0.3333333333333333703, 0.3170188387650512141, 0.3333333333333333703, 0.3170188387650512141, 0.3333333333333333703, 0.3170188387650512141, 0.3333333333333333703, 0.3170188387650512141, 0.3333333333333333703, 0.3170188387650512141, 0.3333333333333333703, 0.3170188387650512141, 0.3333333333333333703, 0.3170188387650512141, 0.3333333333333333703, 0.3170188387650512141, 0.3333333333333333703, 0.3170188387650512141, 0.3333333333333333703, 0.3170188387650512141, 0.3333333333333333703, 0.3170188387650512141, 0.3333333333333333703, 0.3170188387650512141, 0.3333333333333333703, 0.3170188387650512141, 0.3333333333333333703, 0.3170188387650512141, 0.3333333333333333703, 0.3170188387650512141, 0.3333333333333333703, 0.3170188387650512141, 0.3333333333333333703, 0.3170188387650512141, 0.3333333333333333703, 0.3170188387650512141, 0.3333333333333333703, 0.3170188387650512141, 0.3333333333333333703, 0.3170188387650512141, 0.3333333333333333703, 0.3170188387650512141, 0.3333333333333333703, 0.3170188387650512141, 0.3333333333333333703, 0.3170188387650512141, 0.3333333333333333703, 0.3170188387650512141, 0.3333333333333333703, 0.3170188387650512141, 0.3333333333333333703, 0.3170188387650512141, 0.3333333333333333703, 0.3170188387650512141, 0.3333333333333333703, 0.3170188387650512141, 0.3333333333333333703, 0.3170188387650512141, 0.3333333333333333703, 0.3170188387650512141, 0.3333333333333333703, 0.3170188387650512141, 0.3333333333333333703, 0.3170188387650512141, 0.3333333333333333703, 0.3170188387650512141, 0.3333333333333333703, 0.3170188387650512141, 0.3333333333333333703, 0.3170188387650512141, 0.3333333333333333703, 0.3170188387650512141, 0.3333333333333333703, 0.3170188387650512141, 0.3333333333333333703, 0.3170188387650512141, 0.3333333333333333703, 0.3170188387650512141, 0.3333333333333333703, 0.3170188387650512141, 0.3333333333333333703, 0.3170188387650512141, 0.3333333333333333703, 0.3170188387650512141, 0.3333333333333333703, 0.3170188387650512141, 0.3333333333333333703, 0.3170188387650512141, 0.3333333333333333703, 0.3170188387650512141, 0.3333333333333333703, 0.3170188387650512141, 0.3333333333333333703, 0.3170188387650512141, 0.3333333333333333703, 0.3170188387650512141, 0.3333333333333333703, 0.3170188387650512141, 0.3333333333333333703, 0.3170188387650512141, 0.3333333333333333703, 0.3170188387650512141, 0.3333333333333333703, 0.3170188387650512141, 0.3333333333333333703, 0.3170188387650512141, 0.3333333333333333703, 0.3170188387650512141, 0.3333333333333333703, 0.3170188387650512141, 0.3333333333333333703, 0.3170188387650512141, 0.3333333333333333703, 0.3170188387650512141, 0.3333333333333333703, 0.3170188387650512141, 0.3333333333333333703, 0.3170188387650512141, 0.3333333333333333703, 0.3170188387650512141, 0.3333333333333333703, 0.3170188387650512141, 0.3333333333333333703, 0.3170188387650512141, 0.3333333333333333703, 0.3170188387650512141, 0.3333333333333333703, 0.3170188387650512141, 0.3333333333333333703, 0.3170188387650512141, 0.3333333333333333703, 0.3170188387650512141, 0.3333333333333333703, 0.3170188387650512141, 0.3333333333333333703, 0.3170188387650512141, 0.3333333333333333703, 0.3170188387650512141, 0.3333333333333333703, 0.3170188387650512141, 0.3333333333333333703, 0.3170188387650512141, 0.3333333333333333703, 0.3170188387650512141, 0.3333333333333333703, 0.3170188387650512141, 0.3333333333333333703, 0.3170188387650512141, 0.3333333333333333703, 0.3170188387650512141, 0.3333333333333333703, 0.3170188387650512141, 0.3333333333333333703, 0.3170188387650512141, 0.3333333333333333703, 0.3170188387650512141, 0.3333333333333333703, 0.3170188387650512141, 0.3333333333333333703, 0.3170188387650512141, 0.3333333333333333703, 0.3170188387650512141, 0.3333333333333333703, 0.3170188387650512141, 0.3333333333333333703, 0.3170188387650512141, 0.3333333333333333703, 0.3170188387650512141, 0.3333333333333333703, 0.3170188387650512141, 0.3333333333333333703, 0.3170188387650512141, 0.3333333333333333703, 0.3170188387650512141, 0.3333333333333333703, 0.3170188387650512141, 0.3333333333333333703, 0.3170188387650512141, 0.3333333333333333703, 0.3170188387650512141, 0.3333333333333333703),
 ( 1.000000000000000000, 0.9510565162951535312, 1.000000000000000000, 0.9510565162951535312, 1.000000000000000000, 0.9510565162951535312, 1.000000000000000000, 0.9510565162951535312, 1.000000000000000000, 0.9510565162951535312, 1.000000000000000000, 0.9510565162951535312, 1.000000000000000000, 0.9510565162951535312, 1.000000000000000000, 0.9510565162951535312, 1.000000000000000000, 0.9510565162951535312, 1.000000000000000000, 0.9510565162951535312, 1.000000000000000000, 0.9510565162951535312, 1.000000000000000000, 0.9510565162951535312, 1.000000000000000000, 0.9510565162951535312, 1.000000000000000000, 0.9510565162951535312, 1.000000000000000000, 0.9510565162951535312, 1.000000000000000000, 0.9510565162951535312, 1.000000000000000000, 0.9510565162951535312, 1.000000000000000000, 0.9510565162951535312, 1.000000000000000000, 0.9510565162951535312, 1.000000000000000000, 0.9510565162951535312, 1.000000000000000000, 0.9510565162951535312, 1.000000000000000000, 0.9510565162951535312, 1.000000000000000000, 0.9510565162951535312, 1.000000000000000000, 0.9510565162951535312, 1.000000000000000000, 0.9510565162951535312, 1.000000000000000000, 0.9510565162951535312, 1.000000000000000000, 0.9510565162951535312, 1.000000000000000000, 0.9510565162951535312, 1.000000000000000000, 0.9510565162951535312, 1.000000000000000000, 0.9510565162951535312, 1.000000000000000000, 0.9510565162951535312, 1.000000000000000000, 0.9510565162951535312, 1.000000000000000000, 0.9510565162951535312, 1.000000000000000000, 0.9510565162951535312, 1.000000000000000000, 0.9510565162951535312, 1.000000000000000000, 0.9510565162951535312, 1.000000000000000000, 0.9510565162951535312, 1.000000000000000000, 0.9510565162951535312, 1.000000000000000000, 0.9510565162951535312, 1.000000000000000000, 0.9510565162951535312, 1.000000000000000000, 0.9510565162951535312, 1.000000000000000000, 0.9510565162951535312, 1.000000000000000000, 0.9510565162951535312, 1.000000000000000000, 0.9510565162951535312, 1.000000000000000000, 0.9510565162951535312, 1.000000000000000000, 0.9510565162951535312, 1.000000000000000000, 0.9510565162951535312, 1.000000000000000000, 0.9510565162951535312, 1.000000000000000000, 0.9510565162951535312, 1.000000000000000000, 0.9510565162951535312, 1.000000000000000000, 0.9510565162951535312, 1.000000000000000000, 0.9510565162951535312, 1.000000000000000000, 0.9510565162951535312, 1.000000000000000000, 0.9510565162951535312, 1.000000000000000000, 0.9510565162951535312, 1.000000000000000000, 0.9510565162951535312, 1.000000000000000000, 0.9510565162951535312, 1.000000000000000000, 0.9510565162951535312, 1.000000000000000000, 0.9510565162951535312, 1.000000000000000000, 0.9510565162951535312, 1.000000000000000000, 0.9510565162951535312, 1.000000000000000000, 0.9510565162951535312, 1.000000000000000000, 0.9510565162951535312, 1.000000000000000000, 0.9510565162951535312, 1.000000000000000000, 0.9510565162951535312, 1.000000000000000000, 0.9510565162951535312, 1.000000000000000000, 0.9510565162951535312, 1.000000000000000000, 0.9510565162951535312, 1.000000000000000000, 0.9510565162951535312, 1.000000000000000000, 0.9510565162951535312, 1.000000000000000000, 0.9510565162951535312, 1.000000000000000000, 0.9510565162951535312, 1.000000000000000000, 0.9510565162951535312, 1.000000000000000000, 0.9510565162951535312, 1.000000000000000000, 0.9510565162951535312, 1.000000000000000000, 0.9510565162951535312, 1.000000000000000000, 0.9510565162951535312, 1.000000000000000000, 0.9510565162951535312, 1.000000000000000000, 0.9510565162951535312, 1.000000000000000000, 0.9510565162951535312, 1.000000000000000000, 0.9510565162951535312, 1.000000000000000000, 0.9510565162951535312, 1.000000000000000000, 0.9510565162951535312, 1.000000000000000000, 0.9510565162951535312, 1.000000000000000000, 0.9510565162951535312, 1.000000000000000000, 0.9510565162951535312, 1.000000000000000000, 0.9510565162951535312, 1.000000000000000000, 0.9510565162951535312, 1.000000000000000000, 0.9510565162951535312, 1.000000000000000000, 0.9510565162951535312, 1.000000000000000000, 0.9510565162951535312, 1.000000000000000000, 0.9510565162951535312, 1.000000000000000000, 0.9510565162951535312, 1.000000000000000000, 0.9510565162951535312, 1.000000000000000000, 0.9510565162951535312, 1.000000000000000000, 0.9510565162951535312, 1.000000000000000000, 0.9510565162951535312, 1.000000000000000000, 0.9510565162951535312, 1.000000000000000000, 0.9510565162951535312, 1.000000000000000000, 0.9510565162951535312, 1.000000000000000000, 0.9510565162951535312, 1.000000000000000000, 0.9510565162951535312, 1.000000000000000000, 0.9510565162951535312, 1.000000000000000000, 0.9510565162951535312, 1.000000000000000000, 0.9510565162951535312, 1.000000000000000000, 0.9510565162951535312, 1.000000000000000000, 0.9510565162951535312, 1.000000000000000000, 0.9510565162951535312, 1.000000000000000000, 0.9510565162951535312, 1.000000000000000000, 0.9510565162951535312, 1.000000000000000000, 0.9510565162951535312, 1.000000000000000000, 0.9510565162951535312, 1.000000000000000000, 0.9510565162951535312, 1.000000000000000000, 0.9510565162951535312, 1.000000000000000000, 0.9510565162951535312, 1.000000000000000000, 0.9510565162951535312, 1.000000000000000000, 0.9510565162951535312, 1.000000000000000000, 0.9510565162951535312, 1.000000000000000000, 0.9510565162951535312, 1.000000000000000000, 0.9510565162951535312, 1.000000000000000000, 0.9510565162951535312, 1.000000000000000000, 0.9510565162951535312, 1.000000000000000000, 0.9510565162951535312, 1.000000000000000000, 0.9510565162951535312, 1.000000000000000000, 0.9510565162951535312, 1.000000000000000000, 0.9510565162951535312, 1.000000000000000000, 0.9510565162951535312, 1.000000000000000000, 0.9510565162951535312, 1.000000000000000000, 0.9510565162951535312, 1.000000000000000000, 0.9510565162951535312, 1.000000000000000000) ) ) 
 REPRESENTATION_ITEM ( '' )  SURFACE ( )  );
#4780=CARTESIAN_POINT ( 'NONE',  ( -4.784657899331159037, -68.89547149457074227, 1.454677039711874675 ) ) ;
#4782=CARTESIAN_POINT ( 'NONE',  ( 1.719659006605287477, -94.84547149457074511, -4.969112962950050338 ) ) ;
#4783=CARTESIAN_POINT ( 'NONE',  ( 4.191402346623195996, -58.80452850542926058, 5.607243785695311900 ) ) ;
#4789=CARTESIAN_POINT ( 'NONE',  ( -0.09506052544083921918, -84.00452850542926342, -4.999999999999997335 ) ) ;
#4790=CARTESIAN_POINT ( 'NONE',  ( 1.529537955723689890, -74.85452850542925773, -5.030887037049978971 ) ) ;
#4792=CARTESIAN_POINT ( 'NONE',  ( 2.862020680886513180, -68.70452850542925205, -4.100960146804039752 ) ) ;
#4793=CARTESIAN_POINT ( 'NONE',  ( -2.823794231030039903, -77.59547149457073090, -1.017458915287723364 ) ) ;
#4794=CARTESIAN_POINT ( 'NONE',  ( 2.493201789345307784, -60.94547149457074653, 1.934965279058241006 ) ) ;
#4795=CARTESIAN_POINT ( 'NONE',  ( -0.09506052544084034328, -75.00452850542924921, -4.999999999999997335 ) ) ;
#4796=CARTESIAN_POINT ( 'NONE',  ( 4.191402346623198660, -91.80452850542926058, 5.607243785695311900 ) ) ;
#4797=CARTESIAN_POINT ( 'NONE',  ( -0.8796985632579406023, -95.14547149457074227, -3.030887037049952326 ) ) ;
#4802=CARTESIAN_POINT ( 'NONE',  ( -0.09506052544081858291, -81.00452850542926342, -2.999999999999997780 ) ) ;
#4803=CARTESIAN_POINT ( 'NONE',  ( -2.369498399071204631, -93.15452850542925489, -6.969112962950009482 ) ) ;
#4804=CARTESIAN_POINT ( 'NONE',  ( 2.179377348189629693, -78.64547149457074227, 7.030887037049939003 ) ) ;
#4806=CARTESIAN_POINT ( 'NONE',  ( 4.784657899331179465, -94.39547149457074227, -1.454677039711874009 ) ) ;
#4807=CARTESIAN_POINT ( 'NONE',  ( 3.154386672714809770, -86.25452850542924921, -0.09995255151727241993 ) ) ;
#4813=CARTESIAN_POINT ( 'NONE',  ( -4.312004677471058756, -69.45452850542925205, -3.009306630940844052 ) ) ;
#4814=CARTESIAN_POINT ( 'NONE',  ( 2.369498399071078509, -82.84547149457074511, -6.969112962950057444 ) ) ;
#4816=CARTESIAN_POINT ( 'NONE',  ( 4.312004677471010794, -73.54547149457073374, -3.009306630940932425 ) ) ;
#4817=CARTESIAN_POINT ( 'NONE',  ( -4.784657899331159037, -68.89547149457074227, 1.454677039711874675 ) ) ;
#4818=CARTESIAN_POINT ( 'NONE',  ( -1.719659006605374074, -63.15452850542925489, -4.969112962950016588 ) ) ;
#4821=CARTESIAN_POINT ( 'NONE',  ( 4.725907263620372056, -73.09547149457074511, 1.635492904037598283 ) ) ;
#4823=CARTESIAN_POINT ( 'NONE',  ( -6.628020296210623385, -57.90452850542925489, 2.253526892787613978 ) ) ;
#4825=AXIS2_PLACEMENT_3D ( 'NONE', #6438, #27, #2610 ) ;
#4833=CARTESIAN_POINT ( 'NONE',  ( -4.725907263620319654, -90.90452850542926910, 1.635492904037698647 ) ) ;
#4834=CARTESIAN_POINT ( 'NONE',  ( 4.194503406049337357, -74.55452850542923215, -3.171033256558100089 ) ) ;
#4836=CARTESIAN_POINT ( 'NONE',  ( -0.09506052544084073186, -72.00452850542926342, -4.999999999999997335 ) ) ;
#4837=CARTESIAN_POINT ( 'NONE',  ( 0.8796985632579628067, -84.64547149457074227, 3.030887037049952326 ) ) ;
#4838=CARTESIAN_POINT ( 'NONE',  ( -4.194503406049381766, -95.44547149457071100, -3.171033256558012159 ) ) ;
#4839=CARTESIAN_POINT ( 'NONE',  ( 4.312004677471076519, -79.95452850542922363, 3.009306630940844496 ) ) ;
#4841=CARTESIAN_POINT ( 'NONE',  ( 4.037591185471444355, -89.70452850542925205, -5.718994135553947977 ) ) ;
#4842=CARTESIAN_POINT ( 'NONE',  ( -1.686450176301567572, -61.20452850542925916, 2.482926158054133303 ) ) ;
#4849=CARTESIAN_POINT ( 'NONE',  ( -2.823794231030022139, -66.90452850542925489, 1.017458915287783316 ) ) ;
#4851=CARTESIAN_POINT ( 'NONE',  ( 0.09506052544073424759, -76.99547149457075079, -6.999999999999997335 ) ) ;
#4854=STYLED_ITEM ( 'NONE', ( #3552 ), #3582 ) ;
#4855=CARTESIAN_POINT ( 'NONE',  ( -2.823794231030019919, -84.90452850542926910, 1.017458915287783316 ) ) ;
#4860=CARTESIAN_POINT ( 'NONE',  ( 3.015831842038231958, -61.80452850542926058, 3.989209796945429432 ) ) ;
#4861=CARTESIAN_POINT ( 'NONE',  ( 4.037591185471561595, -72.79547149457074795, 5.718994135553860936 ) ) ;
#4865=CARTESIAN_POINT ( 'NONE',  ( -1.529537955723777598, -74.14547149457074227, -5.030887037049945221 ) ) ;
#4866=CARTESIAN_POINT ( 'NONE',  ( 1.529537955723795140, -72.64547149457075648, 5.030887037049945221 ) ) ;
#4867=CARTESIAN_POINT ( 'NONE',  ( 1.529537955723689224, -68.85452850542921510, -5.030887037049978971 ) ) ;
#4870=CARTESIAN_POINT ( 'NONE',  ( 4.194503406049400418, -66.94547149457075363, 3.171033256558012159 ) ) ;
#4872=CARTESIAN_POINT ( 'NONE',  ( 2.862020680886516732, -95.70452850542926626, -4.100960146804039752 ) ) ;
#4878=CARTESIAN_POINT ( 'NONE',  ( -4.725907263620319654, -87.90452850542926910, 1.635492904037698647 ) ) ;
#4879=CARTESIAN_POINT ( 'NONE',  ( 4.312004677471075631, -76.95452850542923784, 3.009306630940844496 ) ) ;
#4880=CARTESIAN_POINT ( 'NONE',  ( 3.015831842038231958, -58.80452850542925347, 3.989209796945429432 ) ) ;
#4881=CARTESIAN_POINT ( 'NONE',  ( 0.8796985632579621406, -78.64547149457074227, 3.030887037049952326 ) ) ;
#4882=CARTESIAN_POINT ( 'NONE',  ( 4.312004677471013459, -97.54547149457070532, -3.009306630940933314 ) ) ;
#4883=CARTESIAN_POINT ( 'NONE',  ( 4.784657899331208775, -71.10452850542925773, 1.454677039711774533 ) ) ;
#4884=CARTESIAN_POINT ( 'NONE',  ( -2.179377348189460051, -88.35452850542924352, 7.030887037049988741 ) ) ;
#4885=CARTESIAN_POINT ( 'NONE',  ( -2.882544866740879730, -57.60452850542926484, -0.8366430509618996147 ) ) ;
#4891=CARTESIAN_POINT ( 'NONE',  ( 1.686450176301584003, -65.70452850542925205, -2.482926158054133303 ) ) ;
#4893=CARTESIAN_POINT ( 'NONE',  ( -4.037591185471544719, -77.29547149457074795, -5.718994135553860936 ) ) ;
#4896=CARTESIAN_POINT ( 'NONE',  ( -4.725907263620351628, -92.59547149457074511, -1.635492904037597617 ) ) ;
#4897=CARTESIAN_POINT ( 'NONE',  ( -3.154386672714787565, -87.75452850542924921, 0.09995255151727280851 ) ) ;
#4903=CARTESIAN_POINT ( 'NONE',  ( 0.8796985632579009673, -92.85452850542924352, -3.030887037049972310 ) ) ;
#4904=CARTESIAN_POINT ( 'NONE',  ( -0.09506052544071416643, -75.49547149457075079, 6.999999999999997335 ) ) ;
#4907=CARTESIAN_POINT ( 'NONE',  ( 1.719659006605285922, -76.84547149457071669, -4.969112962950050338 ) ) ;
#4908=CARTESIAN_POINT ( 'NONE',  ( 0.09506052544075450916, -70.99547149457075079, -4.999999999999997335 ) ) ;
#4910=CARTESIAN_POINT ( 'NONE',  ( 4.784657899331208775, -68.10452850542925773, 1.454677039711774533 ) ) ;
#4912=CARTESIAN_POINT ( 'NONE',  ( -3.015831842038130706, -63.19547149457074653, 3.989209796945492048 ) ) ;
#4914=CARTESIAN_POINT ( 'NONE',  ( 0.09506052544086235345, -94.50452850542926342, 4.999999999999997335 ) ) ;
#4919=CARTESIAN_POINT ( 'NONE',  ( 4.194503406049338246, -83.55452850542921794, -3.171033256558100089 ) ) ;
#4920=CARTESIAN_POINT ( 'NONE',  ( 5.257311121191342806, -91.24547149457072237, 0.09995255151718437925 ) ) ;
#4921=CARTESIAN_POINT ( 'NONE',  ( 4.312004677471074743, -64.95452850542926626, 3.009306630940844052 ) ) ;
#4922=CARTESIAN_POINT ( 'NONE',  ( 3.154386672714809770, -82.24547149457073658, 0.09995255151720662534 ) ) ;
#4923=CARTESIAN_POINT ( 'NONE',  ( 3.015831842038149802, -85.69547149457073942, -3.989209796945492048 ) ) ;
#4924=CARTESIAN_POINT ( 'NONE',  ( -0.09506052544084148126, -66.00452850542926342, -4.999999999999997335 ) ) ;
#4925=CARTESIAN_POINT ( 'NONE',  ( 6.013306294175169597, -82.95452850542925205, 4.245374608440616093 ) ) ;
#4927=CARTESIAN_POINT ( 'NONE',  ( 3.154386672714811102, -94.24547149457075079, 0.09995255151720662534 ) ) ;
#4931=CARTESIAN_POINT ( 'NONE',  ( 4.194503406049340022, -86.55452850542926058, -3.171033256558100977 ) ) ;
#4932=CARTESIAN_POINT ( 'NONE',  ( 3.154386672714808437, -71.25452850542926342, -0.09995255151727241993 ) ) ;
#4933=CARTESIAN_POINT ( 'NONE',  ( -7.360235569667858968, -77.74547149457073658, -0.09995255151716124498 ) ) ;
#4934=CARTESIAN_POINT ( 'NONE',  ( -4.312004677471055203, -93.45452850542922363, -3.009306630940844052 ) ) ;
#4935=CARTESIAN_POINT ( 'NONE',  ( -3.015831842038126709, -96.19547149457075363, 3.989209796945492048 ) ) ;
#4936=CARTESIAN_POINT ( 'NONE',  ( 1.840261337453272583, -88.80452850542926058, 2.371175808195547852 ) ) ;
#4938=ORIENTED_EDGE ( 'NONE', *, *, #1855, .F. ) ;
#4939=CARTESIAN_POINT ( 'NONE',  ( -4.194503406049321370, -58.05452850542925347, 3.171033256558100533 ) ) ;
#4940=CARTESIAN_POINT ( 'NONE',  ( 6.686770931921476979, -67.39547149457074227, -2.072711028461788896 ) ) ;
#4942=CARTESIAN_POINT ( 'NONE',  ( -4.725907263620354293, -71.59547149457074511, -1.635492904037597617 ) ) ;
#4943=CARTESIAN_POINT ( 'NONE',  ( 1.529537955723795140, -69.64547149457074227, 5.030887037049945221 ) ) ;
#4944=CARTESIAN_POINT ( 'NONE',  ( 1.069819614139559061, -94.65452850542924068, 2.969112962950023249 ) ) ;
#4946=CARTESIAN_POINT ( 'NONE',  ( 2.862020680886512736, -65.70452850542925205, -4.100960146804039752 ) ) ;
#4947=CARTESIAN_POINT ( 'NONE',  ( -1.719659006605267937, -60.34547149457073090, 4.969112962950051227 ) ) ;
#4952=CARTESIAN_POINT ( 'NONE',  ( 1.529537955723690557, -80.85452850542925773, -5.030887037049978971 ) ) ;
#4953=CARTESIAN_POINT ( 'NONE',  ( 0.09506052544075639654, -85.99547149457075079, -4.999999999999997335 ) ) ;
#4955=CARTESIAN_POINT ( 'NONE',  ( -4.194503406049320482, -64.05452850542926058, 3.171033256558101865 ) ) ;
#4956=CARTESIAN_POINT ( 'NONE',  ( -3.154386672714789341, -80.74547149457075079, -0.09995255151720625064 ) ) ;
#4957=CARTESIAN_POINT ( 'NONE',  ( 4.037591185471443467, -83.70452850542925205, -5.718994135553947977 ) ) ;
#4958=CARTESIAN_POINT ( 'NONE',  ( -0.09506052544073428923, -84.49547149457075079, 4.999999999999997335 ) ) ;
#4959=CARTESIAN_POINT ( 'NONE',  ( 0.09506052544085895339, -67.50452850542926342, 4.999999999999997335 ) ) ;
#4960=CARTESIAN_POINT ( 'NONE',  ( -4.191402346623178232, -81.30452850542926058, -5.607243785695311900 ) ) ;
#4961=CARTESIAN_POINT ( 'NONE',  ( -1.686450176301615977, -86.29547149457074795, -2.482926158054096000 ) ) ;
#4967=CARTESIAN_POINT ( 'NONE',  ( -5.257311121191322378, -90.75452850542924921, 0.09995255151729529053 ) ) ;
#4968=CARTESIAN_POINT ( 'NONE',  ( -0.8796985632578808723, -64.35452850542924352, 3.030887037049973198 ) ) ;
#4970=CARTESIAN_POINT ( 'NONE',  ( -4.191402346623180897, -60.30452850542926058, -5.607243785695311900 ) ) ;
#4971=CARTESIAN_POINT ( 'NONE',  ( -6.013306294175061240, -72.04547149457074795, 4.245374608440741326 ) ) ;
#4973=CARTESIAN_POINT ( 'NONE',  ( -1.719659006605264384, -87.34547149457074511, 4.969112962950051227 ) ) ;
#4974=CARTESIAN_POINT ( 'NONE',  ( 2.882544866740897049, -83.10452850542927195, 0.8366430509618999478 ) ) ;
#4976=VERTEX_POINT ( 'NONE', #4089 ) ;
#4978=CARTESIAN_POINT ( 'NONE',  ( -4.725907263620323207, -60.90452850542925489, 1.635492904037698647 ) ) ;
#4979=CARTESIAN_POINT ( 'NONE',  ( -6.628020296210667794, -68.59547149457073090, -2.253526892787471869 ) ) ;
#4983=CARTESIAN_POINT ( 'NONE',  ( -3.015831842038129817, -69.19547149457073942, 3.989209796945492048 ) ) ;
#4984=CARTESIAN_POINT ( 'NONE',  ( -1.529537955723777820, -68.14547149457075648, -5.030887037049945221 ) ) ;
#4985=CARTESIAN_POINT ( 'NONE',  ( 4.194503406049334693, -59.55452850542926058, -3.171033256558100089 ) ) ;
#4987=CARTESIAN_POINT ( 'NONE',  ( -3.015831842038215971, -69.30452850542926058, -3.989209796945429432 ) ) ;
#4988=CARTESIAN_POINT ( 'NONE',  ( -1.719659006605267493, -63.34547149457075221, 4.969112962950051227 ) ) ;
#4995=CARTESIAN_POINT ( 'NONE',  ( -2.862020680886494972, -73.20452850542925205, 4.100960146804039752 ) ) ;
#4996=CARTESIAN_POINT ( 'NONE',  ( 1.529537955723797138, -93.64547149457074227, 5.030887037049945221 ) ) ;
#4997=CARTESIAN_POINT ( 'NONE',  ( 2.862020680886511848, -59.70452850542925205, -4.100960146804039752 ) ) ;
#4998=CARTESIAN_POINT ( 'NONE',  ( -0.09506052544075668798, -75.49547149457075079, 2.999999999999997780 ) ) ;
#4999=CARTESIAN_POINT ( 'NONE',  ( 0.09506052544088175460, -79.50452850542926342, 6.999999999999997335 ) ) ;
#5000=CARTESIAN_POINT ( 'NONE',  ( 4.194503406049402194, -90.94547149457071100, 3.171033256558012159 ) ) ;
#5001=CARTESIAN_POINT ( 'NONE',  ( -2.862020680886495860, -64.20452850542926626, 4.100960146804039752 ) ) ;
#5002=CARTESIAN_POINT ( 'NONE',  ( -2.179377348189461827, -76.35452850542924352, 7.030887037049988741 ) ) ;
#5003=CARTESIAN_POINT ( 'NONE',  ( 1.069819614139496000, -91.84547149457074511, -2.969112962950042789 ) ) ;
#5008=CARTESIAN_POINT ( 'NONE',  ( -4.784657899331189235, -87.60452850542925773, -1.454677039711773867 ) ) ;
#5009=CARTESIAN_POINT ( 'NONE',  ( -1.840261337453252821, -66.30452850542926058, -2.371175808195547852 ) ) ;
#5010=CARTESIAN_POINT ( 'NONE',  ( 5.257311121191343695, -95.25452850542924921, -0.09995255151729465215 ) ) ;
#5012=CARTESIAN_POINT ( 'NONE',  ( -6.686770931921459216, -68.89547149457074227, 2.072711028461789784 ) ) ;
#5013=CARTESIAN_POINT ( 'NONE',  ( -4.725907263620351628, -89.59547149457074511, -1.635492904037597617 ) ) ;
#5014=CARTESIAN_POINT ( 'NONE',  ( 2.610703060766983885, -76.95452850542926626, 1.773238653441072232 ) ) ;
#5018=CARTESIAN_POINT ( 'NONE',  ( 1.529537955723688780, -62.85452850542925063, -5.030887037049978971 ) ) ;
#5019=CARTESIAN_POINT ( 'NONE',  ( -6.686770931921459216, -74.89547149457074227, 2.072711028461789784 ) ) ;
#5022=CARTESIAN_POINT ( 'NONE',  ( -1.719659006605267049, -66.34547149457073090, 4.969112962950051227 ) ) ;
#5023=CARTESIAN_POINT ( 'NONE',  ( 5.257311121191341918, -61.24547149457074369, 0.09995255151718437925 ) ) ;
#5024=CARTESIAN_POINT ( 'NONE',  ( -2.610703060766962569, -90.45452850542926626, -1.773238653441072232 ) ) ;
#5029=CARTESIAN_POINT ( 'NONE',  ( -4.784657899331191011, -66.60452850542924352, -1.454677039711773867 ) ) ;
#5030=CARTESIAN_POINT ( 'NONE',  ( -1.529537955723778042, -65.14547149457074227, -5.030887037049945221 ) ) ;
#5037=CARTESIAN_POINT ( 'NONE',  ( -3.015831842038214194, -81.30452850542926058, -3.989209796945429432 ) ) ;
#5038=CARTESIAN_POINT ( 'NONE',  ( -1.529537955723775156, -89.14547149457074227, -5.030887037049945221 ) ) ;
#5040=CARTESIAN_POINT ( 'NONE',  ( -1.719659006605373630, -66.15452850542925489, -4.969112962950015699 ) ) ;
#5041=CARTESIAN_POINT ( 'NONE',  ( 0.8796985632579604752, -66.64547149457072805, 3.030887037049952326 ) ) ;
#5042=CARTESIAN_POINT ( 'NONE',  ( 2.179377348189482699, -83.85452850542927195, -7.030887037049986077 ) ) ;
#5043=CARTESIAN_POINT ( 'NONE',  ( 1.719659006605286367, -85.84547149457075932, -4.969112962950050338 ) ) ;
#5045=CARTESIAN_POINT ( 'NONE',  ( -5.895805022753386027, -79.05452850542926058, 4.407101234057909878 ) ) ;
#5046=CARTESIAN_POINT ( 'NONE',  ( -1.686450176301614867, -92.29547149457074795, -2.482926158054096000 ) ) ;
#5051=CARTESIAN_POINT ( 'NONE',  ( -4.194503406049315153, -94.05452850542926058, 3.171033256558101865 ) ) ;
#5052=CARTESIAN_POINT ( 'NONE',  ( -0.8796985632578817604, -58.35452850542927195, 3.030887037049973198 ) ) ;
#5053=CARTESIAN_POINT ( 'NONE',  ( 4.725907263620341858, -92.40452850542925489, -1.635492904037697981 ) ) ;
#5054=CARTESIAN_POINT ( 'NONE',  ( -6.686770931921459216, -71.89547149457074227, 2.072711028461789784 ) ) ;
#5055=CARTESIAN_POINT ( 'NONE',  ( 1.719659006605287255, -88.84547149457073090, -4.969112962950050338 ) ) ;
#5056=CARTESIAN_POINT ( 'NONE',  ( 2.823794231030040791, -77.40452850542925489, -1.017458915287783316 ) ) ;
#5059=CARTESIAN_POINT ( 'NONE',  ( 3.154386672714809770, -83.25452850542926342, -0.09995255151727241993 ) ) ;
#5060=CARTESIAN_POINT ( 'NONE',  ( -6.013306294175061240, -63.04547149457074084, 4.245374608440741326 ) ) ;
#5062=CARTESIAN_POINT ( 'NONE',  ( 4.312004677471009906, -61.54547149457073374, -3.009306630940932425 ) ) ;
#5063=CARTESIAN_POINT ( 'NONE',  ( -1.529537955723778930, -59.14547149457072805, -5.030887037049945221 ) ) ;
#5064=CARTESIAN_POINT ( 'NONE',  ( 2.610703060766986106, -94.95452850542926626, 1.773238653441072232 ) ) ;
#5067=CARTESIAN_POINT ( 'NONE',  ( 4.194503406049335581, -71.55452850542926058, -3.171033256558100089 ) ) ;
#5068=CARTESIAN_POINT ( 'NONE',  ( 4.037591185471565147, -96.79547149457073374, 5.718994135553860936 ) ) ;
#5076=CARTESIAN_POINT ( 'NONE',  ( 2.862020680886514068, -74.70452850542926626, -4.100960146804039752 ) ) ;
#5077=CARTESIAN_POINT ( 'NONE',  ( 4.725907263620373833, -85.09547149457074511, 1.635492904037598283 ) ) ;
#5078=CARTESIAN_POINT ( 'NONE',  ( 4.371993031763548032, -96.99999999999994316, 1.072437430859429552 ) ) ;
#5079=CARTESIAN_POINT ( 'NONE',  ( 2.610703060766944805, -73.54547149457074795, -1.773238653441125523 ) ) ;
#5080=CARTESIAN_POINT ( 'NONE',  ( -0.09506052544086139588, -75.00452850542926342, -6.999999999999997335 ) ) ;
#5081=CARTESIAN_POINT ( 'NONE',  ( -0.09506052544073352595, -90.49547149457073658, 4.999999999999997335 ) ) ;
#5083=CARTESIAN_POINT ( 'NONE',  ( 6.013306294175169597, -76.95452850542926626, 4.245374608440616093 ) ) ;
#5084=CARTESIAN_POINT ( 'NONE',  ( -2.823794231030038571, -92.59547149457074511, -1.017458915287723364 ) ) ;
#5090=CARTESIAN_POINT ( 'NONE',  ( 5.257311121191343695, -86.25452850542924921, -0.09995255151729466603 ) ) ;
#5091=CARTESIAN_POINT ( 'NONE',  ( -2.823794231030023472, -57.90452850542925489, 1.017458915287783316 ) ) ;
#5092=CARTESIAN_POINT ( 'NONE',  ( -4.784657899331188347, -93.60452850542925773, -1.454677039711773867 ) ) ;
#5093=CARTESIAN_POINT ( 'NONE',  ( -4.191402346623060104, -66.19547149457073942, 5.607243785695398941 ) ) ;
#5095=CARTESIAN_POINT ( 'NONE',  ( -2.862020680886579349, -86.29547149457074795, -4.100960146803977580 ) ) ;
#5096=CARTESIAN_POINT ( 'NONE',  ( 0.8796985632578991909, -77.85452850542925773, -3.030887037049972310 ) ) ;
#5100=CARTESIAN_POINT ( 'NONE',  ( 2.882544866740898382, -89.10452850542925773, 0.8366430509618999478 ) ) ;
#5102=CARTESIAN_POINT ( 'NONE',  ( 6.686770931921525829, -95.10452850542925773, 2.072711028461649008 ) ) ;
#5104=CARTESIAN_POINT ( 'NONE',  ( -0.09506052544073655131, -66.49547149457075079, 4.999999999999997335 ) ) ;
#5105=CARTESIAN_POINT ( 'NONE',  ( 1.529537955723793585, -60.64547149457074937, 5.030887037049945221 ) ) ;
#5106=CARTESIAN_POINT ( 'NONE',  ( 1.069819614139558839, -91.65452850542924068, 2.969112962950023249 ) ) ;
#5108=VECTOR ( 'NONE', #4757, 1000.000000000000000 ) ;
#5109=CARTESIAN_POINT ( 'NONE',  ( -1.719659006605373630, -66.15452850542926910, -4.969112962950016588 ) ) ;
#5111=CARTESIAN_POINT ( 'NONE',  ( -7.360235569667856304, -92.74547149457073658, -0.09995255151716124498 ) ) ;
#5118=CARTESIAN_POINT ( 'NONE',  ( 4.725907263620340082, -77.40452850542925489, -1.635492904037697981 ) ) ;
#5119=CARTESIAN_POINT ( 'NONE',  ( 0.09506052544075525856, -76.99547149457073658, -4.999999999999997335 ) ) ;
#5120=CARTESIAN_POINT ( 'NONE',  ( 2.778853182387016396, -96.99999999999994316, -2.973145269983016092 ) ) ;
#5121=CARTESIAN_POINT ( 'NONE',  ( 2.823794231030058999, -70.09547149457073090, 1.017458915287723809 ) ) ;
#5122=CARTESIAN_POINT ( 'NONE',  ( 5.895805022753406455, -80.55452850542926058, -4.407101234057908989 ) ) ;
#5123=CARTESIAN_POINT ( 'NONE',  ( -4.312004677470992142, -81.04547149457070532, 3.009306630940933758 ) ) ;
#5124=CARTESIAN_POINT ( 'NONE',  ( 4.312004677471073855, -61.95452850542923784, 3.009306630940844496 ) ) ;
#5126=CARTESIAN_POINT ( 'NONE',  ( -6.013306294175152722, -78.45452850542925205, -4.245374608440613429 ) ) ;
#5127=CARTESIAN_POINT ( 'NONE',  ( 1.686450176301637516, -87.79547149457074795, 2.482926158054096000 ) ) ;
#5132=CARTESIAN_POINT ( 'NONE',  ( 5.257311121191341030, -77.25452850542926342, -0.09995255151729466603 ) ) ;
#5133=CARTESIAN_POINT ( 'NONE',  ( 2.610703060766982553, -61.95452850542925916, 1.773238653441072232 ) ) ;
#5134=CARTESIAN_POINT ( 'NONE',  ( -4.725907263620318766, -93.90452850542925489, 1.635492904037698647 ) ) ;
#5135=CARTESIAN_POINT ( 'NONE',  ( 4.037591185471561595, -69.79547149457074795, 5.718994135553860936 ) ) ;
#5136=CARTESIAN_POINT ( 'NONE',  ( -3.015831842038127597, -87.19547149457073942, 3.989209796945492048 ) ) ;
#5137=CARTESIAN_POINT ( 'NONE',  ( -0.8796985632578796510, -73.35452850542924352, 3.030887037049973198 ) ) ;
#5140=CARTESIAN_POINT ( 'NONE',  ( -3.154386672714787565, -87.75452850542924921, 0.09995255151727280851 ) ) ;
#5141=CARTESIAN_POINT ( 'NONE',  ( 7.360235569667875843, -64.24547149457075079, 0.09995255151716216091 ) ) ;
#5145=CARTESIAN_POINT ( 'NONE',  ( -4.194503406049383543, -62.44547149457073232, -3.171033256558012159 ) ) ;
#5146=CARTESIAN_POINT ( 'NONE',  ( -5.257311121191324155, -59.74547149457072948, -0.09995255151718371311 ) ) ;
#5151=CARTESIAN_POINT ( 'NONE',  ( 4.037591185471564259, -87.79547149457074795, 5.718994135553860936 ) ) ;
#5153=CARTESIAN_POINT ( 'NONE',  ( -1.529537955723670128, -79.35452850542925773, 5.030887037049979860 ) ) ;
#5160=CARTESIAN_POINT ( 'NONE',  ( 4.725907263620372945, -79.09547149457074511, 1.635492904037598283 ) ) ;
#5162=CARTESIAN_POINT ( 'NONE',  ( 2.882544866740876177, -67.39547149457074227, -0.8366430509619593447 ) ) ;
#5163=CARTESIAN_POINT ( 'NONE',  ( -5.895805022753386915, -70.05452850542926058, 4.407101234057909878 ) ) ;
#5165=CARTESIAN_POINT ( 'NONE',  ( 2.862020680886599777, -81.79547149457073374, 4.100960146803977580 ) ) ;
#5166=CARTESIAN_POINT ( 'NONE',  ( -1.719659006605374962, -57.15452850542924068, -4.969112962950016588 ) ) ;
#5168=CARTESIAN_POINT ( 'NONE',  ( 5.895805022753404678, -71.55452850542926058, -4.407101234057908989 ) ) ;
#5170=CARTESIAN_POINT ( 'NONE',  ( -0.09506052544075668798, -75.49547149457075079, 2.999999999999997780 ) ) ;
#5173=DIRECTION ( 'NONE',  ( -0.9954714945707483498, -0.09506052544079830746, 1.046913586349167774E-14 ) ) ;
#5174=CARTESIAN_POINT ( 'NONE',  ( 3.015831842038235955, -91.80452850542926058, 3.989209796945429432 ) ) ;
#5176=CARTESIAN_POINT ( 'NONE',  ( 0.09506052544086084077, -82.50452850542926342, 4.999999999999997335 ) ) ;
#5177=CARTESIAN_POINT ( 'NONE',  ( 1.069819614139555064, -61.65452850542925489, 2.969112962950023249 ) ) ;
#5179=CARTESIAN_POINT ( 'NONE',  ( -1.719659006605370744, -87.15452850542926910, -4.969112962950016588 ) ) ;
#5180=CARTESIAN_POINT ( 'NONE',  ( 4.037591185471560706, -60.79547149457074084, 5.718994135553860936 ) ) ;
#5182=CARTESIAN_POINT ( 'NONE',  ( -4.784657899331157260, -80.89547149457074227, 1.454677039711874675 ) ) ;
#5183=CARTESIAN_POINT ( 'NONE',  ( -0.09506052544081895761, -78.00452850542926342, -2.999999999999997780 ) ) ;
#5187=CARTESIAN_POINT ( 'NONE',  ( -0.8796985632578775416, -91.35452850542925773, 3.030887037049973198 ) ) ;
#5188=CARTESIAN_POINT ( 'NONE',  ( -7.360235569667860744, -59.74547149457073658, -0.09995255151716124498 ) ) ;
#5190=CARTESIAN_POINT ( 'NONE',  ( -4.312004677471056979, -81.45452850542923784, -3.009306630940844052 ) ) ;
#5191=CARTESIAN_POINT ( 'NONE',  ( 6.013306294175080779, -97.54547149457074795, -4.245374608440741326 ) ) ;
#5194=CARTESIAN_POINT ( 'NONE',  ( -4.312004677471060532, -63.45452850542926626, -3.009306630940844052 ) ) ;
#5195=CARTESIAN_POINT ( 'NONE',  ( 2.369498399071079842, -94.84547149457073090, -6.969112962950057444 ) ) ;
#5198=CARTESIAN_POINT ( 'NONE',  ( -4.312004677471057867, -72.45452850542922363, -3.009306630940844052 ) ) ;
#5201=CARTESIAN_POINT ( 'NONE',  ( -4.194503406049383543, -83.44547149457071100, -3.171033256558012159 ) ) ;
#5203=CARTESIAN_POINT ( 'NONE',  ( 1.686450176301634185, -63.79547149457074084, 2.482926158054096000 ) ) ;
#5204=CARTESIAN_POINT ( 'NONE',  ( -6.628020296210622497, -69.90452850542925489, 2.253526892787613978 ) ) ;
#5206=CARTESIAN_POINT ( 'NONE',  ( -1.719659006605265050, -78.34547149457074511, 4.969112962950051227 ) ) ;
#5207=CARTESIAN_POINT ( 'NONE',  ( -4.312004677471061420, -57.45452850542925916, -3.009306630940844052 ) ) ;
#5208=CARTESIAN_POINT ( 'NONE',  ( -4.194503406049316041, -85.05452850542926058, 3.171033256558100533 ) ) ;
#5209=CARTESIAN_POINT ( 'NONE',  ( -4.191402346623180009, -69.30452850542926058, -5.607243785695311900 ) ) ;
#5210=CARTESIAN_POINT ( 'NONE',  ( 2.610703060766945693, -76.54547149457074795, -1.773238653441125523 ) ) ;
#5216=CARTESIAN_POINT ( 'NONE',  ( 4.312004677471078296, -88.95452850542922363, 3.009306630940844496 ) ) ;
#5218=CARTESIAN_POINT ( 'NONE',  ( -0.09506052544083921918, -84.00452850542926342, -4.999999999999997335 ) ) ;
#5219=CARTESIAN_POINT ( 'NONE',  ( -2.882544866740856637, -86.89547149457074227, 0.8366430509619596778 ) ) ;
#5221=CARTESIAN_POINT ( 'NONE',  ( -1.529537955723668352, -91.35452850542921510, 5.030887037049979860 ) ) ;
#5222=CARTESIAN_POINT ( 'NONE',  ( 4.191402346623076980, -61.69547149457074653, -5.607243785695398941 ) ) ;
#5223=CARTESIAN_POINT ( 'NONE',  ( 1.069819614139555952, -67.65452850542925489, 2.969112962950023249 ) ) ;
#5226=CARTESIAN_POINT ( 'NONE',  ( -0.8796985632578782077, -85.35452850542924352, 3.030887037049973198 ) ) ;
#5227=CARTESIAN_POINT ( 'NONE',  ( 0.09506052544088365586, -94.50452850542926342, 6.999999999999997335 ) ) ;
#5230=CARTESIAN_POINT ( 'NONE',  ( -5.257311121191324155, -75.75452850542922079, 0.09995255151729526277 ) ) ;
#5231=CARTESIAN_POINT ( 'NONE',  ( -2.179377348189609265, -92.14547149457074227, -7.030887037049939003 ) ) ;
#5234=CARTESIAN_POINT ( 'NONE',  ( -2.493201789345291797, -71.44547149457072521, -1.934965279058240561 ) ) ;
#5236=CARTESIAN_POINT ( 'NONE',  ( -4.725907263620324095, -57.90452850542925489, 1.635492904037698647 ) ) ;
#5237=CARTESIAN_POINT ( 'NONE',  ( -2.179377348189609265, -92.14547149457074227, -7.030887037049939003 ) ) ;
#5239=CARTESIAN_POINT ( 'NONE',  ( -5.257311121191324155, -75.75452850542922079, 0.09995255151729526277 ) ) ;
#5244=CARTESIAN_POINT ( 'NONE',  ( 1.529537955723795584, -78.64547149457074227, 5.030887037049945221 ) ) ;
#5246=CARTESIAN_POINT ( 'NONE',  ( 2.882544866740875733, -64.39547149457074227, -0.8366430509619593447 ) ) ;
#5247=CARTESIAN_POINT ( 'NONE',  ( 2.369498399071224171, -67.65452850542925489, 6.969112962950009482 ) ) ;
#5250=CARTESIAN_POINT ( 'NONE',  ( -0.09506052544073541333, -75.49547149457073658, 4.999999999999997335 ) ) ;
#5252=CARTESIAN_POINT ( 'NONE',  ( -0.09506052544083884448, -87.00452850542924921, -4.999999999999997335 ) ) ;
#5254=CARTESIAN_POINT ( 'NONE',  ( -6.686770931921506289, -69.60452850542924352, -2.072711028461647675 ) ) ;
#5255=CARTESIAN_POINT ( 'NONE',  ( 2.823794231030059887, -76.09547149457073090, 1.017458915287723809 ) ) ;
#5260=CARTESIAN_POINT ( 'NONE',  ( -1.719659006605370744, -90.15452850542922647, -4.969112962950016588 ) ) ;
#5262=CARTESIAN_POINT ( 'NONE',  ( 4.784657899331210551, -80.10452850542925773, 1.454677039711774533 ) ) ;
#5263=CARTESIAN_POINT ( 'NONE',  ( -1.686450176301614867, -92.29547149457074795, -2.482926158054096000 ) ) ;
#5265=CARTESIAN_POINT ( 'NONE',  ( -5.257311121191323267, -84.75452850542923500, 0.09995255151729526277 ) ) ;
#5267=CARTESIAN_POINT ( 'NONE',  ( 0.09506052544088365586, -94.50452850542926342, 6.999999999999997335 ) ) ;
#5268=CARTESIAN_POINT ( 'NONE',  ( -1.069819614139540187, -63.15452850542925489, -2.969112962950023249 ) ) ;
#5271=CARTESIAN_POINT ( 'NONE',  ( 2.823794231030040791, -80.40452850542925489, -1.017458915287783316 ) ) ;
#5272=CARTESIAN_POINT ( 'NONE',  ( -6.013306294175149169, -90.45452850542926626, -4.245374608440613429 ) ) ;
#5274=CARTESIAN_POINT ( 'NONE',  ( 5.895805022753496161, -84.94547149457073942, 4.407101234057782868 ) ) ;
#5277=CARTESIAN_POINT ( 'NONE',  ( 2.493201789345308672, -66.94547149457073942, 1.934965279058241006 ) ) ;
#5278=CARTESIAN_POINT ( 'NONE',  ( -5.257311121191324155, -57.75452850542923500, 0.09995255151729526277 ) ) ;
#5280=CARTESIAN_POINT ( 'NONE',  ( -3.015831842038216859, -63.30452850542925347, -3.989209796945429432 ) ) ;
#5281=CARTESIAN_POINT ( 'NONE',  ( 6.013306294175080779, -85.54547149457074795, -4.245374608440741326 ) ) ;
#5283=CARTESIAN_POINT ( 'NONE',  ( 5.257311121191341918, -77.25452850542926342, -0.09995255151729465215 ) ) ;
#5287=CARTESIAN_POINT ( 'NONE',  ( 4.194503406049402194, -75.94547149457075363, 3.171033256558012159 ) ) ;
#5289=CARTESIAN_POINT ( 'NONE',  ( 2.493201789345307784, -60.94547149457074653, 1.934965279058241006 ) ) ;
#5290=CARTESIAN_POINT ( 'NONE',  ( 4.037591185471441690, -71.70452850542925205, -5.718994135553947977 ) ) ;
#5292=CARTESIAN_POINT ( 'NONE',  ( -1.529537955723776710, -80.14547149457072805, -5.030887037049945221 ) ) ;
#5295=CARTESIAN_POINT ( 'NONE',  ( 5.257311121191342806, -89.25452850542924921, -0.09995255151729465215 ) ) ;
#5296=CARTESIAN_POINT ( 'NONE',  ( -2.369498399071207739, -72.15452850542922647, -6.969112962950009482 ) ) ;
#5297=CARTESIAN_POINT ( 'NONE',  ( -1.686450176301616866, -77.29547149457074795, -2.482926158054096000 ) ) ;
#5302=CARTESIAN_POINT ( 'NONE',  ( -4.784657899331188347, -93.60452850542925773, -1.454677039711773867 ) ) ;
#5303=CARTESIAN_POINT ( 'NONE',  ( -1.529537955723668352, -91.35452850542921510, 5.030887037049979860 ) ) ;
#5305=CARTESIAN_POINT ( 'NONE',  ( 4.725907263620340082, -77.40452850542925489, -1.635492904037697981 ) ) ;
#5306=CARTESIAN_POINT ( 'NONE',  ( -2.610703060766923933, -90.04547149457074795, 1.773238653441125745 ) ) ;
#5308=CARTESIAN_POINT ( 'NONE',  ( -4.725907263620319654, -87.90452850542926910, 1.635492904037698647 ) ) ;
#5309=CARTESIAN_POINT ( 'NONE',  ( 6.013306294175172262, -94.95452850542926626, 4.245374608440616093 ) ) ;
#5310=CARTESIAN_POINT ( 'NONE',  ( 2.493201789345269592, -62.55452850542925347, -1.934965279058294518 ) ) ;
#5313=CARTESIAN_POINT ( 'NONE',  ( -2.823794231030020363, -81.90452850542925489, 1.017458915287783316 ) ) ;
#5314=CARTESIAN_POINT ( 'NONE',  ( -4.191402346623176456, -93.30452850542926058, -5.607243785695311900 ) ) ;
#5317=CARTESIAN_POINT ( 'NONE',  ( -7.360235569667856304, -89.74547149457073658, -0.09995255151716124498 ) ) ;
#5320=CARTESIAN_POINT ( 'NONE',  ( -3.154386672714791118, -65.74547149457073658, -0.09995255151720625064 ) ) ;
#5323=CARTESIAN_POINT ( 'NONE',  ( -4.312004677471057867, -72.45452850542922363, -3.009306630940844052 ) ) ;
#5324=CARTESIAN_POINT ( 'NONE',  ( -2.179377348189610597, -80.14547149457074227, -7.030887037049939003 ) ) ;
#5328=CARTESIAN_POINT ( 'NONE',  ( 4.725907263620340082, -71.40452850542925489, -1.635492904037697981 ) ) ;
#5330=CARTESIAN_POINT ( 'NONE',  ( 3.015831842038148469, -73.69547149457073942, -3.989209796945492048 ) ) ;
#5332=CARTESIAN_POINT ( 'NONE',  ( -2.610703060766927042, -66.04547149457074795, 1.773238653441125745 ) ) ;
#5333=CARTESIAN_POINT ( 'NONE',  ( -6.686770931921506289, -69.60452850542924352, -2.072711028461647675 ) ) ;
#5335=CARTESIAN_POINT ( 'NONE',  ( -4.784657899331190123, -84.60452850542927195, -1.454677039711773867 ) ) ;
#5336=CARTESIAN_POINT ( 'NONE',  ( 5.895805022753404678, -68.55452850542926058, -4.407101234057908989 ) ) ;
#5337=CARTESIAN_POINT ( 'NONE',  ( 2.823794231030060331, -82.09547149457075932, 1.017458915287723809 ) ) ;
#5340=CARTESIAN_POINT ( 'NONE',  ( -4.312004677471055203, -93.45452850542922363, -3.009306630940844052 ) ) ;
#5341=CARTESIAN_POINT ( 'NONE',  ( 4.194503406049338246, -80.55452850542926058, -3.171033256558100089 ) ) ;
#5343=CARTESIAN_POINT ( 'NONE',  ( 0.09506052544085932809, -70.50452850542926342, 4.999999999999997335 ) ) ;
#5344=CARTESIAN_POINT ( 'NONE',  ( -1.069819614139473352, -87.34547149457073090, 2.969112962950044121 ) ) ;
#5345=CARTESIAN_POINT ( 'NONE',  ( -0.09506052544083846978, -90.00452850542924921, -4.999999999999997335 ) ) ;
#5346=CARTESIAN_POINT ( 'NONE',  ( -4.037591185471420374, -94.20452850542928047, 5.718994135553947977 ) ) ;
#5348=CARTESIAN_POINT ( 'NONE',  ( 2.610703060766982553, -61.95452850542925916, 1.773238653441072232 ) ) ;
#5353=CARTESIAN_POINT ( 'NONE',  ( -0.8796985632578793179, -76.35452850542924352, 3.030887037049973198 ) ) ;
#5354=CARTESIAN_POINT ( 'NONE',  ( 6.628020296210642037, -92.40452850542925489, -2.253526892787612645 ) ) ;
#5355=CARTESIAN_POINT ( 'NONE',  ( 5.895805022753496161, -90.94547149457073942, 4.407101234057782868 ) ) ;
#5359=CARTESIAN_POINT ( 'NONE',  ( 2.882544866740876177, -67.39547149457074227, -0.8366430509619593447 ) ) ;
#5363=CARTESIAN_POINT ( 'NONE',  ( 1.719659006605389617, -67.65452850542925489, 4.969112962950016588 ) ) ;
#5364=CARTESIAN_POINT ( 'NONE',  ( 6.013306294175080779, -82.54547149457074795, -4.245374608440741326 ) ) ;
#5366=CARTESIAN_POINT ( 'NONE',  ( -0.09506052544084148126, -66.00452850542926342, -4.999999999999997335 ) ) ;
#5369=PRODUCT_DEFINITION_FORMATION_WITH_SPECIFIED_SOURCE ( 'ANY', '', #8042, .NOT_KNOWN. ) ;
#5370=CARTESIAN_POINT ( 'NONE',  ( 4.725907263620372056, -67.09547149457073090, 1.635492904037598283 ) ) ;
#5372=CARTESIAN_POINT ( 'NONE',  ( -1.840261337453202195, -63.19547149457074653, 2.371175808195584267 ) ) ;
#5373=CARTESIAN_POINT ( 'NONE',  ( -2.179377348189463159, -64.35452850542924352, 7.030887037049988741 ) ) ;
#5377=CARTESIAN_POINT ( 'NONE',  ( -5.257311121191322378, -87.75452850542922079, 0.09995255151729526277 ) ) ;
#5378=CARTESIAN_POINT ( 'NONE',  ( -6.013306294175153610, -63.45452850542924494, -4.245374608440613429 ) ) ;
#5381=CARTESIAN_POINT ( 'NONE',  ( 2.823794231030059443, -73.09547149457071669, 1.017458915287723809 ) ) ;
#5384=CARTESIAN_POINT ( 'NONE',  ( 4.194503406049339134, -92.55452850542924637, -3.171033256558100089 ) ) ;
#5385=CARTESIAN_POINT ( 'NONE',  ( 0.09506052544086007750, -76.50452850542924921, 4.999999999999997335 ) ) ;
#5387=CARTESIAN_POINT ( 'NONE',  ( 4.194503406049336469, -71.55452850542926058, -3.171033256558100977 ) ) ;
#5388=CARTESIAN_POINT ( 'NONE',  ( 2.493201789345311781, -93.94547149457073942, 1.934965279058241006 ) ) ;
#5389=CARTESIAN_POINT ( 'NONE',  ( -2.862020680886578461, -95.29547149457074795, -4.100960146803977580 ) ) ;
#5390=CARTESIAN_POINT ( 'NONE',  ( 3.015831842038233734, -76.80452850542926058, 3.989209796945429432 ) ) ;
#5391=CARTESIAN_POINT ( 'NONE',  ( -4.191402346623177344, -90.30452850542926058, -5.607243785695311900 ) ) ;
#5392=CARTESIAN_POINT ( 'NONE',  ( 2.882544866740895717, -71.10452850542924352, 0.8366430509618999478 ) ) ;
#5396=CARTESIAN_POINT ( 'NONE',  ( -3.154386672714789785, -75.75452850542926342, 0.09995255151727280851 ) ) ;
#5397=CARTESIAN_POINT ( 'NONE',  ( 0.09506052544088250400, -85.50452850542926342, 6.999999999999997335 ) ) ;
#5398=CARTESIAN_POINT ( 'NONE',  ( 6.628020296210689111, -88.09547149457074511, 2.253526892787472757 ) ) ;
#5401=CARTESIAN_POINT ( 'NONE',  ( 2.882544866740875733, -64.39547149457074227, -0.8366430509619593447 ) ) ;
#5404=CARTESIAN_POINT ( 'NONE',  ( -0.09506052544084073186, -72.00452850542926342, -4.999999999999997335 ) ) ;
#5405=CARTESIAN_POINT ( 'NONE',  ( -0.09506052544071341703, -81.49547149457075079, 6.999999999999997335 ) ) ;
#5406=SURFACE_STYLE_FILL_AREA ( #265 ) ;
#5409=CARTESIAN_POINT ( 'NONE',  ( -4.784657899331158148, -77.89547149457074227, 1.454677039711874675 ) ) ;
#5410=CARTESIAN_POINT ( 'NONE',  ( 0.09506052544085895339, -67.50452850542926342, 4.999999999999997335 ) ) ;
#5413=CARTESIAN_POINT ( 'NONE',  ( -4.312004677470994807, -66.04547149457074795, 3.009306630940933758 ) ) ;
#5415=CARTESIAN_POINT ( 'NONE',  ( -4.725907263620350740, -95.59547149457074511, -1.635492904037597617 ) ) ;
#5416=CARTESIAN_POINT ( 'NONE',  ( 7.360235569667875843, -59.25452850542926342, -0.09995255151731691212 ) ) ;
#5420=CARTESIAN_POINT ( 'NONE',  ( 4.194503406049338246, -80.55452850542926058, -3.171033256558100089 ) ) ;
#5423=CARTESIAN_POINT ( 'NONE',  ( -2.862020680886493196, -85.20452850542925205, 4.100960146804039752 ) ) ;
#5424=CARTESIAN_POINT ( 'NONE',  ( -5.257311121191324155, -75.75452850542922079, 0.09995255151729526277 ) ) ;
#5426=CARTESIAN_POINT ( 'NONE',  ( -1.719659006605372964, -72.15452850542924068, -4.969112962950015699 ) ) ;
#5427=CARTESIAN_POINT ( 'NONE',  ( -1.840261337453199531, -84.19547149457073942, 2.371175808195584267 ) ) ;
#5428=CARTESIAN_POINT ( 'NONE',  ( 0.09506052544075790922, -97.99547149457075079, -4.999999999999997335 ) ) ;
#5430=CARTESIAN_POINT ( 'NONE',  ( -4.725907263620321430, -75.90452850542925489, 1.635492904037698647 ) ) ;
#5431=CARTESIAN_POINT ( 'NONE',  ( -7.360235569667858080, -84.75452850542926342, 0.09995255151731782806 ) ) ;
#5434=CARTESIAN_POINT ( 'NONE',  ( 0.8796985632579643610, -96.64547149457075648, 3.030887037049952326 ) ) ;
#5439=CARTESIAN_POINT ( 'NONE',  ( 3.154386672714808437, -74.25452850542924921, -0.09995255151727241993 ) ) ;
#5440=CARTESIAN_POINT ( 'NONE',  ( -6.628020296210620721, -84.90452850542926910, 2.253526892787613978 ) ) ;
#5441=CARTESIAN_POINT ( 'NONE',  ( -7.360235569667858080, -83.74547149457075079, -0.09995255151716124498 ) ) ;
#5445=CARTESIAN_POINT ( 'NONE',  ( -3.154386672714789341, -81.75452850542926342, 0.09995255151727280851 ) ) ;
#5451=CARTESIAN_POINT ( 'NONE',  ( -2.862020680886495860, -64.20452850542926626, 4.100960146804039752 ) ) ;
#5452=CARTESIAN_POINT ( 'NONE',  ( 2.179377348189630137, -81.64547149457074227, 7.030887037049939003 ) ) ;
#5454=CARTESIAN_POINT ( 'NONE',  ( 0.09506052544075488386, -73.99547149457075079, -4.999999999999997335 ) ) ;
#5455=CARTESIAN_POINT ( 'NONE',  ( -4.784657899331159925, -65.89547149457074227, 1.454677039711874675 ) ) ;
#5456=CARTESIAN_POINT ( 'NONE',  ( -4.784657899331191899, -63.60452850542925063, -1.454677039711773867 ) ) ;
#5459=CARTESIAN_POINT ( 'NONE',  ( -1.719659006605266827, -69.34547149457074511, 4.969112962950051227 ) ) ;
#5460=CARTESIAN_POINT ( 'NONE',  ( 6.628020296210639373, -62.40452850542925489, -2.253526892787612645 ) ) ;
#5466=CARTESIAN_POINT ( 'NONE',  ( 1.529537955723691889, -86.85452850542921510, -5.030887037049978971 ) ) ;
#5467=CARTESIAN_POINT ( 'NONE',  ( -4.725907263620320542, -78.90452850542925489, 1.635492904037698647 ) ) ;
#5468=ORIENTED_EDGE ( 'NONE', *, *, #7757, .F. ) ;
#5469=CARTESIAN_POINT ( 'NONE',  ( -1.529537955723671683, -67.35452850542925773, 5.030887037049979860 ) ) ;
#5470=CARTESIAN_POINT ( 'NONE',  ( 2.882544866740877954, -82.39547149457074227, -0.8366430509619593447 ) ) ;
#5471=CARTESIAN_POINT ( 'NONE',  ( -2.823794231030042123, -62.59547149457074511, -1.017458915287723364 ) ) ;
#5472=CARTESIAN_POINT ( 'NONE',  ( 1.719659006605390283, -73.65452850542924068, 4.969112962950016588 ) ) ;
#5473=CARTESIAN_POINT ( 'NONE',  ( -2.369498399071205963, -84.15452850542925489, -6.969112962950009482 ) ) ;
#5474=CARTESIAN_POINT ( 'NONE',  ( 3.154386672714811990, -97.24547149457075079, 0.09995255151720662534 ) ) ;
#5480=CARTESIAN_POINT ( 'NONE',  ( 0.8796985632578979697, -68.85452850542924352, -3.030887037049972310 ) ) ;
#5481=CARTESIAN_POINT ( 'NONE',  ( -6.628020296210667794, -77.59547149457073090, -2.253526892787471869 ) ) ;
#5483=CARTESIAN_POINT ( 'NONE',  ( -4.312004677470991254, -93.04547149457074795, 3.009306630940933314 ) ) ;
#5484=CARTESIAN_POINT ( 'NONE',  ( -2.493201789345251385, -82.05452850542926058, 1.934965279058294518 ) ) ;
#5487=EDGE_LOOP ( 'NONE', ( #5867, #4381 ) ) ;
#5489=CARTESIAN_POINT ( 'NONE',  ( -3.015831842038216859, -60.30452850542926058, -3.989209796945429432 ) ) ;
#5490=CARTESIAN_POINT ( 'NONE',  ( 5.895805022753492608, -66.94547149457073942, 4.407101234057782868 ) ) ;
#5492=CARTESIAN_POINT ( 'NONE',  ( -3.015831842038129817, -72.19547149457073942, 3.989209796945492048 ) ) ;
#5493=CARTESIAN_POINT ( 'NONE',  ( 4.725907263620372056, -70.09547149457074511, 1.635492904037598283 ) ) ;
#5494=CARTESIAN_POINT ( 'NONE',  ( 0.09506052544085819012, -61.50452850542925631, 4.999999999999997335 ) ) ;
#5496=CARTESIAN_POINT ( 'NONE',  ( 5.257311121191341918, -67.24547149457075079, 0.09995255151718437925 ) ) ;
#5497=DIRECTION ( 'NONE',  ( 0.000000000000000000, 0.000000000000000000, 1.000000000000000000 ) ) ;
#5498=CARTESIAN_POINT ( 'NONE',  ( 0.09506052544087949252, -61.50452850542925631, 6.999999999999997335 ) ) ;
#5506=CARTESIAN_POINT ( 'NONE',  ( 1.719659006605392504, -88.65452850542925489, 4.969112962950016588 ) ) ;
#5507=CARTESIAN_POINT ( 'NONE',  ( -2.862020680886494084, -79.20452850542925205, 4.100960146804039752 ) ) ;
#5508=CARTESIAN_POINT ( 'NONE',  ( -3.015831842038216859, -60.30452850542926058, -3.989209796945429432 ) ) ;
#5509=CARTESIAN_POINT ( 'NONE',  ( -2.493201789345290464, -77.44547149457073942, -1.934965279058240561 ) ) ;
#5510=CARTESIAN_POINT ( 'NONE',  ( -1.719659006605263496, -96.34547149457074511, 4.969112962950051227 ) ) ;
#5511=CARTESIAN_POINT ( 'NONE',  ( 4.784657899331208775, -68.10452850542925773, 1.454677039711774533 ) ) ;
#5513=CARTESIAN_POINT ( 'NONE',  ( -5.895805022753386027, -85.05452850542926058, 4.407101234057909878 ) ) ;
#5514=CARTESIAN_POINT ( 'NONE',  ( 0.09506052544077894795, -97.99547149457075079, -2.999999999999997780 ) ) ;
#5521=CARTESIAN_POINT ( 'NONE',  ( 2.493201789345271369, -71.55452850542926058, -1.934965279058294518 ) ) ;
#5523=CARTESIAN_POINT ( 'NONE',  ( -4.191402346623057440, -81.19547149457073942, 5.607243785695398941 ) ) ;
#5524=CARTESIAN_POINT ( 'NONE',  ( -5.257311121191322378, -90.75452850542924921, 0.09995255151729526277 ) ) ;
#5525=CARTESIAN_POINT ( 'NONE',  ( 1.529537955723798248, -96.64547149457072805, 5.030887037049945221 ) ) ;
#5526=CARTESIAN_POINT ( 'NONE',  ( -1.069819614139537967, -81.15452850542924068, -2.969112962950023249 ) ) ;
#5529=CARTESIAN_POINT ( 'NONE',  ( -2.862020680886496304, -61.20452850542925205, 4.100960146804039752 ) ) ;
#5530=CARTESIAN_POINT ( 'NONE',  ( -6.628020296210667794, -74.59547149457071669, -2.253526892787471869 ) ) ;
#5532=CARTESIAN_POINT ( 'NONE',  ( 5.257311121191341030, -73.24547149457073658, 0.09995255151718437925 ) ) ;
#5533=CARTESIAN_POINT ( 'NONE',  ( 0.09506052544075412059, -67.99547149457075079, -4.999999999999997335 ) ) ;
#5534=CARTESIAN_POINT ( 'NONE',  ( 3.015831842038231958, -61.80452850542926058, 3.989209796945429432 ) ) ;
#5536=CARTESIAN_POINT ( 'NONE',  ( 2.862020680886597557, -60.79547149457074084, 4.100960146803977580 ) ) ;
#5539=CARTESIAN_POINT ( 'NONE',  ( 1.719659006605392504, -94.65452850542921226, 4.969112962950016588 ) ) ;
#5545=CARTESIAN_POINT ( 'NONE',  ( -3.015831842038213750, -84.30452850542926058, -3.989209796945429432 ) ) ;
#5546=CARTESIAN_POINT ( 'NONE',  ( -1.529537955723774711, -92.14547149457071384, -5.030887037049945221 ) ) ;
#5547=CARTESIAN_POINT ( 'NONE',  ( -3.015831842038216415, -66.30452850542926058, -3.989209796945429432 ) ) ;
#5549=CARTESIAN_POINT ( 'NONE',  ( -0.09506052544075593858, -81.49547149457075079, 2.999999999999997780 ) ) ;
#5550=CARTESIAN_POINT ( 'NONE',  ( 1.840261337453218626, -61.69547149457074653, -2.371175808195584267 ) ) ;
#5551=CARTESIAN_POINT ( 'NONE',  ( -4.725907263620322318, -66.90452850542925489, 1.635492904037698647 ) ) ;
#5552=CARTESIAN_POINT ( 'NONE',  ( 6.628020296210642037, -83.40452850542925489, -2.253526892787612645 ) ) ;
#5553=CARTESIAN_POINT ( 'NONE',  ( -1.840261337453197976, -96.19547149457075363, 2.371175808195584267 ) ) ;
#5557=CARTESIAN_POINT ( 'NONE',  ( -0.09506052544083884448, -87.00452850542924921, -4.999999999999997335 ) ) ;
#5558=CARTESIAN_POINT ( 'NONE',  ( 2.882544866740894829, -65.10452850542924352, 0.8366430509618999478 ) ) ;
#5560=CARTESIAN_POINT ( 'NONE',  ( 0.09506052544073499699, -82.99547149457075079, -6.999999999999997335 ) ) ;
#5561=CARTESIAN_POINT ( 'NONE',  ( -1.719659006605370744, -93.15452850542925489, -4.969112962950016588 ) ) ;
#5562=CARTESIAN_POINT ( 'NONE',  ( 5.257311121191343695, -91.24547149457072237, 0.09995255151718437925 ) ) ;
#5563=CARTESIAN_POINT ( 'NONE',  ( 0.09506052544084032940, -88.50452850542926342, 2.999999999999997780 ) ) ;
#5567=CARTESIAN_POINT ( 'NONE',  ( -4.312004677471060532, -60.45452850542923784, -3.009306630940844052 ) ) ;
#5568=CARTESIAN_POINT ( 'NONE',  ( 6.628020296210686446, -73.09547149457071669, 2.253526892787472757 ) ) ;
#5570=CARTESIAN_POINT ( 'NONE',  ( 4.784657899331177688, -79.39547149457074227, -1.454677039711874009 ) ) ;
#5571=CARTESIAN_POINT ( 'NONE',  ( 4.194503406049401306, -72.94547149457073942, 3.171033256558012159 ) ) ;
#5573=CARTESIAN_POINT ( 'NONE',  ( -4.784657899331191899, -60.60452850542925773, -1.454677039711773867 ) ) ;
#5576=CARTESIAN_POINT ( 'NONE',  ( -4.725907263620321430, -72.90452850542925489, 1.635492904037698647 ) ) ;
#5578=CARTESIAN_POINT ( 'NONE',  ( -4.312004677470994807, -63.04547149457074084, 3.009306630940933758 ) ) ;
#5583=CARTESIAN_POINT ( 'NONE',  ( -1.529537955723668574, -88.35452850542925773, 5.030887037049979860 ) ) ;
#5584=CARTESIAN_POINT ( 'NONE',  ( -4.725907263620352516, -86.59547149457075932, -1.635492904037597617 ) ) ;
#5585=CARTESIAN_POINT ( 'NONE',  ( -5.257311121191325043, -66.75452850542924921, 0.09995255151729529053 ) ) ;
#5586=CARTESIAN_POINT ( 'NONE',  ( 1.840261337453220625, -79.69547149457075363, -2.371175808195584267 ) ) ;
#5587=CARTESIAN_POINT ( 'NONE',  ( 6.628020296210641149, -77.40452850542925489, -2.253526892787612645 ) ) ;
#5588=CARTESIAN_POINT ( 'NONE',  ( 4.194503406049402194, -84.94547149457073942, 3.171033256558012159 ) ) ;
#5589=CARTESIAN_POINT ( 'NONE',  ( 3.015831842038232402, -64.80452850542926058, 3.989209796945429432 ) ) ;
#5590=CARTESIAN_POINT ( 'NONE',  ( 4.191402346623197772, -76.80452850542926058, 5.607243785695311900 ) ) ;
#5591=CARTESIAN_POINT ( 'NONE',  ( -0.8796985632578817604, -58.35452850542927195, 3.030887037049973198 ) ) ;
#5595=CARTESIAN_POINT ( 'NONE',  ( 0.09506052544086235345, -94.50452850542926342, 4.999999999999997335 ) ) ;
#5596=CARTESIAN_POINT ( 'NONE',  ( -0.8796985632578805392, -67.35452850542924352, 3.030887037049973198 ) ) ;
#5598=CARTESIAN_POINT ( 'NONE',  ( 0.09506052544086235345, -94.50452850542926342, 4.999999999999997335 ) ) ;
#5599=CARTESIAN_POINT ( 'NONE',  ( -6.013306294175060351, -78.04547149457074795, 4.245374608440741326 ) ) ;
#5601=CARTESIAN_POINT ( 'NONE',  ( 5.257311121191343695, -88.24547149457073658, 0.09995255151718437925 ) ) ;
#5602=CARTESIAN_POINT ( 'NONE',  ( 2.493201789345272257, -83.55452850542926058, -1.934965279058294518 ) ) ;
#5606=CARTESIAN_POINT ( 'NONE',  ( -1.686450176301563353, -94.20452850542928047, 2.482926158054133303 ) ) ;
#5607=CARTESIAN_POINT ( 'NONE',  ( 6.686770931921476979, -73.39547149457074227, -2.072711028461788896 ) ) ;
#5610=CARTESIAN_POINT ( 'NONE',  ( 4.315201955286068092, -96.99999999999994316, -4.064365295468459927 ) ) ;
#5611=CARTESIAN_POINT ( 'NONE',  ( 1.719659006605284146, -64.84547149457071669, -4.969112962950050338 ) ) ;
#5612=CARTESIAN_POINT ( 'NONE',  ( -5.257311121191324155, -65.74547149457073658, -0.09995255151718371311 ) ) ;
#5613=CARTESIAN_POINT ( 'NONE',  ( 4.725907263620339194, -59.40452850542926200, -1.635492904037697981 ) ) ;
#5615=CARTESIAN_POINT ( 'NONE',  ( -0.09506052544084148126, -66.00452850542926342, -4.999999999999997335 ) ) ;
#5616=CARTESIAN_POINT ( 'NONE',  ( 2.369498399071080286, -97.84547149457073090, -6.969112962950057444 ) ) ;
#5619=ORIENTED_EDGE ( 'NONE', *, *, #6344, .F. ) ;
#5621=CARTESIAN_POINT ( 'NONE',  ( 1.719659006605390283, -73.65452850542924068, 4.969112962950016588 ) ) ;
#5622=EDGE_CURVE ( 'NONE', #7927, #4976, #2545, .T. ) ;
#5623=CARTESIAN_POINT ( 'NONE',  ( 1.719659006605286811, -88.84547149457070248, -4.969112962950050338 ) ) ;
#5624=CARTESIAN_POINT ( 'NONE',  ( -4.312004677471058756, -60.45452850542924494, -3.009306630940843608 ) ) ;
#5625=CARTESIAN_POINT ( 'NONE',  ( -0.09506052544075706268, -72.49547149457075079, 2.999999999999997780 ) ) ;
#5627=CARTESIAN_POINT ( 'NONE',  ( -5.895805022753386027, -82.05452850542926058, 4.407101234057909878 ) ) ;
#5628=CARTESIAN_POINT ( 'NONE',  ( -4.194503406049382654, -89.44547149457073942, -3.171033256558012159 ) ) ;
#5629=CARTESIAN_POINT ( 'NONE',  ( -4.784657899331191011, -69.60452850542925773, -1.454677039711773867 ) ) ;
#5630=CARTESIAN_POINT ( 'NONE',  ( -6.686770931921506289, -75.60452850542924352, -2.072711028461647675 ) ) ;
#5631=CARTESIAN_POINT ( 'NONE',  ( 2.882544866740878842, -88.39547149457074227, -0.8366430509619593447 ) ) ;
#5635=CARTESIAN_POINT ( 'NONE',  ( 0.09506052544075295485, -58.99547149457073658, -4.999999999999997335 ) ) ;
#5637=CARTESIAN_POINT ( 'NONE',  ( 1.719659006605392504, -91.65452850542925489, 4.969112962950015699 ) ) ;
#5638=CARTESIAN_POINT ( 'NONE',  ( 2.610703060766983441, -70.95452850542925205, 1.773238653441072232 ) ) ;
#5641=CARTESIAN_POINT ( 'NONE',  ( 6.686770931921522276, -59.10452850542926484, 2.072711028461649008 ) ) ;
#5642=CARTESIAN_POINT ( 'NONE',  ( 6.686770931921476979, -73.39547149457074227, -2.072711028461788896 ) ) ;
#5643=CARTESIAN_POINT ( 'NONE',  ( 2.862020680886601109, -90.79547149457074795, 4.100960146803977580 ) ) ;
#5644=CARTESIAN_POINT ( 'NONE',  ( 2.882544866740897049, -77.10452850542924352, 0.8366430509618999478 ) ) ;
#5647=CARTESIAN_POINT ( 'NONE',  ( -0.09506052544084186984, -63.00452850542925631, -4.999999999999997335 ) ) ;
#5648=CARTESIAN_POINT ( 'NONE',  ( -0.09506052544071454113, -72.49547149457075079, 6.999999999999997335 ) ) ;
#5649=CARTESIAN_POINT ( 'NONE',  ( 5.679463638039127460, -97.00000000000000000, -1.065672799591116826 ) ) ;
#5650=CARTESIAN_POINT ( 'NONE',  ( -4.312004677470994807, -63.04547149457073374, 3.009306630940933314 ) ) ;
#5651=CARTESIAN_POINT ( 'NONE',  ( 4.725907263620371168, -64.09547149457073090, 1.635492904037598283 ) ) ;
#5652=CARTESIAN_POINT ( 'NONE',  ( -3.154386672714787565, -90.75452850542924921, 0.09995255151727280851 ) ) ;
#5654=CARTESIAN_POINT ( 'NONE',  ( -2.862020680886495860, -64.20452850542926626, 4.100960146804039752 ) ) ;
#5655=CARTESIAN_POINT ( 'NONE',  ( -6.013306294175056799, -96.04547149457074795, 4.245374608440741326 ) ) ;
#5661=CARTESIAN_POINT ( 'NONE',  ( -4.725907263620321430, -75.90452850542925489, 1.635492904037698647 ) ) ;
#5662=CARTESIAN_POINT ( 'NONE',  ( 5.257311121191342806, -94.24547149457070816, 0.09995255151718437925 ) ) ;
#5663=CARTESIAN_POINT ( 'NONE',  ( 1.719659006605388951, -61.65452850542924779, 4.969112962950015699 ) ) ;
#5664=CARTESIAN_POINT ( 'NONE',  ( 1.840261337453219515, -70.69547149457073942, -2.371175808195584267 ) ) ;
#5665=CARTESIAN_POINT ( 'NONE',  ( -2.179377348189461383, -79.35452850542927195, 7.030887037049988741 ) ) ;
#5666=CARTESIAN_POINT ( 'NONE',  ( -5.257311121191322378, -89.74547149457070816, -0.09995255151718371311 ) ) ;
#5667=CARTESIAN_POINT ( 'NONE',  ( 1.529537955723689224, -68.85452850542921510, -5.030887037049978971 ) ) ;
#5668=CARTESIAN_POINT ( 'NONE',  ( -4.037591185471422150, -82.20452850542925205, 5.718994135553947977 ) ) ;
#5669=CARTESIAN_POINT ( 'NONE',  ( -0.09506052544075556388, -84.49547149457075079, 2.999999999999997780 ) ) ;
#5674=CARTESIAN_POINT ( 'NONE',  ( -4.784657899331188347, -93.60452850542925773, -1.454677039711773867 ) ) ;
#5675=CARTESIAN_POINT ( 'NONE',  ( -1.686450176301567572, -61.20452850542925916, 2.482926158054133303 ) ) ;
#5677=CARTESIAN_POINT ( 'NONE',  ( 4.784657899331212327, -95.10452850542925773, 1.454677039711774533 ) ) ;
#5678=CARTESIAN_POINT ( 'NONE',  ( -6.628020296210667794, -71.59547149457071669, -2.253526892787471869 ) ) ;
#5679=CARTESIAN_POINT ( 'NONE',  ( 4.194503406049403083, -90.94547149457072521, 3.171033256558012159 ) ) ;
#5680=CARTESIAN_POINT ( 'NONE',  ( 3.154386672714809325, -80.25452850542926342, -0.09995255151727241993 ) ) ;
#5684=CARTESIAN_POINT ( 'NONE',  ( -1.686450176301564019, -91.20452850542925205, 2.482926158054133303 ) ) ;
#5685=CARTESIAN_POINT ( 'NONE',  ( -4.191402346623060104, -63.19547149457074653, 5.607243785695398941 ) ) ;
#5687=CARTESIAN_POINT ( 'NONE',  ( 4.194503406049401306, -69.94547149457072521, 3.171033256558012159 ) ) ;
#5688=CARTESIAN_POINT ( 'NONE',  ( -2.179377348189608821, -95.14547149457074227, -7.030887037049939003 ) ) ;
#5689=CARTESIAN_POINT ( 'NONE',  ( -2.823794231030019031, -93.90452850542926910, 1.017458915287783316 ) ) ;
#5693=CARTESIAN_POINT ( 'NONE',  ( 4.194503406049335581, -68.55452850542926058, -3.171033256558100089 ) ) ;
#5694=CARTESIAN_POINT ( 'NONE',  ( -4.037591185471542055, -95.29547149457076216, -5.718994135553860936 ) ) ;
#5702=CARTESIAN_POINT ( 'NONE',  ( 1.529537955723689890, -74.85452850542925773, -5.030887037049978971 ) ) ;
#5703=CARTESIAN_POINT ( 'NONE',  ( 4.784657899331178577, -85.39547149457074227, -1.454677039711874009 ) ) ;
#5705=CARTESIAN_POINT ( 'NONE',  ( 2.493201789345310004, -75.94547149457073942, 1.934965279058241006 ) ) ;
#5706=CARTESIAN_POINT ( 'NONE',  ( -6.628020296210620721, -81.90452850542925489, 2.253526892787613978 ) ) ;
#5708=CARTESIAN_POINT ( 'NONE',  ( 1.529537955723796916, -90.64547149457075648, 5.030887037049945221 ) ) ;
#5710=CARTESIAN_POINT ( 'NONE',  ( -5.895805022753386027, -76.05452850542926058, 4.407101234057909878 ) ) ;
#5711=CARTESIAN_POINT ( 'NONE',  ( 2.610703060766946582, -88.54547149457074795, -1.773238653441125523 ) ) ;
#5718=CARTESIAN_POINT ( 'NONE',  ( -3.015831842038213750, -87.30452850542926058, -3.989209796945429432 ) ) ;
#5719=CARTESIAN_POINT ( 'NONE',  ( 1.686450176301638626, -96.79547149457073374, 2.482926158054096000 ) ) ;
#5720=CARTESIAN_POINT ( 'NONE',  ( 4.037591185471440802, -59.70452850542925916, -5.718994135553947977 ) ) ;
#5721=CARTESIAN_POINT ( 'NONE',  ( -4.037591185471545607, -68.29547149457073374, -5.718994135553860936 ) ) ;
#5722=CARTESIAN_POINT ( 'NONE',  ( 2.862020680886600665, -87.79547149457074795, 4.100960146803977580 ) ) ;
#5723=CARTESIAN_POINT ( 'NONE',  ( -1.840261337453251489, -78.30452850542926058, -2.371175808195547852 ) ) ;
#5726=CARTESIAN_POINT ( 'NONE',  ( -0.09506052544081780575, -87.00452850542926342, -2.999999999999997780 ) ) ;
#5727=CARTESIAN_POINT ( 'NONE',  ( 0.09506052544073198551, -58.99547149457073658, -6.999999999999997335 ) ) ;
#5729=CARTESIAN_POINT ( 'NONE',  ( -2.862020680886581570, -68.29547149457074795, -4.100960146803977580 ) ) ;
#5730=CARTESIAN_POINT ( 'NONE',  ( 0.09506052544073653743, -94.99547149457075079, -6.999999999999997335 ) ) ;
#5731=CARTESIAN_POINT ( 'NONE',  ( 2.882544866740898382, -92.10452850542925773, 0.8366430509618999478 ) ) ;
#5733=CARTESIAN_POINT ( 'NONE',  ( 4.312004677471074743, -67.95452850542922363, 3.009306630940844496 ) ) ;
#5734=CARTESIAN_POINT ( 'NONE',  ( -4.037591185471542943, -92.29547149457074795, -5.718994135553860936 ) ) ;
#5743=CARTESIAN_POINT ( 'NONE',  ( -4.312004677471056979, -81.45452850542923784, -3.009306630940844052 ) ) ;
#5744=CARTESIAN_POINT ( 'NONE',  ( -5.257311121191324155, -77.74547149457070816, -0.09995255151718371311 ) ) ;
#5745=CARTESIAN_POINT ( 'NONE',  ( 3.640901902936454437, -96.99999999999988631, -1.978986728491922920 ) ) ;
#5746=CARTESIAN_POINT ( 'NONE',  ( 0.8796985632579609193, -69.64547149457072805, 3.030887037049952326 ) ) ;
#5747=CARTESIAN_POINT ( 'NONE',  ( -6.628020296210620721, -78.90452850542925489, 2.253526892787613978 ) ) ;
#5748=CARTESIAN_POINT ( 'NONE',  ( 1.719659006605285478, -73.84547149457074511, -4.969112962950050338 ) ) ;
#5750=CARTESIAN_POINT ( 'NONE',  ( 4.312004677471079184, -94.95452850542926626, 3.009306630940844496 ) ) ;
#5751=CARTESIAN_POINT ( 'NONE',  ( 6.686770931921524941, -80.10452850542927195, 2.072711028461649008 ) ) ;
#5752=CARTESIAN_POINT ( 'NONE',  ( 1.069819614139496000, -88.84547149457073090, -2.969112962950042789 ) ) ;
#5754=ORIENTED_EDGE ( 'NONE', *, *, #7828, .F. ) ;
#5758=CARTESIAN_POINT ( 'NONE',  ( -3.015831842038213750, -84.30452850542926058, -3.989209796945429432 ) ) ;
#5759=CARTESIAN_POINT ( 'NONE',  ( -1.840261337453197976, -96.19547149457075363, 2.371175808195584267 ) ) ;
#5760=CARTESIAN_POINT ( 'NONE',  ( 2.369498399071222838, -58.65452850542925489, 6.969112962950009482 ) ) ;
#5761=CARTESIAN_POINT ( 'NONE',  ( 2.369498399071076733, -70.84547149457073090, -6.969112962950057444 ) ) ;
#5764=CARTESIAN_POINT ( 'NONE',  ( -4.725907263620352516, -83.59547149457074511, -1.635492904037597617 ) ) ;
#5765=CARTESIAN_POINT ( 'NONE',  ( 1.840261337453270585, -73.80452850542926058, 2.371175808195547852 ) ) ;
#5770=CARTESIAN_POINT ( 'NONE',  ( -2.493201789345250940, -85.05452850542926058, 1.934965279058294518 ) ) ;
#5771=CARTESIAN_POINT ( 'NONE',  ( -5.895805022753480173, -59.44547149457074653, -4.407101234057782868 ) ) ;
#5773=CARTESIAN_POINT ( 'NONE',  ( 4.784657899331175912, -64.39547149457074227, -1.454677039711874009 ) ) ;
#5774=CARTESIAN_POINT ( 'NONE',  ( -1.529537955723778486, -62.14547149457074227, -5.030887037049945221 ) ) ;
#5778=CARTESIAN_POINT ( 'NONE',  ( 4.312004677471073855, -61.95452850542923784, 3.009306630940844496 ) ) ;
#5780=CARTESIAN_POINT ( 'NONE',  ( 7.360235569667880284, -91.24547149457073658, 0.09995255151716216091 ) ) ;
#5782=CARTESIAN_POINT ( 'NONE',  ( -4.784657899331190123, -78.60452850542925773, -1.454677039711773867 ) ) ;
#5787=CARTESIAN_POINT ( 'NONE',  ( 4.312004677471012570, -76.54547149457071953, -3.009306630940933314 ) ) ;
#5789=CARTESIAN_POINT ( 'NONE',  ( 0.09506052544077515931, -67.99547149457075079, -2.999999999999997780 ) ) ;
#5790=CARTESIAN_POINT ( 'NONE',  ( 7.360235569667877620, -65.25452850542926342, -0.09995255151731691212 ) ) ;
#5792=CARTESIAN_POINT ( 'NONE',  ( -0.09506052544073466393, -81.49547149457075079, 4.999999999999997335 ) ) ;
#5794=CARTESIAN_POINT ( 'NONE',  ( 0.09506052544086197875, -91.50452850542924921, 4.999999999999997335 ) ) ;
#5795=CARTESIAN_POINT ( 'NONE',  ( -2.179377348189461827, -70.35452850542922931, 7.030887037049988741 ) ) ;
#5796=CARTESIAN_POINT ( 'NONE',  ( 1.686450176301637960, -90.79547149457074795, 2.482926158054096000 ) ) ;
#5800=CARTESIAN_POINT ( 'NONE',  ( 4.725907263620341858, -92.40452850542925489, -1.635492904037697981 ) ) ;
#5802=CARTESIAN_POINT ( 'NONE',  ( -4.784657899331190123, -81.60452850542925773, -1.454677039711773867 ) ) ;
#5803=CARTESIAN_POINT ( 'NONE',  ( 2.823794231030038571, -62.40452850542925489, -1.017458915287783316 ) ) ;
#5805=CARTESIAN_POINT ( 'NONE',  ( 2.862020680886515400, -86.70452850542925205, -4.100960146804039752 ) ) ;
#5806=CARTESIAN_POINT ( 'NONE',  ( -2.179377348189612373, -68.14547149457074227, -7.030887037049939003 ) ) ;
#5807=CARTESIAN_POINT ( 'NONE',  ( -0.09506052544073466393, -81.49547149457075079, 4.999999999999997335 ) ) ;
#5808=CARTESIAN_POINT ( 'NONE',  ( 2.493201789345271369, -71.55452850542926058, -1.934965279058294518 ) ) ;
#5811=CARTESIAN_POINT ( 'NONE',  ( 0.8796985632579000791, -86.85452850542924352, -3.030887037049972310 ) ) ;
#5812=CARTESIAN_POINT ( 'NONE',  ( -6.686770931921461880, -59.89547149457074937, 2.072711028461789784 ) ) ;
#5815=CARTESIAN_POINT ( 'NONE',  ( 5.257311121191341918, -80.25452850542922079, -0.09995255151729465215 ) ) ;
#5816=CARTESIAN_POINT ( 'NONE',  ( -6.628020296210665130, -95.59547149457074511, -2.253526892787471869 ) ) ;
#5819=CARTESIAN_POINT ( 'NONE',  ( -4.784657899331192787, -57.60452850542925773, -1.454677039711773867 ) ) ;
#5820=CARTESIAN_POINT ( 'NONE',  ( -2.369498399071055861, -87.34547149457073090, 6.969112962950058332 ) ) ;
#5823=CARTESIAN_POINT ( 'NONE',  ( 4.194503406049335581, -71.55452850542926058, -3.171033256558100089 ) ) ;
#5833=CARTESIAN_POINT ( 'NONE',  ( -3.015831842038128041, -84.19547149457073942, 3.989209796945492048 ) ) ;
#5835=CARTESIAN_POINT ( 'NONE',  ( 1.686450176301633963, -60.79547149457074084, 2.482926158054096000 ) ) ;
#5836=CARTESIAN_POINT ( 'NONE',  ( -2.369498399071207739, -72.15452850542922647, -6.969112962950009482 ) ) ;
#5838=CARTESIAN_POINT ( 'NONE',  ( -5.257311121191324155, -80.74547149457075079, -0.09995255151718371311 ) ) ;
#5839=CARTESIAN_POINT ( 'NONE',  ( 4.784657899331207886, -62.10452850542925063, 1.454677039711774533 ) ) ;
#5840=CARTESIAN_POINT ( 'NONE',  ( 4.725907263620341858, -89.40452850542926910, -1.635492904037697981 ) ) ;
#5841=CARTESIAN_POINT ( 'NONE',  ( -6.686770931921506289, -72.60452850542924352, -2.072711028461647675 ) ) ;
#5843=CARTESIAN_POINT ( 'NONE',  ( 1.840261337453220625, -79.69547149457075363, -2.371175808195584267 ) ) ;
#5846=CARTESIAN_POINT ( 'NONE',  ( 4.312004677471079184, -94.95452850542926626, 3.009306630940844496 ) ) ;
#5847=CARTESIAN_POINT ( 'NONE',  ( -2.862020680886492752, -88.20452850542925205, 4.100960146804039752 ) ) ;
#5849=CARTESIAN_POINT ( 'NONE',  ( 2.862020680886514956, -80.70452850542925205, -4.100960146804039752 ) ) ;
#5850=CARTESIAN_POINT ( 'NONE',  ( -2.823794231030038571, -95.59547149457074511, -1.017458915287723364 ) ) ;
#5852=CARTESIAN_POINT ( 'NONE',  ( 3.015831842038234623, -82.80452850542926058, 3.989209796945429432 ) ) ;
#5853=CARTESIAN_POINT ( 'NONE',  ( -4.191402346623060104, -60.19547149457074653, 5.607243785695398941 ) ) ;
#5854=CARTESIAN_POINT ( 'NONE',  ( 1.840261337453269919, -70.80452850542926058, 2.371175808195547852 ) ) ;
#5857=CARTESIAN_POINT ( 'NONE',  ( -1.069819614139537078, -87.15452850542926910, -2.969112962950023249 ) ) ;
#5858=CARTESIAN_POINT ( 'NONE',  ( 5.895805022753409119, -95.55452850542926058, -4.407101234057908989 ) ) ;
#5860=CARTESIAN_POINT ( 'NONE',  ( -1.719659006605372076, -75.15452850542925489, -4.969112962950016588 ) ) ;
#5861=CARTESIAN_POINT ( 'NONE',  ( 6.013306294175080779, -91.54547149457074795, -4.245374608440741326 ) ) ;
#5864=CARTESIAN_POINT ( 'NONE',  ( -4.194503406049320482, -61.05452850542923926, 3.171033256558100533 ) ) ;
#5865=PRODUCT_DEFINITION ( 'UNKNOWN', '', #5369, #3509 ) ;
#5866=CARTESIAN_POINT ( 'NONE',  ( 6.628020296210689111, -91.09547149457074511, 2.253526892787472757 ) ) ;
#5867=ORIENTED_EDGE ( 'NONE', *, *, #2532, .F. ) ;
#5868=CARTESIAN_POINT ( 'NONE',  ( -4.725907263620321430, -75.90452850542925489, 1.635492904037698647 ) ) ;
#5873=CARTESIAN_POINT ( 'NONE',  ( -4.725907263620353405, -80.59547149457074511, -1.635492904037597617 ) ) ;
#5875=CARTESIAN_POINT ( 'NONE',  ( -0.09506052544075858923, -60.49547149457073658, 2.999999999999997780 ) ) ;
#5876=CARTESIAN_POINT ( 'NONE',  ( 5.895805022753404678, -71.55452850542926058, -4.407101234057908989 ) ) ;
#5878=CARTESIAN_POINT ( 'NONE',  ( -2.862020680886580681, -77.29547149457074795, -4.100960146803977580 ) ) ;
#5881=CARTESIAN_POINT ( 'NONE',  ( -2.862020680886493196, -85.20452850542925205, 4.100960146804039752 ) ) ;
#5882=CARTESIAN_POINT ( 'NONE',  ( 7.360235569667877620, -71.25452850542926342, -0.09995255151731691212 ) ) ;
#5883=CARTESIAN_POINT ( 'NONE',  ( -1.686450176301617310, -74.29547149457074795, -2.482926158054096000 ) ) ;
#5888=CARTESIAN_POINT ( 'NONE',  ( 4.194503406049339134, -92.55452850542924637, -3.171033256558100089 ) ) ;
#5890=CARTESIAN_POINT ( 'NONE',  ( -4.312004677471056979, -81.45452850542923784, -3.009306630940843608 ) ) ;
#5891=CARTESIAN_POINT ( 'NONE',  ( 3.154386672714810658, -88.24547149457073658, 0.09995255151720662534 ) ) ;
#5893=CARTESIAN_POINT ( 'NONE',  ( -3.015831842038213750, -84.30452850542926058, -3.989209796945429432 ) ) ;
#5894=CARTESIAN_POINT ( 'NONE',  ( 5.895805022753409119, -95.55452850542926058, -4.407101234057908989 ) ) ;
#5895=CARTESIAN_POINT ( 'NONE',  ( 2.610703060766982553, -64.95452850542926626, 1.773238653441072232 ) ) ;
#5899=CARTESIAN_POINT ( 'NONE',  ( 0.09506052544083844202, -73.50452850542924921, 2.999999999999997780 ) ) ;
#5900=CARTESIAN_POINT ( 'NONE',  ( -4.191402346623178232, -84.30452850542926058, -5.607243785695311900 ) ) ;
#5903=CARTESIAN_POINT ( 'NONE',  ( -4.191402346623055664, -90.19547149457073942, 5.607243785695398941 ) ) ;
#5906=CARTESIAN_POINT ( 'NONE',  ( -1.686450176301617976, -68.29547149457073374, -2.482926158054096000 ) ) ;
#5909=CARTESIAN_POINT ( 'NONE',  ( 1.529537955723688336, -59.85452850542924352, -5.030887037049978971 ) ) ;
#5911=CARTESIAN_POINT ( 'NONE',  ( -3.015831842038214639, -78.30452850542926058, -3.989209796945429432 ) ) ;
#5912=CARTESIAN_POINT ( 'NONE',  ( 6.628020296210689111, -94.09547149457074511, 2.253526892787472757 ) ) ;
#5916=CARTESIAN_POINT ( 'NONE',  ( -5.257311121191324155, -72.75452850542924921, 0.09995255151729526277 ) ) ;
#5921=CARTESIAN_POINT ( 'NONE',  ( -4.784657899331157260, -80.89547149457074227, 1.454677039711874675 ) ) ;
#5922=CARTESIAN_POINT ( 'NONE',  ( 1.488389562037239156, -97.00000000000000000, -3.748545376255541850 ) ) ;
#5923=CARTESIAN_POINT ( 'NONE',  ( -0.8796985632579451542, -59.14547149457074227, -3.030887037049952326 ) ) ;
#5924=CARTESIAN_POINT ( 'NONE',  ( 6.686770931921523164, -68.10452850542924352, 2.072711028461649008 ) ) ;
#5926=CARTESIAN_POINT ( 'NONE',  ( 0.09506052544075525856, -76.99547149457073658, -4.999999999999997335 ) ) ;
#5928=CARTESIAN_POINT ( 'NONE',  ( 4.725907263620340970, -83.40452850542925489, -1.635492904037697981 ) ) ;
#5929=CARTESIAN_POINT ( 'NONE',  ( 6.686770931921523164, -71.10452850542924352, 2.072711028461649008 ) ) ;
#5930=CARTESIAN_POINT ( 'NONE',  ( 0.09506052544077665811, -79.99547149457075079, -2.999999999999997780 ) ) ;
#5934=CARTESIAN_POINT ( 'NONE',  ( 1.529537955723691001, -83.85452850542927195, -5.030887037049978971 ) ) ;
#5936=CARTESIAN_POINT ( 'NONE',  ( 1.719659006605391172, -79.65452850542925489, 4.969112962950015699 ) ) ;
#5937=CARTESIAN_POINT ( 'NONE',  ( -2.882544866740855749, -89.89547149457074227, 0.8366430509619596778 ) ) ;
#5939=CARTESIAN_POINT ( 'NONE',  ( 5.257311121191342806, -89.25452850542924921, -0.09995255151729465215 ) ) ;
#5940=CARTESIAN_POINT ( 'NONE',  ( 2.369498399071075401, -61.84547149457074511, -6.969112962950057444 ) ) ;
#5941=CARTESIAN_POINT ( 'NONE',  ( 2.882544866740895717, -68.10452850542924352, 0.8366430509618999478 ) ) ;
#5946=CARTESIAN_POINT ( 'NONE',  ( 2.493201789345272257, -80.55452850542926058, -1.934965279058294518 ) ) ;
#5947=CARTESIAN_POINT ( 'NONE',  ( 4.191402346623198660, -85.80452850542926058, 5.607243785695311900 ) ) ;
#5949=CARTESIAN_POINT ( 'NONE',  ( -2.369498399071054529, -93.34547149457073090, 6.969112962950058332 ) ) ;
#5952=CARTESIAN_POINT ( 'NONE',  ( -1.686450176301617976, -71.29547149457074795, -2.482926158054096000 ) ) ;
#5953=CARTESIAN_POINT ( 'NONE',  ( -1.719659006605374962, -57.15452850542924068, -4.969112962950016588 ) ) ;
#5955=CARTESIAN_POINT ( 'NONE',  ( -4.784657899331191011, -69.60452850542925773, -1.454677039711773867 ) ) ;
#5956=CARTESIAN_POINT ( 'NONE',  ( -6.628020296210666018, -83.59547149457075932, -2.253526892787471869 ) ) ;
#5958=CARTESIAN_POINT ( 'NONE',  ( 4.312004677471076519, -79.95452850542922363, 3.009306630940844496 ) ) ;
#5960=( BOUNDED_SURFACE ( )  B_SPLINE_SURFACE ( 3, 2, ( 
 ( #7840, #834, #161, #4040, #6607, #7283, #3996, #5846, #240, #1343, #2740, #4619, #5978, #2657, #4663, #4077, #5302, #5340, #7885, #202, #7160, #2109, #2781, #5384, #3914, #1509, #6482, #3287, #6180, #1552, #1636, #3488, #7491, #1042, #4833, #4157, #8126, #3612, #7411, #6095, #4196, #4116, #2901, #6058, #2314, #1592, #3021, #6221, #1001, #5506, #8087, #5583, #405, #322, #4878, #8164, #3567, #283, #1719, #4278, #2860, #5466, #6137, #6685, #916, #6728, #6851, #958, #2392, #1082, #3652, #7326, #5423, #7449, #3527, #8005, #7362, #2233, #5545, #2272, #4789, #1680, #8045, #4919, #6766, #362, #2939, #4240, #6808, #2979, #2357, #444, #6305, #4439, #4396, #7655, #1889, #5743, #5037, #1121, #4480, #4952, #1209, #3735, #7019, #3696, #8283, #7695, #2474, #606, #3779, #1246, #8202, #526, #6974, #1927, #1287, #3817, #5911, #6266, #6389, #7530, #7611, #484, #5118, #3188, #1846, #1803, #8324, #2557, #6349, #3105, #567, #1761, #5661, #3061, #2512, #7567, #770, #3857, #3145, #5702, #5076, #3350, #7060, #8242, #6427, #141, #4316, #5621, #6887, #2433, #4995, #4359, #6933, #1167, #4644, #5323, #8030, #2130, #5404, #2764, #4102, #7264, #2089, #182, #2802, #1491, #7906, #4682, #2257, #4772, #4059, #1575, #6627, #3473, #5955, #4813, #6589, #7390, #983, #4181, #2172, #3397, #855, #6751, #817, #1619, #3436, #5363, #4725, #7306, #5998, #223, #1448, #6039, #2214, #7947, #7348, #1531, #7986, #4141, #3513, #6669, #7226, #3550, #2722, #900, #263, #6709, #4018, #2845, #5451, #941, #6081, #306, #2883, #6121, #5280, #7862, #5647, #5018, #3045, #1190, #1661, #7553, #2924, #3001, #4860, #506, #2415, #6203, #5529, #1150, #4978, #427, #7475, #5567, #5489, #4260, #7432, #3676, #2964, #4382, #7594, #2377, #6874, #1103, #6957, #1784, #1704, #6247, #3760, #4939, #4221, #3084, #8226, #6794, #6832, #7513, #8069 ),
 ( #469, #1025, #3592, #2456, #8109, #8150, #6917, #3720, #1829, #6162, #385, #6290, #5606, #1064, #1743, #2336, #345, #4302, #8187, #4340, #2299, #4903, #3638, #3883, #1356, #3801, #4462, #4418, #7042, #1312, #7171, #5187, #5684, #1273, #4506, #7001, #3301, #6454, #2669, #3212, #3171, #7809, #3926, #7085, #40, #86, #5100, #7765, #2537, #1871, #676, #3256, #2040, #2579, #1230, #5140, #3128, #8267, #592, #5857, #5726, #5811, #6371, #7720, #7679, #2498, #8304, #6411, #1911, #3842, #629, #5226, #2628, #5770, #1996, #8337, #4546, #1956, #4588, #7129, #1395, #6333, #551, #6493, #715, #5059, #7637, #7852, #296, #2752, #4051, #5990, #213, #4674, #5313, #2713, #7296, #2247, #3502, #2873, #4802, #2078, #4091, #5946, #5271, #4008, #6537, #2203, #7254, #131, #1523, #7377, #1564, #4633, #2793, #7216, #759, #1440, #6577, #6029, #3464, #7896, #253, #3425, #6661, #890, #4758, #6619, #808, #6072, #3968, #5353, #2121, #2835, #3388, #5396, #6698, #1483, #7977, #7936, #7339, #172, #846, #2163, #929, #5439, #4130, #3341, #4716, #8020, #5899, #4252, #6110, #1774, #3666, #7466, #6784, #2407, #6234, #1695, #377, #6822, #4171, #5521, #336, #4932, #4210, #5638, #498, #3626, #8141, #2369, #8219, #460, #2953, #7505, #2447, #6193, #2913, #4329, #6903, #5480, #8102, #7425, #1055, #6151, #1016, #1651, #1141, #3034, #2328, #5596, #3584, #1735, #4849, #3710, #8059, #6280, #5009, #3076, #419, #2286, #4891, #1606, #2992, #6742, #5558, #4292, #6864, #1094, #8178, #4968, #7544, #972, #3540, #7119, #3918, #78, #3120, #7712, #1224, #542, #7627, #1821, #5803, #2528, #3749, #5133, #2661, #5177, #6323, #6404, #5675, #4373, #8257, #1862, #1304, #7077, #582, #3874, #7034, #1945, #4498, #32, #7671, #2491, #1347, #7582, #3834, #6365, #6443, #5052, #2572, #1988, #5091, #3247, #622, #664, #4410, #3164, #1262 ),
 ( #6992, #7756, #2615, #1904, #3793, #4538, #6486, #4453, #5719, #3203, #6948, #8298, #5759, #707, #4293, #3291, #5850, #1181, #3418, #5982, #3492, #4081, #4000, #206, #6063, #7248, #6530, #5388, #7969, #752, #796, #4044, #2031, #7164, #7844, #2194, #4623, #7929, #5263, #6611, #1433, #4580, #1387, #3958, #2071, #4746, #7208, #2155, #6570, #838, #3378, #3333, #2704, #5306, #5937, #165, #2745, #7330, #7287, #7889, #6653, #2113, #2785, #121, #1556, #5891, #4121, #287, #6689, #4667, #1474, #5344, #920, #4709, #5219, #1513, #882, #3456, #6020, #244, #2824, #7799, #6183, #1125, #2396, #7533, #3699, #6732, #2982, #4837, #4161, #2905, #5427, #1085, #6140, #7367, #409, #6269, #447, #1596, #1683, #963, #8009, #3531, #5470, #4922, #2360, #4200, #7494, #2317, #5549, #8130, #3656, #2942, #6099, #4956, #2864, #7453, #1640, #1723, #326, #4281, #5586, #365, #6854, #4243, #6225, #8049, #6770, #4881, #8167, #1764, #3024, #2237, #2276, #4319, #4793, #5509, #7415, #6892, #1005, #8090, #3571, #6812, #1045, #3615, #7614, #5705, #3064, #4399, #4998, #3821, #3109, #4524, #7741, #2515, #7022, #1249, #7104, #7698, #1849, #6393, #1330, #5079, #1807, #648, #3232, #4362, #6977, #7658, #5625, #7063, #3782, #7570, #609, #3903, #6430, #6936, #1892, #1170, #8206, #3738, #5664, #2560, #8327, #1212, #5121, #8286, #3191, #5746, #1291, #570, #6308, #17, #487, #4442, #6352, #1930, #530, #4483, #5789, #3150, #3860, #2599, #5162, #8245, #1973, #2436, #2478, #5041, #824, #7313, #7784, #5332, #691, #782, #2646, #6636, #193, #3986, #3318, #7274, #2772, #6554, #5246, #3362, #3275, #2058, #5203, #1457, #738, #2181, #5372, #149, #4653, #7234, #4734, #7914, #7830, #4029, #1542, #2731, #2013, #868, #3444, #4565, #4606, #5289, #5835, #63, #5875, #6007, #105, #3404, #6514, #7874, #2689, #7150, #3942, #5923, #7193 ),
 ( #1373, #232, #1417, #2810, #6472, #7955, #2100, #6598, #5965, #2140, #4693, #1500, #4067, #6050, #274, #2853, #5415, #3480, #6678, #7995, #7357, #4782, #4110, #909, #2226, #5662, #445, #4397, #4440, #4996, #6852, #485, #7656, #8203, #6350, #4317, #2980, #2358, #8128, #5546, #3062, #6888, #3106, #3780, #2394, #4920, #6222, #528, #3697, #7531, #7020, #7568, #6267, #6975, #1083, #1805, #7492, #2434, #8243, #5038, #4360, #5623, #1847, #1762, #1720, #6934, #1247, #3819, #4279, #3653, #3022, #568, #1210, #3147, #1168, #2476, #5584, #6390, #6306, #8165, #4953, #8284, #1123, #3736, #5703, #2513, #5077, #7612, #1890, #6552, #6512, #1971, #5833, #15, #7191, #2011, #736, #5201, #689, #6428, #8325, #3316, #3984, #645, #7102, #7061, #1327, #3940, #1455, #7827, #2558, #3901, #7148, #1288, #5921, #4521, #5873, #3230, #2056, #2098, #780, #1371, #2687, #2728, #7739, #4604, #5160, #4481, #103, #5244, #4651, #7781, #3858, #147, #7232, #5744, #6470, #1415, #3273, #3360, #5119, #61, #4563, #5787, #607, #7872, #2597, #5287, #7696, #4027, #2644, #3189, #1928, #2808, #2264, #5962, #1583, #6720, #2138, #2307, #4148, #2770, #5330, #3560, #6005, #4107, #4821, #1629, #6129, #4691, #6634, #4190, #951, #7953, #3478, #230, #7402, #7993, #3520, #2851, #6676, #4065, #191, #6089, #6760, #865, #4732, #7272, #7311, #313, #7442, #5459, #7912, #1540, #4780, #1498, #354, #2179, #2893, #3442, #8037, #8079, #993, #7355, #2931, #5496, #5370, #4870, #907, #6048, #1669, #6596, #822, #5413, #272, #3402, #2224, #1033, #1755, #5030, #3012, #517, #398, #437, #479, #7483, #4232, #3137, #8119, #7604, #3602, #4988, #4912, #5578, #3054, #8158, #8235, #6169, #7562, #6259, #2346, #4310, #559, #1114, #1840, #2387, #6801, #2971, #5536, #1711, #6882, #4947, #4351, #4390, #3646, #4269, #6841, #1796, #7522, #3687, #8277 ),
 ( #6299, #5616, #8195, #3098, #2427, #1074, #6927, #2506, #5068, #6212, #1161, #3729, #6967, #5655, #1199, #2466, #3770, #6342, #5694, #7647, #7774, #5195, #3351, #6464, #2547, #1407, #5912, #7012, #7732, #2679, #639, #6503, #6381, #6420, #684, #5111, #1881, #771, #5734, #5237, #1239, #2638, #7687, #3223, #3264, #5780, #5866, #3809, #2004, #3894, #8317, #1965, #6547, #7094, #7821, #8, #4430, #600, #3181, #1921, #4514, #2587, #4556, #2049, #1281, #4473, #7053, #7141, #5151, #1321, #142, #5820, #54, #96, #3850, #1365, #3934, #728, #3310, #4598, #7182, #3978, #2723, #5281, #7863, #3474, #3551, #346, #4019, #3398, #6590, #307, #6711, #8031, #1532, #7987, #5956, #6122, #2846, #818, #183, #4814, #7265, #5364, #6082, #2884, #7392, #2765, #7907, #5452, #5405, #856, #4726, #1492, #2258, #901, #2215, #4103, #7948, #5324, #7227, #4773, #1620, #2131, #5999, #4683, #224, #7349, #2925, #942, #1449, #2803, #6040, #4060, #4182, #3437, #1576, #6628, #3514, #984, #6752, #264, #4142, #2090, #2173, #4645, #7307, #6670, #1662, #2457, #4904, #3002, #3721, #507, #5019, #1026, #5530, #3087, #3046, #6833, #2378, #7476, #6291, #6875, #5607, #1745, #5568, #2965, #4861, #8188, #5648, #8110, #3639, #3593, #6204, #470, #6334, #4341, #7433, #428, #3677, #6163, #7595, #1065, #2417, #2337, #6918, #6958, #8227, #6248, #7554, #1830, #4261, #1151, #1705, #387, #4979, #1785, #1191, #4303, #8151, #4383, #3762, #2300, #4940, #552, #7514, #5490, #4222, #1104, #8071, #6795, #3129, #2042, #7002, #3927, #8268, #3885, #3802, #7680, #1957, #1912, #7131, #2499, #6455, #5141, #1231, #630, #7810, #1, #6494, #4463, #5685, #5060, #7638, #1872, #3213, #7043, #3257, #717, #2538, #4420, #6372, #677, #3843, #1274, #7172, #7721, #6412, #1357, #593, #4507, #3172, #2580, #5812, #5188, #7086, #5771, #1997, #1313, #5727 ),
 ( #3302, #41, #2629, #5858, #7766, #8305, #5102, #4547, #87, #2670, #5227, #4589, #1397, #3969, #6538, #4009, #6662, #1484, #5314, #4803, #2794, #4052, #4760, #7217, #5354, #132, #5991, #3465, #2836, #7937, #6620, #7978, #7897, #760, #4717, #7379, #1607, #5272, #4634, #7853, #1565, #2204, #930, #2164, #891, #1441, #4172, #4093, #2079, #6578, #6073, #173, #847, #7340, #4131, #297, #809, #3389, #6699, #6030, #2122, #214, #2754, #3503, #7297, #254, #1524, #3427, #5947, #2714, #5397, #2874, #4675, #7255, #5440, #8021, #2248, #3342, #5900, #6111, #1808, #5042, #4957, #3822, #2437, #1213, #4320, #8287, #8329, #4443, #7615, #571, #610, #5627, #5706, #3065, #2397, #4400, #1850, #2561, #3110, #7534, #6394, #5122, #3541, #4363, #7660, #8207, #3151, #2914, #4999, #5665, #1765, #6743, #5747, #6893, #1893, #337, #6979, #1126, #7571, #8246, #6937, #2516, #5587, #3783, #531, #3700, #1171, #3192, #3739, #6310, #973, #2479, #7699, #1931, #8168, #6270, #488, #7023, #5080, #1250, #6353, #4607, #18, #194, #7831, #650, #3233, #1458, #3904, #2015, #2732, #7875, #4031, #2600, #4525, #2101, #2059, #5836, #1374, #6473, #5290, #5876, #7194, #739, #4566, #1974, #3861, #1418, #4654, #7105, #2647, #5163, #5204, #3987, #5333, #3364, #6431, #7785, #2691, #7742, #6599, #64, #6555, #1332, #5924, #5966, #7235, #5247, #783, #825, #3276, #150, #692, #7151, #3405, #2773, #7915, #3319, #3943, #4484, #7064, #1292, #6515, #5790, #106, #6761, #6637, #6679, #6722, #5373, #2141, #1035, #6008, #2934, #7275, #2895, #2811, #910, #953, #3481, #6130, #1501, #5460, #4151, #233, #7997, #6803, #7358, #5498, #6051, #4694, #4068, #869, #3445, #2227, #275, #2267, #8080, #1543, #7956, #2182, #8039, #2854, #5416, #6171, #3522, #4783, #355, #4735, #6090, #7315, #1586, #4823, #4191, #315, #7405, #995, #4111, #1631 ),
 ( #2309, #3562, #4872, #7444, #1672, #4234, #3605, #400, #2973, #5539, #4914, #8121, #3647, #439, #7485, #4271, #1713, #6842, #1075, #2349, #6213, #3013, #2658, #5888, #5800, #4664, #3288, #2068, #5174, #793, #835, #5303, #118, #1430, #1471, #6483, #6567, #3915, #3244, #5260, #2701, #3415, #3955, #29, #7245, #5979, #4495, #5216, #162, #704, #3997, #3871, #5847, #6527, #2612, #7709, #6608, #7753, #2741, #7074, #7841, #1985, #75, #749, #7796, #3375, #1301, #4620, #1384, #4535, #2028, #4041, #4577, #7886, #7161, #1942, #6440, #661, #7116, #3330, #7205, #5934, #2110, #1344, #203, #2782, #2902, #6059, #1553, #1043, #7363, #284, #1002, #3453, #1593, #4706, #2234, #8046, #7412, #4158, #2861, #4197, #4117, #5341, #959, #3613, #6181, #1510, #878, #4078, #6138, #6767, #5507, #6729, #5467, #6017, #406, #323, #6650, #8088, #2315, #241, #917, #3528, #2152, #7284, #7966, #4879, #4743, #2273, #5385, #6096, #6686, #2820, #2191, #5424, #3489, #7327, #8006, #7451, #1637, #4790, #3568, #4834, #363, #2940, #1681, #4241, #6809, #7926, #1280, #7646, #3136, #3686, #5576, #3769, #1237, #6257, #4350, #4309, #6926, #1198, #7052, #5067, #8157, #1160, #4389, #6881, #3179, #1795, #558, #478, #1879, #7686, #3808, #6966, #8276, #8316, #4987, #4427, #2425, #1753, #6340, #5693, #1920, #2465, #1113, #5733, #4471, #3010, #3728, #7011, #7561, #2505, #2386, #6298, #5029, #3053, #6211, #5109, #5615, #6380, #4946, #599, #8194, #516, #7603, #3096, #2546, #7521, #436, #8234, #5654, #1839, #179, #727, #7224, #5194, #3849, #3222, #638, #6419, #3933, #7772, #3977, #4642, #3263, #5778, #7092, #1406, #4554, #53, #7904, #5864, #7139, #7860, #1964, #95, #7, #3308, #6545, #5909, #2678, #1364, #2720, #2636, #2586, #1319, #6501, #2003, #6463, #3893, #3395, #139, #5236, #5278, #5819, #4597, #683, #5953, #7730 ) ),
 .UNSPECIFIED., .T., .F., .T. ) 
 B_SPLINE_SURFACE_WITH_KNOTS ( ( 4, 3, 4 ),
 ( 3, 2, 2, 2, 2, 2, 2, 2, 2, 2, 2, 2, 2, 2, 2, 2, 2, 2, 2, 2, 2, 2, 2, 2, 2, 2, 2, 2, 2, 2, 2, 2, 2, 2, 2, 2, 2, 2, 2, 2, 2, 2, 2, 2, 2, 2, 2, 2, 2, 2, 2, 2, 2, 2, 2, 2, 2, 2, 2, 2, 2, 2, 2, 2, 2, 2, 2, 2, 2, 2, 2, 2, 2, 2, 2, 2, 2, 2, 2, 2, 2, 2, 2, 2, 2, 2, 2, 2, 2, 2, 2, 2, 2, 2, 2, 2, 2, 2, 2, 2, 2, 2, 2, 2, 2, 2, 2, 2, 2, 2, 2, 2, 2, 2, 2, 2, 2, 2, 2, 2, 2, 2, 2, 2, 2, 2, 2, 2, 2, 2, 3 ),
 ( 0.000000000000000000, 0.5000000000000000000, 1.000000000000000000 ),
 ( 0.000000000000000000, 0.007692307692307692735, 0.01538461538461538547, 0.02307692307692307820, 0.03076923076923077094, 0.03846153846153846367, 0.04615384615384615641, 0.05384615384615384914, 0.06153846153846154188, 0.06923076923076923461, 0.07692307692307692735, 0.08461538461538462008, 0.09230769230769231282, 0.1000000000000000056, 0.1076923076923076983, 0.1153846153846153910, 0.1230769230769230838, 0.1307692307692307765, 0.1384615384615384692, 0.1461538461538461620, 0.1538461538461538547, 0.1615384615384615474, 0.1692307692307692402, 0.1769230769230769329, 0.1846153846153846256, 0.1923076923076923184, 0.2000000000000000111, 0.2076923076923077038, 0.2153846153846153966, 0.2230769230769230893, 0.2307692307692307820, 0.2384615384615384748, 0.2461538461538461675, 0.2538461538461538325, 0.2615384615384615530, 0.2692307692307692180, 0.2769230769230769384, 0.2846153846153846034, 0.2923076923076923239, 0.2999999999999999889, 0.3076923076923077094, 0.3153846153846153744, 0.3230769230769230949, 0.3307692307692307598, 0.3384615384615384803, 0.3461538461538461453, 0.3538461538461538658, 0.3615384615384615308, 0.3692307692307692513, 0.3769230769230769162, 0.3846153846153846367, 0.3923076923076923017, 0.4000000000000000222, 0.4076923076923076872, 0.4153846153846154077, 0.4230769230769230727, 0.4307692307692307931, 0.4384615384615384581, 0.4461538461538461786, 0.4538461538461538436, 0.4615384615384615641, 0.4692307692307692291, 0.4769230769230769496, 0.4846153846153846145, 0.4923076923076923350, 0.5000000000000000000, 0.5076923076923076650, 0.5153846153846153300, 0.5230769230769231060, 0.5307692307692307709, 0.5384615384615384359, 0.5461538461538461009, 0.5538461538461538769, 0.5615384615384615419, 0.5692307692307692069, 0.5769230769230768718, 0.5846153846153846478, 0.5923076923076923128, 0.5999999999999999778, 0.6076923076923076428, 0.6153846153846154188, 0.6230769230769230838, 0.6307692307692307487, 0.6384615384615384137, 0.6461538461538461897, 0.6538461538461538547, 0.6615384615384615197, 0.6692307692307691847, 0.6769230769230769607, 0.6846153846153846256, 0.6923076923076922906, 0.6999999999999999556, 0.7076923076923077316, 0.7153846153846153966, 0.7230769230769230616, 0.7307692307692307265, 0.7384615384615385025, 0.7461538461538461675, 0.7538461538461538325, 0.7615384615384614975, 0.7692307692307692735, 0.7769230769230769384, 0.7846153846153846034, 0.7923076923076922684, 0.8000000000000000444, 0.8076923076923077094, 0.8153846153846153744, 0.8230769230769230393, 0.8307692307692308153, 0.8384615384615384803, 0.8461538461538461453, 0.8538461538461538103, 0.8615384615384615863, 0.8692307692307692513, 0.8769230769230769162, 0.8846153846153845812, 0.8923076923076923572, 0.9000000000000000222, 0.9076923076923076872, 0.9153846153846153522, 0.9230769230769231282, 0.9307692307692307931, 0.9384615384615384581, 0.9461538461538461231, 0.9538461538461538991, 0.9615384615384615641, 0.9692307692307692291, 0.9769230769230768940, 0.9846153846153846700, 0.9923076923076923350, 1.000000000000000000 ),
 .UNSPECIFIED. ) 
 GEOMETRIC_REPRESENTATION_ITEM ( )  RATIONAL_B_SPLINE_SURFACE ( (
 ( 1.000000000000000000, 0.9510565162951535312, 1.000000000000000000, 0.9510565162951535312, 1.000000000000000000, 0.9510565162951535312, 1.000000000000000000, 0.9510565162951535312, 1.000000000000000000, 0.9510565162951535312, 1.000000000000000000, 0.9510565162951535312, 1.000000000000000000, 0.9510565162951535312, 1.000000000000000000, 0.9510565162951535312, 1.000000000000000000, 0.9510565162951535312, 1.000000000000000000, 0.9510565162951535312, 1.000000000000000000, 0.9510565162951535312, 1.000000000000000000, 0.9510565162951535312, 1.000000000000000000, 0.9510565162951535312, 1.000000000000000000, 0.9510565162951535312, 1.000000000000000000, 0.9510565162951535312, 1.000000000000000000, 0.9510565162951535312, 1.000000000000000000, 0.9510565162951535312, 1.000000000000000000, 0.9510565162951535312, 1.000000000000000000, 0.9510565162951535312, 1.000000000000000000, 0.9510565162951535312, 1.000000000000000000, 0.9510565162951535312, 1.000000000000000000, 0.9510565162951535312, 1.000000000000000000, 0.9510565162951535312, 1.000000000000000000, 0.9510565162951535312, 1.000000000000000000, 0.9510565162951535312, 1.000000000000000000, 0.9510565162951535312, 1.000000000000000000, 0.9510565162951535312, 1.000000000000000000, 0.9510565162951535312, 1.000000000000000000, 0.9510565162951535312, 1.000000000000000000, 0.9510565162951535312, 1.000000000000000000, 0.9510565162951535312, 1.000000000000000000, 0.9510565162951535312, 1.000000000000000000, 0.9510565162951535312, 1.000000000000000000, 0.9510565162951535312, 1.000000000000000000, 0.9510565162951535312, 1.000000000000000000, 0.9510565162951535312, 1.000000000000000000, 0.9510565162951535312, 1.000000000000000000, 0.9510565162951535312, 1.000000000000000000, 0.9510565162951535312, 1.000000000000000000, 0.9510565162951535312, 1.000000000000000000, 0.9510565162951535312, 1.000000000000000000, 0.9510565162951535312, 1.000000000000000000, 0.9510565162951535312, 1.000000000000000000, 0.9510565162951535312, 1.000000000000000000, 0.9510565162951535312, 1.000000000000000000, 0.9510565162951535312, 1.000000000000000000, 0.9510565162951535312, 1.000000000000000000, 0.9510565162951535312, 1.000000000000000000, 0.9510565162951535312, 1.000000000000000000, 0.9510565162951535312, 1.000000000000000000, 0.9510565162951535312, 1.000000000000000000, 0.9510565162951535312, 1.000000000000000000, 0.9510565162951535312, 1.000000000000000000, 0.9510565162951535312, 1.000000000000000000, 0.9510565162951535312, 1.000000000000000000, 0.9510565162951535312, 1.000000000000000000, 0.9510565162951535312, 1.000000000000000000, 0.9510565162951535312, 1.000000000000000000, 0.9510565162951535312, 1.000000000000000000, 0.9510565162951535312, 1.000000000000000000, 0.9510565162951535312, 1.000000000000000000, 0.9510565162951535312, 1.000000000000000000, 0.9510565162951535312, 1.000000000000000000, 0.9510565162951535312, 1.000000000000000000, 0.9510565162951535312, 1.000000000000000000, 0.9510565162951535312, 1.000000000000000000, 0.9510565162951535312, 1.000000000000000000, 0.9510565162951535312, 1.000000000000000000, 0.9510565162951535312, 1.000000000000000000, 0.9510565162951535312, 1.000000000000000000, 0.9510565162951535312, 1.000000000000000000, 0.9510565162951535312, 1.000000000000000000, 0.9510565162951535312, 1.000000000000000000, 0.9510565162951535312, 1.000000000000000000, 0.9510565162951535312, 1.000000000000000000, 0.9510565162951535312, 1.000000000000000000, 0.9510565162951535312, 1.000000000000000000, 0.9510565162951535312, 1.000000000000000000, 0.9510565162951535312, 1.000000000000000000, 0.9510565162951535312, 1.000000000000000000, 0.9510565162951535312, 1.000000000000000000, 0.9510565162951535312, 1.000000000000000000, 0.9510565162951535312, 1.000000000000000000, 0.9510565162951535312, 1.000000000000000000, 0.9510565162951535312, 1.000000000000000000, 0.9510565162951535312, 1.000000000000000000, 0.9510565162951535312, 1.000000000000000000, 0.9510565162951535312, 1.000000000000000000, 0.9510565162951535312, 1.000000000000000000, 0.9510565162951535312, 1.000000000000000000, 0.9510565162951535312, 1.000000000000000000, 0.9510565162951535312, 1.000000000000000000, 0.9510565162951535312, 1.000000000000000000, 0.9510565162951535312, 1.000000000000000000, 0.9510565162951535312, 1.000000000000000000, 0.9510565162951535312, 1.000000000000000000, 0.9510565162951535312, 1.000000000000000000, 0.9510565162951535312, 1.000000000000000000, 0.9510565162951535312, 1.000000000000000000, 0.9510565162951535312, 1.000000000000000000, 0.9510565162951535312, 1.000000000000000000, 0.9510565162951535312, 1.000000000000000000, 0.9510565162951535312, 1.000000000000000000, 0.9510565162951535312, 1.000000000000000000, 0.9510565162951535312, 1.000000000000000000, 0.9510565162951535312, 1.000000000000000000, 0.9510565162951535312, 1.000000000000000000, 0.9510565162951535312, 1.000000000000000000, 0.9510565162951535312, 1.000000000000000000, 0.9510565162951535312, 1.000000000000000000, 0.9510565162951535312, 1.000000000000000000, 0.9510565162951535312, 1.000000000000000000, 0.9510565162951535312, 1.000000000000000000, 0.9510565162951535312, 1.000000000000000000, 0.9510565162951535312, 1.000000000000000000, 0.9510565162951535312, 1.000000000000000000, 0.9510565162951535312, 1.000000000000000000, 0.9510565162951535312, 1.000000000000000000, 0.9510565162951535312, 1.000000000000000000, 0.9510565162951535312, 1.000000000000000000, 0.9510565162951535312, 1.000000000000000000, 0.9510565162951535312, 1.000000000000000000, 0.9510565162951535312, 1.000000000000000000, 0.9510565162951535312, 1.000000000000000000, 0.9510565162951535312, 1.000000000000000000, 0.9510565162951535312, 1.000000000000000000, 0.9510565162951535312, 1.000000000000000000, 0.9510565162951535312, 1.000000000000000000, 0.9510565162951535312, 1.000000000000000000, 0.9510565162951535312, 1.000000000000000000),
 ( 0.3333333333333333703, 0.3170188387650512141, 0.3333333333333333703, 0.3170188387650512141, 0.3333333333333333703, 0.3170188387650512141, 0.3333333333333333703, 0.3170188387650512141, 0.3333333333333333703, 0.3170188387650512141, 0.3333333333333333703, 0.3170188387650512141, 0.3333333333333333703, 0.3170188387650512141, 0.3333333333333333703, 0.3170188387650512141, 0.3333333333333333703, 0.3170188387650512141, 0.3333333333333333703, 0.3170188387650512141, 0.3333333333333333703, 0.3170188387650512141, 0.3333333333333333703, 0.3170188387650512141, 0.3333333333333333703, 0.3170188387650512141, 0.3333333333333333703, 0.3170188387650512141, 0.3333333333333333703, 0.3170188387650512141, 0.3333333333333333703, 0.3170188387650512141, 0.3333333333333333703, 0.3170188387650512141, 0.3333333333333333703, 0.3170188387650512141, 0.3333333333333333703, 0.3170188387650512141, 0.3333333333333333703, 0.3170188387650512141, 0.3333333333333333703, 0.3170188387650512141, 0.3333333333333333703, 0.3170188387650512141, 0.3333333333333333703, 0.3170188387650512141, 0.3333333333333333703, 0.3170188387650512141, 0.3333333333333333703, 0.3170188387650512141, 0.3333333333333333703, 0.3170188387650512141, 0.3333333333333333703, 0.3170188387650512141, 0.3333333333333333703, 0.3170188387650512141, 0.3333333333333333703, 0.3170188387650512141, 0.3333333333333333703, 0.3170188387650512141, 0.3333333333333333703, 0.3170188387650512141, 0.3333333333333333703, 0.3170188387650512141, 0.3333333333333333703, 0.3170188387650512141, 0.3333333333333333703, 0.3170188387650512141, 0.3333333333333333703, 0.3170188387650512141, 0.3333333333333333703, 0.3170188387650512141, 0.3333333333333333703, 0.3170188387650512141, 0.3333333333333333703, 0.3170188387650512141, 0.3333333333333333703, 0.3170188387650512141, 0.3333333333333333703, 0.3170188387650512141, 0.3333333333333333703, 0.3170188387650512141, 0.3333333333333333703, 0.3170188387650512141, 0.3333333333333333703, 0.3170188387650512141, 0.3333333333333333703, 0.3170188387650512141, 0.3333333333333333703, 0.3170188387650512141, 0.3333333333333333703, 0.3170188387650512141, 0.3333333333333333703, 0.3170188387650512141, 0.3333333333333333703, 0.3170188387650512141, 0.3333333333333333703, 0.3170188387650512141, 0.3333333333333333703, 0.3170188387650512141, 0.3333333333333333703, 0.3170188387650512141, 0.3333333333333333703, 0.3170188387650512141, 0.3333333333333333703, 0.3170188387650512141, 0.3333333333333333703, 0.3170188387650512141, 0.3333333333333333703, 0.3170188387650512141, 0.3333333333333333703, 0.3170188387650512141, 0.3333333333333333703, 0.3170188387650512141, 0.3333333333333333703, 0.3170188387650512141, 0.3333333333333333703, 0.3170188387650512141, 0.3333333333333333703, 0.3170188387650512141, 0.3333333333333333703, 0.3170188387650512141, 0.3333333333333333703, 0.3170188387650512141, 0.3333333333333333703, 0.3170188387650512141, 0.3333333333333333703, 0.3170188387650512141, 0.3333333333333333703, 0.3170188387650512141, 0.3333333333333333703, 0.3170188387650512141, 0.3333333333333333703, 0.3170188387650512141, 0.3333333333333333703, 0.3170188387650512141, 0.3333333333333333703, 0.3170188387650512141, 0.3333333333333333703, 0.3170188387650512141, 0.3333333333333333703, 0.3170188387650512141, 0.3333333333333333703, 0.3170188387650512141, 0.3333333333333333703, 0.3170188387650512141, 0.3333333333333333703, 0.3170188387650512141, 0.3333333333333333703, 0.3170188387650512141, 0.3333333333333333703, 0.3170188387650512141, 0.3333333333333333703, 0.3170188387650512141, 0.3333333333333333703, 0.3170188387650512141, 0.3333333333333333703, 0.3170188387650512141, 0.3333333333333333703, 0.3170188387650512141, 0.3333333333333333703, 0.3170188387650512141, 0.3333333333333333703, 0.3170188387650512141, 0.3333333333333333703, 0.3170188387650512141, 0.3333333333333333703, 0.3170188387650512141, 0.3333333333333333703, 0.3170188387650512141, 0.3333333333333333703, 0.3170188387650512141, 0.3333333333333333703, 0.3170188387650512141, 0.3333333333333333703, 0.3170188387650512141, 0.3333333333333333703, 0.3170188387650512141, 0.3333333333333333703, 0.3170188387650512141, 0.3333333333333333703, 0.3170188387650512141, 0.3333333333333333703, 0.3170188387650512141, 0.3333333333333333703, 0.3170188387650512141, 0.3333333333333333703, 0.3170188387650512141, 0.3333333333333333703, 0.3170188387650512141, 0.3333333333333333703, 0.3170188387650512141, 0.3333333333333333703, 0.3170188387650512141, 0.3333333333333333703, 0.3170188387650512141, 0.3333333333333333703, 0.3170188387650512141, 0.3333333333333333703, 0.3170188387650512141, 0.3333333333333333703, 0.3170188387650512141, 0.3333333333333333703, 0.3170188387650512141, 0.3333333333333333703, 0.3170188387650512141, 0.3333333333333333703, 0.3170188387650512141, 0.3333333333333333703, 0.3170188387650512141, 0.3333333333333333703, 0.3170188387650512141, 0.3333333333333333703, 0.3170188387650512141, 0.3333333333333333703, 0.3170188387650512141, 0.3333333333333333703, 0.3170188387650512141, 0.3333333333333333703, 0.3170188387650512141, 0.3333333333333333703, 0.3170188387650512141, 0.3333333333333333703, 0.3170188387650512141, 0.3333333333333333703, 0.3170188387650512141, 0.3333333333333333703, 0.3170188387650512141, 0.3333333333333333703, 0.3170188387650512141, 0.3333333333333333703, 0.3170188387650512141, 0.3333333333333333703, 0.3170188387650512141, 0.3333333333333333703, 0.3170188387650512141, 0.3333333333333333703, 0.3170188387650512141, 0.3333333333333333703, 0.3170188387650512141, 0.3333333333333333703, 0.3170188387650512141, 0.3333333333333333703, 0.3170188387650512141, 0.3333333333333333703, 0.3170188387650512141, 0.3333333333333333703, 0.3170188387650512141, 0.3333333333333333703, 0.3170188387650512141, 0.3333333333333333703, 0.3170188387650512141, 0.3333333333333333703, 0.3170188387650512141, 0.3333333333333333703, 0.3170188387650512141, 0.3333333333333333703, 0.3170188387650512141, 0.3333333333333333703, 0.3170188387650512141, 0.3333333333333333703),
 ( 0.3333333333333333703, 0.3170188387650512141, 0.3333333333333333703, 0.3170188387650512141, 0.3333333333333333703, 0.3170188387650512141, 0.3333333333333333703, 0.3170188387650512141, 0.3333333333333333703, 0.3170188387650512141, 0.3333333333333333703, 0.3170188387650512141, 0.3333333333333333703, 0.3170188387650512141, 0.3333333333333333703, 0.3170188387650512141, 0.3333333333333333703, 0.3170188387650512141, 0.3333333333333333703, 0.3170188387650512141, 0.3333333333333333703, 0.3170188387650512141, 0.3333333333333333703, 0.3170188387650512141, 0.3333333333333333703, 0.3170188387650512141, 0.3333333333333333703, 0.3170188387650512141, 0.3333333333333333703, 0.3170188387650512141, 0.3333333333333333703, 0.3170188387650512141, 0.3333333333333333703, 0.3170188387650512141, 0.3333333333333333703, 0.3170188387650512141, 0.3333333333333333703, 0.3170188387650512141, 0.3333333333333333703, 0.3170188387650512141, 0.3333333333333333703, 0.3170188387650512141, 0.3333333333333333703, 0.3170188387650512141, 0.3333333333333333703, 0.3170188387650512141, 0.3333333333333333703, 0.3170188387650512141, 0.3333333333333333703, 0.3170188387650512141, 0.3333333333333333703, 0.3170188387650512141, 0.3333333333333333703, 0.3170188387650512141, 0.3333333333333333703, 0.3170188387650512141, 0.3333333333333333703, 0.3170188387650512141, 0.3333333333333333703, 0.3170188387650512141, 0.3333333333333333703, 0.3170188387650512141, 0.3333333333333333703, 0.3170188387650512141, 0.3333333333333333703, 0.3170188387650512141, 0.3333333333333333703, 0.3170188387650512141, 0.3333333333333333703, 0.3170188387650512141, 0.3333333333333333703, 0.3170188387650512141, 0.3333333333333333703, 0.3170188387650512141, 0.3333333333333333703, 0.3170188387650512141, 0.3333333333333333703, 0.3170188387650512141, 0.3333333333333333703, 0.3170188387650512141, 0.3333333333333333703, 0.3170188387650512141, 0.3333333333333333703, 0.3170188387650512141, 0.3333333333333333703, 0.3170188387650512141, 0.3333333333333333703, 0.3170188387650512141, 0.3333333333333333703, 0.3170188387650512141, 0.3333333333333333703, 0.3170188387650512141, 0.3333333333333333703, 0.3170188387650512141, 0.3333333333333333703, 0.3170188387650512141, 0.3333333333333333703, 0.3170188387650512141, 0.3333333333333333703, 0.3170188387650512141, 0.3333333333333333703, 0.3170188387650512141, 0.3333333333333333703, 0.3170188387650512141, 0.3333333333333333703, 0.3170188387650512141, 0.3333333333333333703, 0.3170188387650512141, 0.3333333333333333703, 0.3170188387650512141, 0.3333333333333333703, 0.3170188387650512141, 0.3333333333333333703, 0.3170188387650512141, 0.3333333333333333703, 0.3170188387650512141, 0.3333333333333333703, 0.3170188387650512141, 0.3333333333333333703, 0.3170188387650512141, 0.3333333333333333703, 0.3170188387650512141, 0.3333333333333333703, 0.3170188387650512141, 0.3333333333333333703, 0.3170188387650512141, 0.3333333333333333703, 0.3170188387650512141, 0.3333333333333333703, 0.3170188387650512141, 0.3333333333333333703, 0.3170188387650512141, 0.3333333333333333703, 0.3170188387650512141, 0.3333333333333333703, 0.3170188387650512141, 0.3333333333333333703, 0.3170188387650512141, 0.3333333333333333703, 0.3170188387650512141, 0.3333333333333333703, 0.3170188387650512141, 0.3333333333333333703, 0.3170188387650512141, 0.3333333333333333703, 0.3170188387650512141, 0.3333333333333333703, 0.3170188387650512141, 0.3333333333333333703, 0.3170188387650512141, 0.3333333333333333703, 0.3170188387650512141, 0.3333333333333333703, 0.3170188387650512141, 0.3333333333333333703, 0.3170188387650512141, 0.3333333333333333703, 0.3170188387650512141, 0.3333333333333333703, 0.3170188387650512141, 0.3333333333333333703, 0.3170188387650512141, 0.3333333333333333703, 0.3170188387650512141, 0.3333333333333333703, 0.3170188387650512141, 0.3333333333333333703, 0.3170188387650512141, 0.3333333333333333703, 0.3170188387650512141, 0.3333333333333333703, 0.3170188387650512141, 0.3333333333333333703, 0.3170188387650512141, 0.3333333333333333703, 0.3170188387650512141, 0.3333333333333333703, 0.3170188387650512141, 0.3333333333333333703, 0.3170188387650512141, 0.3333333333333333703, 0.3170188387650512141, 0.3333333333333333703, 0.3170188387650512141, 0.3333333333333333703, 0.3170188387650512141, 0.3333333333333333703, 0.3170188387650512141, 0.3333333333333333703, 0.3170188387650512141, 0.3333333333333333703, 0.3170188387650512141, 0.3333333333333333703, 0.3170188387650512141, 0.3333333333333333703, 0.3170188387650512141, 0.3333333333333333703, 0.3170188387650512141, 0.3333333333333333703, 0.3170188387650512141, 0.3333333333333333703, 0.3170188387650512141, 0.3333333333333333703, 0.3170188387650512141, 0.3333333333333333703, 0.3170188387650512141, 0.3333333333333333703, 0.3170188387650512141, 0.3333333333333333703, 0.3170188387650512141, 0.3333333333333333703, 0.3170188387650512141, 0.3333333333333333703, 0.3170188387650512141, 0.3333333333333333703, 0.3170188387650512141, 0.3333333333333333703, 0.3170188387650512141, 0.3333333333333333703, 0.3170188387650512141, 0.3333333333333333703, 0.3170188387650512141, 0.3333333333333333703, 0.3170188387650512141, 0.3333333333333333703, 0.3170188387650512141, 0.3333333333333333703, 0.3170188387650512141, 0.3333333333333333703, 0.3170188387650512141, 0.3333333333333333703, 0.3170188387650512141, 0.3333333333333333703, 0.3170188387650512141, 0.3333333333333333703, 0.3170188387650512141, 0.3333333333333333703, 0.3170188387650512141, 0.3333333333333333703, 0.3170188387650512141, 0.3333333333333333703, 0.3170188387650512141, 0.3333333333333333703, 0.3170188387650512141, 0.3333333333333333703, 0.3170188387650512141, 0.3333333333333333703, 0.3170188387650512141, 0.3333333333333333703, 0.3170188387650512141, 0.3333333333333333703, 0.3170188387650512141, 0.3333333333333333703, 0.3170188387650512141, 0.3333333333333333703, 0.3170188387650512141, 0.3333333333333333703, 0.3170188387650512141, 0.3333333333333333703, 0.3170188387650512141, 0.3333333333333333703),
 ( 1.000000000000000000, 0.9510565162951535312, 1.000000000000000000, 0.9510565162951535312, 1.000000000000000000, 0.9510565162951535312, 1.000000000000000000, 0.9510565162951535312, 1.000000000000000000, 0.9510565162951535312, 1.000000000000000000, 0.9510565162951535312, 1.000000000000000000, 0.9510565162951535312, 1.000000000000000000, 0.9510565162951535312, 1.000000000000000000, 0.9510565162951535312, 1.000000000000000000, 0.9510565162951535312, 1.000000000000000000, 0.9510565162951535312, 1.000000000000000000, 0.9510565162951535312, 1.000000000000000000, 0.9510565162951535312, 1.000000000000000000, 0.9510565162951535312, 1.000000000000000000, 0.9510565162951535312, 1.000000000000000000, 0.9510565162951535312, 1.000000000000000000, 0.9510565162951535312, 1.000000000000000000, 0.9510565162951535312, 1.000000000000000000, 0.9510565162951535312, 1.000000000000000000, 0.9510565162951535312, 1.000000000000000000, 0.9510565162951535312, 1.000000000000000000, 0.9510565162951535312, 1.000000000000000000, 0.9510565162951535312, 1.000000000000000000, 0.9510565162951535312, 1.000000000000000000, 0.9510565162951535312, 1.000000000000000000, 0.9510565162951535312, 1.000000000000000000, 0.9510565162951535312, 1.000000000000000000, 0.9510565162951535312, 1.000000000000000000, 0.9510565162951535312, 1.000000000000000000, 0.9510565162951535312, 1.000000000000000000, 0.9510565162951535312, 1.000000000000000000, 0.9510565162951535312, 1.000000000000000000, 0.9510565162951535312, 1.000000000000000000, 0.9510565162951535312, 1.000000000000000000, 0.9510565162951535312, 1.000000000000000000, 0.9510565162951535312, 1.000000000000000000, 0.9510565162951535312, 1.000000000000000000, 0.9510565162951535312, 1.000000000000000000, 0.9510565162951535312, 1.000000000000000000, 0.9510565162951535312, 1.000000000000000000, 0.9510565162951535312, 1.000000000000000000, 0.9510565162951535312, 1.000000000000000000, 0.9510565162951535312, 1.000000000000000000, 0.9510565162951535312, 1.000000000000000000, 0.9510565162951535312, 1.000000000000000000, 0.9510565162951535312, 1.000000000000000000, 0.9510565162951535312, 1.000000000000000000, 0.9510565162951535312, 1.000000000000000000, 0.9510565162951535312, 1.000000000000000000, 0.9510565162951535312, 1.000000000000000000, 0.9510565162951535312, 1.000000000000000000, 0.9510565162951535312, 1.000000000000000000, 0.9510565162951535312, 1.000000000000000000, 0.9510565162951535312, 1.000000000000000000, 0.9510565162951535312, 1.000000000000000000, 0.9510565162951535312, 1.000000000000000000, 0.9510565162951535312, 1.000000000000000000, 0.9510565162951535312, 1.000000000000000000, 0.9510565162951535312, 1.000000000000000000, 0.9510565162951535312, 1.000000000000000000, 0.9510565162951535312, 1.000000000000000000, 0.9510565162951535312, 1.000000000000000000, 0.9510565162951535312, 1.000000000000000000, 0.9510565162951535312, 1.000000000000000000, 0.9510565162951535312, 1.000000000000000000, 0.9510565162951535312, 1.000000000000000000, 0.9510565162951535312, 1.000000000000000000, 0.9510565162951535312, 1.000000000000000000, 0.9510565162951535312, 1.000000000000000000, 0.9510565162951535312, 1.000000000000000000, 0.9510565162951535312, 1.000000000000000000, 0.9510565162951535312, 1.000000000000000000, 0.9510565162951535312, 1.000000000000000000, 0.9510565162951535312, 1.000000000000000000, 0.9510565162951535312, 1.000000000000000000, 0.9510565162951535312, 1.000000000000000000, 0.9510565162951535312, 1.000000000000000000, 0.9510565162951535312, 1.000000000000000000, 0.9510565162951535312, 1.000000000000000000, 0.9510565162951535312, 1.000000000000000000, 0.9510565162951535312, 1.000000000000000000, 0.9510565162951535312, 1.000000000000000000, 0.9510565162951535312, 1.000000000000000000, 0.9510565162951535312, 1.000000000000000000, 0.9510565162951535312, 1.000000000000000000, 0.9510565162951535312, 1.000000000000000000, 0.9510565162951535312, 1.000000000000000000, 0.9510565162951535312, 1.000000000000000000, 0.9510565162951535312, 1.000000000000000000, 0.9510565162951535312, 1.000000000000000000, 0.9510565162951535312, 1.000000000000000000, 0.9510565162951535312, 1.000000000000000000, 0.9510565162951535312, 1.000000000000000000, 0.9510565162951535312, 1.000000000000000000, 0.9510565162951535312, 1.000000000000000000, 0.9510565162951535312, 1.000000000000000000, 0.9510565162951535312, 1.000000000000000000, 0.9510565162951535312, 1.000000000000000000, 0.9510565162951535312, 1.000000000000000000, 0.9510565162951535312, 1.000000000000000000, 0.9510565162951535312, 1.000000000000000000, 0.9510565162951535312, 1.000000000000000000, 0.9510565162951535312, 1.000000000000000000, 0.9510565162951535312, 1.000000000000000000, 0.9510565162951535312, 1.000000000000000000, 0.9510565162951535312, 1.000000000000000000, 0.9510565162951535312, 1.000000000000000000, 0.9510565162951535312, 1.000000000000000000, 0.9510565162951535312, 1.000000000000000000, 0.9510565162951535312, 1.000000000000000000, 0.9510565162951535312, 1.000000000000000000, 0.9510565162951535312, 1.000000000000000000, 0.9510565162951535312, 1.000000000000000000, 0.9510565162951535312, 1.000000000000000000, 0.9510565162951535312, 1.000000000000000000, 0.9510565162951535312, 1.000000000000000000, 0.9510565162951535312, 1.000000000000000000, 0.9510565162951535312, 1.000000000000000000, 0.9510565162951535312, 1.000000000000000000, 0.9510565162951535312, 1.000000000000000000, 0.9510565162951535312, 1.000000000000000000, 0.9510565162951535312, 1.000000000000000000, 0.9510565162951535312, 1.000000000000000000, 0.9510565162951535312, 1.000000000000000000, 0.9510565162951535312, 1.000000000000000000, 0.9510565162951535312, 1.000000000000000000, 0.9510565162951535312, 1.000000000000000000, 0.9510565162951535312, 1.000000000000000000, 0.9510565162951535312, 1.000000000000000000, 0.9510565162951535312, 1.000000000000000000),
 ( 0.3333333333333333703, 0.3170188387650512141, 0.3333333333333333703, 0.3170188387650512141, 0.3333333333333333703, 0.3170188387650512141, 0.3333333333333333703, 0.3170188387650512141, 0.3333333333333333703, 0.3170188387650512141, 0.3333333333333333703, 0.3170188387650512141, 0.3333333333333333703, 0.3170188387650512141, 0.3333333333333333703, 0.3170188387650512141, 0.3333333333333333703, 0.3170188387650512141, 0.3333333333333333703, 0.3170188387650512141, 0.3333333333333333703, 0.3170188387650512141, 0.3333333333333333703, 0.3170188387650512141, 0.3333333333333333703, 0.3170188387650512141, 0.3333333333333333703, 0.3170188387650512141, 0.3333333333333333703, 0.3170188387650512141, 0.3333333333333333703, 0.3170188387650512141, 0.3333333333333333703, 0.3170188387650512141, 0.3333333333333333703, 0.3170188387650512141, 0.3333333333333333703, 0.3170188387650512141, 0.3333333333333333703, 0.3170188387650512141, 0.3333333333333333703, 0.3170188387650512141, 0.3333333333333333703, 0.3170188387650512141, 0.3333333333333333703, 0.3170188387650512141, 0.3333333333333333703, 0.3170188387650512141, 0.3333333333333333703, 0.3170188387650512141, 0.3333333333333333703, 0.3170188387650512141, 0.3333333333333333703, 0.3170188387650512141, 0.3333333333333333703, 0.3170188387650512141, 0.3333333333333333703, 0.3170188387650512141, 0.3333333333333333703, 0.3170188387650512141, 0.3333333333333333703, 0.3170188387650512141, 0.3333333333333333703, 0.3170188387650512141, 0.3333333333333333703, 0.3170188387650512141, 0.3333333333333333703, 0.3170188387650512141, 0.3333333333333333703, 0.3170188387650512141, 0.3333333333333333703, 0.3170188387650512141, 0.3333333333333333703, 0.3170188387650512141, 0.3333333333333333703, 0.3170188387650512141, 0.3333333333333333703, 0.3170188387650512141, 0.3333333333333333703, 0.3170188387650512141, 0.3333333333333333703, 0.3170188387650512141, 0.3333333333333333703, 0.3170188387650512141, 0.3333333333333333703, 0.3170188387650512141, 0.3333333333333333703, 0.3170188387650512141, 0.3333333333333333703, 0.3170188387650512141, 0.3333333333333333703, 0.3170188387650512141, 0.3333333333333333703, 0.3170188387650512141, 0.3333333333333333703, 0.3170188387650512141, 0.3333333333333333703, 0.3170188387650512141, 0.3333333333333333703, 0.3170188387650512141, 0.3333333333333333703, 0.3170188387650512141, 0.3333333333333333703, 0.3170188387650512141, 0.3333333333333333703, 0.3170188387650512141, 0.3333333333333333703, 0.3170188387650512141, 0.3333333333333333703, 0.3170188387650512141, 0.3333333333333333703, 0.3170188387650512141, 0.3333333333333333703, 0.3170188387650512141, 0.3333333333333333703, 0.3170188387650512141, 0.3333333333333333703, 0.3170188387650512141, 0.3333333333333333703, 0.3170188387650512141, 0.3333333333333333703, 0.3170188387650512141, 0.3333333333333333703, 0.3170188387650512141, 0.3333333333333333703, 0.3170188387650512141, 0.3333333333333333703, 0.3170188387650512141, 0.3333333333333333703, 0.3170188387650512141, 0.3333333333333333703, 0.3170188387650512141, 0.3333333333333333703, 0.3170188387650512141, 0.3333333333333333703, 0.3170188387650512141, 0.3333333333333333703, 0.3170188387650512141, 0.3333333333333333703, 0.3170188387650512141, 0.3333333333333333703, 0.3170188387650512141, 0.3333333333333333703, 0.3170188387650512141, 0.3333333333333333703, 0.3170188387650512141, 0.3333333333333333703, 0.3170188387650512141, 0.3333333333333333703, 0.3170188387650512141, 0.3333333333333333703, 0.3170188387650512141, 0.3333333333333333703, 0.3170188387650512141, 0.3333333333333333703, 0.3170188387650512141, 0.3333333333333333703, 0.3170188387650512141, 0.3333333333333333703, 0.3170188387650512141, 0.3333333333333333703, 0.3170188387650512141, 0.3333333333333333703, 0.3170188387650512141, 0.3333333333333333703, 0.3170188387650512141, 0.3333333333333333703, 0.3170188387650512141, 0.3333333333333333703, 0.3170188387650512141, 0.3333333333333333703, 0.3170188387650512141, 0.3333333333333333703, 0.3170188387650512141, 0.3333333333333333703, 0.3170188387650512141, 0.3333333333333333703, 0.3170188387650512141, 0.3333333333333333703, 0.3170188387650512141, 0.3333333333333333703, 0.3170188387650512141, 0.3333333333333333703, 0.3170188387650512141, 0.3333333333333333703, 0.3170188387650512141, 0.3333333333333333703, 0.3170188387650512141, 0.3333333333333333703, 0.3170188387650512141, 0.3333333333333333703, 0.3170188387650512141, 0.3333333333333333703, 0.3170188387650512141, 0.3333333333333333703, 0.3170188387650512141, 0.3333333333333333703, 0.3170188387650512141, 0.3333333333333333703, 0.3170188387650512141, 0.3333333333333333703, 0.3170188387650512141, 0.3333333333333333703, 0.3170188387650512141, 0.3333333333333333703, 0.3170188387650512141, 0.3333333333333333703, 0.3170188387650512141, 0.3333333333333333703, 0.3170188387650512141, 0.3333333333333333703, 0.3170188387650512141, 0.3333333333333333703, 0.3170188387650512141, 0.3333333333333333703, 0.3170188387650512141, 0.3333333333333333703, 0.3170188387650512141, 0.3333333333333333703, 0.3170188387650512141, 0.3333333333333333703, 0.3170188387650512141, 0.3333333333333333703, 0.3170188387650512141, 0.3333333333333333703, 0.3170188387650512141, 0.3333333333333333703, 0.3170188387650512141, 0.3333333333333333703, 0.3170188387650512141, 0.3333333333333333703, 0.3170188387650512141, 0.3333333333333333703, 0.3170188387650512141, 0.3333333333333333703, 0.3170188387650512141, 0.3333333333333333703, 0.3170188387650512141, 0.3333333333333333703, 0.3170188387650512141, 0.3333333333333333703, 0.3170188387650512141, 0.3333333333333333703, 0.3170188387650512141, 0.3333333333333333703, 0.3170188387650512141, 0.3333333333333333703, 0.3170188387650512141, 0.3333333333333333703, 0.3170188387650512141, 0.3333333333333333703, 0.3170188387650512141, 0.3333333333333333703, 0.3170188387650512141, 0.3333333333333333703, 0.3170188387650512141, 0.3333333333333333703, 0.3170188387650512141, 0.3333333333333333703, 0.3170188387650512141, 0.3333333333333333703),
 ( 0.3333333333333333703, 0.3170188387650512141, 0.3333333333333333703, 0.3170188387650512141, 0.3333333333333333703, 0.3170188387650512141, 0.3333333333333333703, 0.3170188387650512141, 0.3333333333333333703, 0.3170188387650512141, 0.3333333333333333703, 0.3170188387650512141, 0.3333333333333333703, 0.3170188387650512141, 0.3333333333333333703, 0.3170188387650512141, 0.3333333333333333703, 0.3170188387650512141, 0.3333333333333333703, 0.3170188387650512141, 0.3333333333333333703, 0.3170188387650512141, 0.3333333333333333703, 0.3170188387650512141, 0.3333333333333333703, 0.3170188387650512141, 0.3333333333333333703, 0.3170188387650512141, 0.3333333333333333703, 0.3170188387650512141, 0.3333333333333333703, 0.3170188387650512141, 0.3333333333333333703, 0.3170188387650512141, 0.3333333333333333703, 0.3170188387650512141, 0.3333333333333333703, 0.3170188387650512141, 0.3333333333333333703, 0.3170188387650512141, 0.3333333333333333703, 0.3170188387650512141, 0.3333333333333333703, 0.3170188387650512141, 0.3333333333333333703, 0.3170188387650512141, 0.3333333333333333703, 0.3170188387650512141, 0.3333333333333333703, 0.3170188387650512141, 0.3333333333333333703, 0.3170188387650512141, 0.3333333333333333703, 0.3170188387650512141, 0.3333333333333333703, 0.3170188387650512141, 0.3333333333333333703, 0.3170188387650512141, 0.3333333333333333703, 0.3170188387650512141, 0.3333333333333333703, 0.3170188387650512141, 0.3333333333333333703, 0.3170188387650512141, 0.3333333333333333703, 0.3170188387650512141, 0.3333333333333333703, 0.3170188387650512141, 0.3333333333333333703, 0.3170188387650512141, 0.3333333333333333703, 0.3170188387650512141, 0.3333333333333333703, 0.3170188387650512141, 0.3333333333333333703, 0.3170188387650512141, 0.3333333333333333703, 0.3170188387650512141, 0.3333333333333333703, 0.3170188387650512141, 0.3333333333333333703, 0.3170188387650512141, 0.3333333333333333703, 0.3170188387650512141, 0.3333333333333333703, 0.3170188387650512141, 0.3333333333333333703, 0.3170188387650512141, 0.3333333333333333703, 0.3170188387650512141, 0.3333333333333333703, 0.3170188387650512141, 0.3333333333333333703, 0.3170188387650512141, 0.3333333333333333703, 0.3170188387650512141, 0.3333333333333333703, 0.3170188387650512141, 0.3333333333333333703, 0.3170188387650512141, 0.3333333333333333703, 0.3170188387650512141, 0.3333333333333333703, 0.3170188387650512141, 0.3333333333333333703, 0.3170188387650512141, 0.3333333333333333703, 0.3170188387650512141, 0.3333333333333333703, 0.3170188387650512141, 0.3333333333333333703, 0.3170188387650512141, 0.3333333333333333703, 0.3170188387650512141, 0.3333333333333333703, 0.3170188387650512141, 0.3333333333333333703, 0.3170188387650512141, 0.3333333333333333703, 0.3170188387650512141, 0.3333333333333333703, 0.3170188387650512141, 0.3333333333333333703, 0.3170188387650512141, 0.3333333333333333703, 0.3170188387650512141, 0.3333333333333333703, 0.3170188387650512141, 0.3333333333333333703, 0.3170188387650512141, 0.3333333333333333703, 0.3170188387650512141, 0.3333333333333333703, 0.3170188387650512141, 0.3333333333333333703, 0.3170188387650512141, 0.3333333333333333703, 0.3170188387650512141, 0.3333333333333333703, 0.3170188387650512141, 0.3333333333333333703, 0.3170188387650512141, 0.3333333333333333703, 0.3170188387650512141, 0.3333333333333333703, 0.3170188387650512141, 0.3333333333333333703, 0.3170188387650512141, 0.3333333333333333703, 0.3170188387650512141, 0.3333333333333333703, 0.3170188387650512141, 0.3333333333333333703, 0.3170188387650512141, 0.3333333333333333703, 0.3170188387650512141, 0.3333333333333333703, 0.3170188387650512141, 0.3333333333333333703, 0.3170188387650512141, 0.3333333333333333703, 0.3170188387650512141, 0.3333333333333333703, 0.3170188387650512141, 0.3333333333333333703, 0.3170188387650512141, 0.3333333333333333703, 0.3170188387650512141, 0.3333333333333333703, 0.3170188387650512141, 0.3333333333333333703, 0.3170188387650512141, 0.3333333333333333703, 0.3170188387650512141, 0.3333333333333333703, 0.3170188387650512141, 0.3333333333333333703, 0.3170188387650512141, 0.3333333333333333703, 0.3170188387650512141, 0.3333333333333333703, 0.3170188387650512141, 0.3333333333333333703, 0.3170188387650512141, 0.3333333333333333703, 0.3170188387650512141, 0.3333333333333333703, 0.3170188387650512141, 0.3333333333333333703, 0.3170188387650512141, 0.3333333333333333703, 0.3170188387650512141, 0.3333333333333333703, 0.3170188387650512141, 0.3333333333333333703, 0.3170188387650512141, 0.3333333333333333703, 0.3170188387650512141, 0.3333333333333333703, 0.3170188387650512141, 0.3333333333333333703, 0.3170188387650512141, 0.3333333333333333703, 0.3170188387650512141, 0.3333333333333333703, 0.3170188387650512141, 0.3333333333333333703, 0.3170188387650512141, 0.3333333333333333703, 0.3170188387650512141, 0.3333333333333333703, 0.3170188387650512141, 0.3333333333333333703, 0.3170188387650512141, 0.3333333333333333703, 0.3170188387650512141, 0.3333333333333333703, 0.3170188387650512141, 0.3333333333333333703, 0.3170188387650512141, 0.3333333333333333703, 0.3170188387650512141, 0.3333333333333333703, 0.3170188387650512141, 0.3333333333333333703, 0.3170188387650512141, 0.3333333333333333703, 0.3170188387650512141, 0.3333333333333333703, 0.3170188387650512141, 0.3333333333333333703, 0.3170188387650512141, 0.3333333333333333703, 0.3170188387650512141, 0.3333333333333333703, 0.3170188387650512141, 0.3333333333333333703, 0.3170188387650512141, 0.3333333333333333703, 0.3170188387650512141, 0.3333333333333333703, 0.3170188387650512141, 0.3333333333333333703, 0.3170188387650512141, 0.3333333333333333703, 0.3170188387650512141, 0.3333333333333333703, 0.3170188387650512141, 0.3333333333333333703, 0.3170188387650512141, 0.3333333333333333703, 0.3170188387650512141, 0.3333333333333333703, 0.3170188387650512141, 0.3333333333333333703, 0.3170188387650512141, 0.3333333333333333703, 0.3170188387650512141, 0.3333333333333333703, 0.3170188387650512141, 0.3333333333333333703),
 ( 1.000000000000000000, 0.9510565162951535312, 1.000000000000000000, 0.9510565162951535312, 1.000000000000000000, 0.9510565162951535312, 1.000000000000000000, 0.9510565162951535312, 1.000000000000000000, 0.9510565162951535312, 1.000000000000000000, 0.9510565162951535312, 1.000000000000000000, 0.9510565162951535312, 1.000000000000000000, 0.9510565162951535312, 1.000000000000000000, 0.9510565162951535312, 1.000000000000000000, 0.9510565162951535312, 1.000000000000000000, 0.9510565162951535312, 1.000000000000000000, 0.9510565162951535312, 1.000000000000000000, 0.9510565162951535312, 1.000000000000000000, 0.9510565162951535312, 1.000000000000000000, 0.9510565162951535312, 1.000000000000000000, 0.9510565162951535312, 1.000000000000000000, 0.9510565162951535312, 1.000000000000000000, 0.9510565162951535312, 1.000000000000000000, 0.9510565162951535312, 1.000000000000000000, 0.9510565162951535312, 1.000000000000000000, 0.9510565162951535312, 1.000000000000000000, 0.9510565162951535312, 1.000000000000000000, 0.9510565162951535312, 1.000000000000000000, 0.9510565162951535312, 1.000000000000000000, 0.9510565162951535312, 1.000000000000000000, 0.9510565162951535312, 1.000000000000000000, 0.9510565162951535312, 1.000000000000000000, 0.9510565162951535312, 1.000000000000000000, 0.9510565162951535312, 1.000000000000000000, 0.9510565162951535312, 1.000000000000000000, 0.9510565162951535312, 1.000000000000000000, 0.9510565162951535312, 1.000000000000000000, 0.9510565162951535312, 1.000000000000000000, 0.9510565162951535312, 1.000000000000000000, 0.9510565162951535312, 1.000000000000000000, 0.9510565162951535312, 1.000000000000000000, 0.9510565162951535312, 1.000000000000000000, 0.9510565162951535312, 1.000000000000000000, 0.9510565162951535312, 1.000000000000000000, 0.9510565162951535312, 1.000000000000000000, 0.9510565162951535312, 1.000000000000000000, 0.9510565162951535312, 1.000000000000000000, 0.9510565162951535312, 1.000000000000000000, 0.9510565162951535312, 1.000000000000000000, 0.9510565162951535312, 1.000000000000000000, 0.9510565162951535312, 1.000000000000000000, 0.9510565162951535312, 1.000000000000000000, 0.9510565162951535312, 1.000000000000000000, 0.9510565162951535312, 1.000000000000000000, 0.9510565162951535312, 1.000000000000000000, 0.9510565162951535312, 1.000000000000000000, 0.9510565162951535312, 1.000000000000000000, 0.9510565162951535312, 1.000000000000000000, 0.9510565162951535312, 1.000000000000000000, 0.9510565162951535312, 1.000000000000000000, 0.9510565162951535312, 1.000000000000000000, 0.9510565162951535312, 1.000000000000000000, 0.9510565162951535312, 1.000000000000000000, 0.9510565162951535312, 1.000000000000000000, 0.9510565162951535312, 1.000000000000000000, 0.9510565162951535312, 1.000000000000000000, 0.9510565162951535312, 1.000000000000000000, 0.9510565162951535312, 1.000000000000000000, 0.9510565162951535312, 1.000000000000000000, 0.9510565162951535312, 1.000000000000000000, 0.9510565162951535312, 1.000000000000000000, 0.9510565162951535312, 1.000000000000000000, 0.9510565162951535312, 1.000000000000000000, 0.9510565162951535312, 1.000000000000000000, 0.9510565162951535312, 1.000000000000000000, 0.9510565162951535312, 1.000000000000000000, 0.9510565162951535312, 1.000000000000000000, 0.9510565162951535312, 1.000000000000000000, 0.9510565162951535312, 1.000000000000000000, 0.9510565162951535312, 1.000000000000000000, 0.9510565162951535312, 1.000000000000000000, 0.9510565162951535312, 1.000000000000000000, 0.9510565162951535312, 1.000000000000000000, 0.9510565162951535312, 1.000000000000000000, 0.9510565162951535312, 1.000000000000000000, 0.9510565162951535312, 1.000000000000000000, 0.9510565162951535312, 1.000000000000000000, 0.9510565162951535312, 1.000000000000000000, 0.9510565162951535312, 1.000000000000000000, 0.9510565162951535312, 1.000000000000000000, 0.9510565162951535312, 1.000000000000000000, 0.9510565162951535312, 1.000000000000000000, 0.9510565162951535312, 1.000000000000000000, 0.9510565162951535312, 1.000000000000000000, 0.9510565162951535312, 1.000000000000000000, 0.9510565162951535312, 1.000000000000000000, 0.9510565162951535312, 1.000000000000000000, 0.9510565162951535312, 1.000000000000000000, 0.9510565162951535312, 1.000000000000000000, 0.9510565162951535312, 1.000000000000000000, 0.9510565162951535312, 1.000000000000000000, 0.9510565162951535312, 1.000000000000000000, 0.9510565162951535312, 1.000000000000000000, 0.9510565162951535312, 1.000000000000000000, 0.9510565162951535312, 1.000000000000000000, 0.9510565162951535312, 1.000000000000000000, 0.9510565162951535312, 1.000000000000000000, 0.9510565162951535312, 1.000000000000000000, 0.9510565162951535312, 1.000000000000000000, 0.9510565162951535312, 1.000000000000000000, 0.9510565162951535312, 1.000000000000000000, 0.9510565162951535312, 1.000000000000000000, 0.9510565162951535312, 1.000000000000000000, 0.9510565162951535312, 1.000000000000000000, 0.9510565162951535312, 1.000000000000000000, 0.9510565162951535312, 1.000000000000000000, 0.9510565162951535312, 1.000000000000000000, 0.9510565162951535312, 1.000000000000000000, 0.9510565162951535312, 1.000000000000000000, 0.9510565162951535312, 1.000000000000000000, 0.9510565162951535312, 1.000000000000000000, 0.9510565162951535312, 1.000000000000000000, 0.9510565162951535312, 1.000000000000000000, 0.9510565162951535312, 1.000000000000000000, 0.9510565162951535312, 1.000000000000000000, 0.9510565162951535312, 1.000000000000000000, 0.9510565162951535312, 1.000000000000000000, 0.9510565162951535312, 1.000000000000000000, 0.9510565162951535312, 1.000000000000000000, 0.9510565162951535312, 1.000000000000000000, 0.9510565162951535312, 1.000000000000000000, 0.9510565162951535312, 1.000000000000000000, 0.9510565162951535312, 1.000000000000000000, 0.9510565162951535312, 1.000000000000000000, 0.9510565162951535312, 1.000000000000000000) ) ) 
 REPRESENTATION_ITEM ( '' )  SURFACE ( )  );
#5962=CARTESIAN_POINT ( 'NONE',  ( -5.257311121191324155, -74.74547149457075079, -0.09995255151718371311 ) ) ;
#5965=CARTESIAN_POINT ( 'NONE',  ( 2.862020680886601998, -96.79547149457073374, 4.100960146803977580 ) ) ;
#5966=CARTESIAN_POINT ( 'NONE',  ( 6.013306294175168709, -67.95452850542925205, 4.245374608440616093 ) ) ;
#5971=CARTESIAN_POINT ( 'NONE',  ( 4.312004677471078296, -85.95452850542925205, 3.009306630940844496 ) ) ;
#5972=CARTESIAN_POINT ( 'NONE',  ( -2.179377348189463159, -64.35452850542924352, 7.030887037049988741 ) ) ;
#5973=CARTESIAN_POINT ( 'NONE',  ( 2.493201789345310004, -78.94547149457073942, 1.934965279058241006 ) ) ;
#5975=STYLED_ITEM ( 'NONE', ( #1149 ), #7136 ) ;
#5978=CARTESIAN_POINT ( 'NONE',  ( -2.862020680886492308, -94.20452850542926626, 4.100960146804039752 ) ) ;
#5979=CARTESIAN_POINT ( 'NONE',  ( 5.257311121191342806, -89.25452850542924921, -0.09995255151729465215 ) ) ;
#5981=CARTESIAN_POINT ( 'NONE',  ( 4.784657899331209663, -74.10452850542925773, 1.454677039711774533 ) ) ;
#5982=CARTESIAN_POINT ( 'NONE',  ( -0.8796985632579406023, -95.14547149457074227, -3.030887037049952326 ) ) ;
#5984=CARTESIAN_POINT ( 'NONE',  ( 2.862020680886514956, -83.70452850542925205, -4.100960146804039752 ) ) ;
#5985=CARTESIAN_POINT ( 'NONE',  ( 4.191402346623199549, -94.80452850542926058, 5.607243785695311900 ) ) ;
#5986=CARTESIAN_POINT ( 'NONE',  ( -0.09506052544082083111, -63.00452850542925631, -2.999999999999997780 ) ) ;
#5990=CARTESIAN_POINT ( 'NONE',  ( -0.8796985632578785408, -82.35452850542927195, 3.030887037049973198 ) ) ;
#5991=CARTESIAN_POINT ( 'NONE',  ( 6.686770931921525829, -92.10452850542925773, 2.072711028461649008 ) ) ;
#5992=CARTESIAN_POINT ( 'NONE',  ( -7.360235569667856304, -92.74547149457073658, -0.09995255151716124498 ) ) ;
#5996=CARTESIAN_POINT ( 'NONE',  ( -0.09506052544075706268, -72.49547149457075079, 2.999999999999997780 ) ) ;
#5998=CARTESIAN_POINT ( 'NONE',  ( -2.862020680886495416, -67.20452850542925205, 4.100960146804039752 ) ) ;
#5999=CARTESIAN_POINT ( 'NONE',  ( 6.686770931921477867, -79.39547149457074227, -2.072711028461788896 ) ) ;
#6002=CARTESIAN_POINT ( 'NONE',  ( -1.529537955723671683, -64.35452850542924352, 5.030887037049979860 ) ) ;
#6005=CARTESIAN_POINT ( 'NONE',  ( 4.784657899331176800, -73.39547149457074227, -1.454677039711874009 ) ) ;
#6007=CARTESIAN_POINT ( 'NONE',  ( -1.069819614139476460, -60.34547149457074511, 2.969112962950044121 ) ) ;
#6008=CARTESIAN_POINT ( 'NONE',  ( -6.628020296210623385, -63.90452850542925489, 2.253526892787613978 ) ) ;
#6011=CARTESIAN_POINT ( 'NONE',  ( 4.784657899331210551, -83.10452850542927195, 1.454677039711774533 ) ) ;
#6012=CARTESIAN_POINT ( 'NONE',  ( 4.037591185471440802, -62.70452850542925916, -5.718994135553947977 ) ) ;
#6013=CARTESIAN_POINT ( 'NONE',  ( 0.8796985632579624736, -81.64547149457074227, 3.030887037049952326 ) ) ;
#6017=CARTESIAN_POINT ( 'NONE',  ( -5.257311121191324155, -78.75452850542924921, 0.09995255151729526277 ) ) ;
#6019=CARTESIAN_POINT ( 'NONE',  ( -1.529537955723670795, -73.35452850542924352, 5.030887037049979860 ) ) ;
#6020=CARTESIAN_POINT ( 'NONE',  ( -1.686450176301615977, -86.29547149457074795, -2.482926158054096000 ) ) ;
#6021=CARTESIAN_POINT ( 'NONE',  ( -1.686450176301618864, -62.29547149457074084, -2.482926158054096000 ) ) ;
#6022=CARTESIAN_POINT ( 'NONE',  ( 4.784657899331209663, -74.10452850542925773, 1.454677039711774533 ) ) ;
#6023=CARTESIAN_POINT ( 'NONE',  ( -6.628020296210619833, -87.90452850542926910, 2.253526892787613978 ) ) ;
#6024=CARTESIAN_POINT ( 'NONE',  ( -1.069819614139539521, -69.15452850542926910, -2.969112962950023249 ) ) ;
#6029=CARTESIAN_POINT ( 'NONE',  ( -1.069819614139537967, -78.15452850542924068, -2.969112962950023249 ) ) ;
#6030=CARTESIAN_POINT ( 'NONE',  ( -2.369498399071205963, -87.15452850542926910, -6.969112962950009482 ) ) ;
#6032=CARTESIAN_POINT ( 'NONE',  ( -6.628020296210665130, -89.59547149457074511, -2.253526892787471869 ) ) ;
#6035=CARTESIAN_POINT ( 'NONE',  ( 2.823794231030058555, -67.09547149457073090, 1.017458915287723809 ) ) ;
#6039=CARTESIAN_POINT ( 'NONE',  ( -5.257311121191324155, -66.75452850542923500, 0.09995255151729526277 ) ) ;
#6040=CARTESIAN_POINT ( 'NONE',  ( -4.191402346623058328, -78.19547149457073942, 5.607243785695398941 ) ) ;
#6042=CARTESIAN_POINT ( 'NONE',  ( -5.257311121191325043, -71.74547149457075079, -0.09995255151718372699 ) ) ;
#6043=CARTESIAN_POINT ( 'NONE',  ( 4.784657899331208775, -65.10452850542924352, 1.454677039711774533 ) ) ;
#6048=CARTESIAN_POINT ( 'NONE',  ( 1.529537955723794695, -66.64547149457071384, 5.030887037049945221 ) ) ;
#6050=CARTESIAN_POINT ( 'NONE',  ( -4.312004677470990366, -96.04547149457074795, 3.009306630940933758 ) ) ;
#6051=CARTESIAN_POINT ( 'NONE',  ( -2.179377348189463603, -61.35452850542925773, 7.030887037049988741 ) ) ;
#6054=CARTESIAN_POINT ( 'NONE',  ( 4.725907263620340970, -80.40452850542925489, -1.635492904037697981 ) ) ;
#6058=CARTESIAN_POINT ( 'NONE',  ( 4.194503406049339134, -89.55452850542926058, -3.171033256558100089 ) ) ;
#6059=CARTESIAN_POINT ( 'NONE',  ( 4.312004677471076519, -82.95452850542925205, 3.009306630940844496 ) ) ;
#6062=CARTESIAN_POINT ( 'NONE',  ( -5.257311121191325043, -69.75452850542926342, 0.09995255151729529053 ) ) ;
#6063=CARTESIAN_POINT ( 'NONE',  ( 2.882544866740879730, -94.39547149457074227, -0.8366430509619593447 ) ) ;
#6064=CARTESIAN_POINT ( 'NONE',  ( -2.610703060766927930, -60.04547149457073374, 1.773238653441125745 ) ) ;
#6065=CARTESIAN_POINT ( 'NONE',  ( -3.015831842038214639, -78.30452850542926058, -3.989209796945429432 ) ) ;
#6066=CARTESIAN_POINT ( 'NONE',  ( 0.09506052544088250400, -85.50452850542926342, 6.999999999999997335 ) ) ;
#6067=CARTESIAN_POINT ( 'NONE',  ( -0.09506052544075405120, -96.49547149457075079, 2.999999999999997780 ) ) ;
#6072=CARTESIAN_POINT ( 'NONE',  ( 1.069819614139557062, -76.65452850542925489, 2.969112962950023249 ) ) ;
#6073=CARTESIAN_POINT ( 'NONE',  ( 0.09506052544088290646, -88.50452850542926342, 6.999999999999997335 ) ) ;
#6074=CARTESIAN_POINT ( 'NONE',  ( 2.179377348189630137, -81.64547149457074227, 7.030887037049939003 ) ) ;
#6076=CARTESIAN_POINT ( 'NONE',  ( -2.862020680886578461, -95.29547149457074795, -4.100960146803977580 ) ) ;
#6077=CARTESIAN_POINT ( 'NONE',  ( 1.686450176301586668, -86.70452850542925205, -2.482926158054133303 ) ) ;
#6081=CARTESIAN_POINT ( 'NONE',  ( -4.725907263620323207, -63.90452850542925489, 1.635492904037698647 ) ) ;
#6082=CARTESIAN_POINT ( 'NONE',  ( 6.686770931921479644, -82.39547149457074227, -2.072711028461788896 ) ) ;
#6084=CARTESIAN_POINT ( 'NONE',  ( -4.312004677470993030, -78.04547149457076216, 3.009306630940933314 ) ) ;
#6085=CARTESIAN_POINT ( 'NONE',  ( 4.784657899331176800, -67.39547149457074227, -1.454677039711874009 ) ) ;
#6086=CARTESIAN_POINT ( 'NONE',  ( 3.015831842038232846, -67.80452850542926058, 3.989209796945429432 ) ) ;
#6089=CARTESIAN_POINT ( 'NONE',  ( 4.312004677471011682, -70.54547149457074795, -3.009306630940933314 ) ) ;
#6090=CARTESIAN_POINT ( 'NONE',  ( -2.179377348189463603, -58.35452850542927195, 7.030887037049988741 ) ) ;
#6095=CARTESIAN_POINT ( 'NONE',  ( -1.719659006605370744, -90.15452850542922647, -4.969112962950016588 ) ) ;
#6096=CARTESIAN_POINT ( 'NONE',  ( -1.529537955723670350, -76.35452850542925773, 5.030887037049979860 ) ) ;
#6098=CARTESIAN_POINT ( 'NONE',  ( 3.015831842038232846, -67.80452850542926058, 3.989209796945429432 ) ) ;
#6099=CARTESIAN_POINT ( 'NONE',  ( -2.882544866740857081, -80.89547149457074227, 0.8366430509619596778 ) ) ;
#6100=CARTESIAN_POINT ( 'NONE',  ( -1.069819614139476460, -60.34547149457074511, 2.969112962950044121 ) ) ;
#6101=CARTESIAN_POINT ( 'NONE',  ( 0.09506052544085971667, -73.50452850542924921, 4.999999999999997335 ) ) ;
#6102=CARTESIAN_POINT ( 'NONE',  ( 6.013306294175171374, -85.95452850542925205, 4.245374608440616093 ) ) ;
#6105=CARTESIAN_POINT ( 'NONE',  ( 0.8796985632579640280, -93.64547149457074227, 3.030887037049952326 ) ) ;
#6109=CARTESIAN_POINT ( 'NONE',  ( 1.529537955723692999, -95.85452850542924352, -5.030887037049978971 ) ) ;
#6110=CARTESIAN_POINT ( 'NONE',  ( -1.686450176301566017, -73.20452850542925205, 2.482926158054133303 ) ) ;
#6111=CARTESIAN_POINT ( 'NONE',  ( -2.369498399071205963, -84.15452850542925489, -6.969112962950009482 ) ) ;
#6112=CARTESIAN_POINT ( 'NONE',  ( -6.686770931921458327, -80.89547149457074227, 2.072711028461789784 ) ) ;
#6114=CARTESIAN_POINT ( 'NONE',  ( -0.09506052544073315125, -93.49547149457073658, 4.999999999999997335 ) ) ;
#6115=CARTESIAN_POINT ( 'NONE',  ( 2.610703060766985217, -88.95452850542925205, 1.773238653441072232 ) ) ;
#6117=UNCERTAINTY_MEASURE_WITH_UNIT (LENGTH_MEASURE( 1.000000000000000082E-05 ), #1409, 'distance_accuracy_value', 'NONE');
#6121=CARTESIAN_POINT ( 'NONE',  ( -4.312004677471060532, -63.45452850542926626, -3.009306630940844052 ) ) ;
#6122=CARTESIAN_POINT ( 'NONE',  ( -5.895805022753476621, -83.44547149457073942, -4.407101234057782868 ) ) ;
#6124=CARTESIAN_POINT ( 'NONE',  ( -0.09506052544073503863, -78.49547149457073658, 4.999999999999997335 ) ) ;
#6125=CARTESIAN_POINT ( 'NONE',  ( 4.725907263620372056, -73.09547149457074511, 1.635492904037598283 ) ) ;
#6126=CARTESIAN_POINT ( 'NONE',  ( 1.719659006605388507, -61.65452850542923358, 4.969112962950016588 ) ) ;
#6129=CARTESIAN_POINT ( 'NONE',  ( 2.862020680886599333, -72.79547149457074795, 4.100960146803977580 ) ) ;
#6130=CARTESIAN_POINT ( 'NONE',  ( 4.037591185471440802, -62.70452850542925916, -5.718994135553947977 ) ) ;
#6137=CARTESIAN_POINT ( 'NONE',  ( 2.862020680886515400, -86.70452850542925205, -4.100960146804039752 ) ) ;
#6138=CARTESIAN_POINT ( 'NONE',  ( 0.09506052544086046607, -79.50452850542926342, 4.999999999999997335 ) ) ;
#6139=CARTESIAN_POINT ( 'NONE',  ( -1.719659006605372298, -75.15452850542925489, -4.969112962950015699 ) ) ;
#6140=CARTESIAN_POINT ( 'NONE',  ( -2.882544866740857081, -83.89547149457074227, 0.8366430509619596778 ) ) ;
#6141=CARTESIAN_POINT ( 'NONE',  ( -2.882544866740859746, -62.89547149457074227, 0.8366430509619596778 ) ) ;
#6142=CARTESIAN_POINT ( 'NONE',  ( -5.257311121191324155, -66.75452850542923500, 0.09995255151729526277 ) ) ;
#6143=CARTESIAN_POINT ( 'NONE',  ( -6.686770931921504513, -84.60452850542927195, -2.072711028461647675 ) ) ;
#6144=CARTESIAN_POINT ( 'NONE',  ( -2.823794231030023028, -60.90452850542925489, 1.017458915287783316 ) ) ;
#6151=CARTESIAN_POINT ( 'NONE',  ( 3.154386672714807549, -68.25452850542924921, -0.09995255151727241993 ) ) ;
#6152=CARTESIAN_POINT ( 'NONE',  ( -7.360235569667858968, -80.74547149457075079, -0.09995255151716124498 ) ) ;
#6156=CARTESIAN_POINT ( 'NONE',  ( 2.610703060766984329, -82.95452850542925205, 1.773238653441072232 ) ) ;
#6162=CARTESIAN_POINT ( 'NONE',  ( 1.069819614139559061, -94.65452850542924068, 2.969112962950023249 ) ) ;
#6163=CARTESIAN_POINT ( 'NONE',  ( 2.369498399071076733, -70.84547149457073090, -6.969112962950057444 ) ) ;
#6165=CARTESIAN_POINT ( 'NONE',  ( 2.862020680886599333, -78.79547149457074795, 4.100960146803977580 ) ) ;
#6166=CARTESIAN_POINT ( 'NONE',  ( 4.725907263620372056, -67.09547149457073090, 1.635492904037598283 ) ) ;
#6167=CARTESIAN_POINT ( 'NONE',  ( -4.784657899331191011, -69.60452850542925773, -1.454677039711773867 ) ) ;
#6169=CARTESIAN_POINT ( 'NONE',  ( -4.194503406049384431, -62.44547149457072521, -3.171033256558012159 ) ) ;
#6171=CARTESIAN_POINT ( 'NONE',  ( 6.686770931921522276, -59.10452850542926484, 2.072711028461649008 ) ) ;
#6178=AXIS2_PLACEMENT_3D ( 'NONE', #3924, #3881, #757 ) ;
#6180=CARTESIAN_POINT ( 'NONE',  ( 3.015831842038235955, -91.80452850542926058, 3.989209796945429432 ) ) ;
#6181=CARTESIAN_POINT ( 'NONE',  ( 4.784657899331210551, -80.10452850542925773, 1.454677039711774533 ) ) ;
#6182=CARTESIAN_POINT ( 'NONE',  ( -0.09506052544084224454, -60.00452850542925631, -4.999999999999997335 ) ) ;
#6183=CARTESIAN_POINT ( 'NONE',  ( 1.840261337453221291, -85.69547149457073942, -2.371175808195584267 ) ) ;
#6184=CARTESIAN_POINT ( 'NONE',  ( -1.686450176301619308, -59.29547149457074084, -2.482926158054096000 ) ) ;
#6185=CARTESIAN_POINT ( 'NONE',  ( 3.015831842038233290, -70.80452850542926058, 3.989209796945429432 ) ) ;
#6186=CARTESIAN_POINT ( 'NONE',  ( 4.037591185471444355, -86.70452850542925205, -5.718994135553947977 ) ) ;
#6187=CARTESIAN_POINT ( 'NONE',  ( 1.840261337453222845, -97.69547149457076785, -2.371175808195584267 ) ) ;
#6192=CARTESIAN_POINT ( 'NONE',  ( 4.194503406049340022, -92.55452850542924637, -3.171033256558100977 ) ) ;
#6193=CARTESIAN_POINT ( 'NONE',  ( -2.610703060766966122, -69.45452850542925205, -1.773238653441072232 ) ) ;
#6194=CARTESIAN_POINT ( 'NONE',  ( 6.686770931921477867, -76.39547149457074227, -2.072711028461788896 ) ) ;
#6195=CARTESIAN_POINT ( 'NONE',  ( -4.725907263620319654, -90.90452850542926910, 1.635492904037698647 ) ) ;
#6197=CARTESIAN_POINT ( 'NONE',  ( -4.725907263620350740, -95.59547149457074511, -1.635492904037597617 ) ) ;
#6198=CARTESIAN_POINT ( 'NONE',  ( 0.09506052544083994083, -85.50452850542926342, 2.999999999999997780 ) ) ;
#6203=CARTESIAN_POINT ( 'NONE',  ( -1.529537955723671905, -61.35452850542925773, 5.030887037049979860 ) ) ;
#6204=CARTESIAN_POINT ( 'NONE',  ( -6.686770931921459216, -71.89547149457074227, 2.072711028461789784 ) ) ;
#6206=CARTESIAN_POINT ( 'NONE',  ( 5.186942113755784511, -97.00000000000001421, 1.679816887229922839 ) ) ;
#6207=CARTESIAN_POINT ( 'NONE',  ( 1.719659006605285034, -70.84547149457074511, -4.969112962950050338 ) ) ;
#6208=CARTESIAN_POINT ( 'NONE',  ( -3.015831842038129817, -72.19547149457073942, 3.989209796945492048 ) ) ;
#6209=CARTESIAN_POINT ( 'NONE',  ( -0.09506052544081705635, -93.00452850542926342, -2.999999999999997780 ) ) ;
#6211=CARTESIAN_POINT ( 'NONE',  ( -3.015831842038216415, -66.30452850542926058, -3.989209796945429432 ) ) ;
#6212=CARTESIAN_POINT ( 'NONE',  ( 2.179377348189632357, -96.64547149457075648, 7.030887037049939003 ) ) ;
#6213=CARTESIAN_POINT ( 'NONE',  ( -0.09506052544083808120, -93.00452850542926342, -4.999999999999997335 ) ) ;
#6216=CARTESIAN_POINT ( 'NONE',  ( -3.989863994746656317E-14, -97.00000000000000000, -4.999999999999997335 ) ) ;
#6221=CARTESIAN_POINT ( 'NONE',  ( 4.312004677471078296, -88.95452850542922363, 3.009306630940844496 ) ) ;
#6222=CARTESIAN_POINT ( 'NONE',  ( 4.725907263620374721, -91.09547149457074511, 1.635492904037598283 ) ) ;
#6223=CARTESIAN_POINT ( 'NONE',  ( -0.09506052544084186984, -63.00452850542925631, -4.999999999999997335 ) ) ;
#6225=CARTESIAN_POINT ( 'NONE',  ( 2.823794231030060331, -79.09547149457075932, 1.017458915287723809 ) ) ;
#6226=CARTESIAN_POINT ( 'NONE',  ( 4.784657899331179465, -91.39547149457075648, -1.454677039711874009 ) ) ;
#6227=CARTESIAN_POINT ( 'NONE',  ( 4.725907263620340082, -65.40452850542925489, -1.635492904037697981 ) ) ;
#6228=CARTESIAN_POINT ( 'NONE',  ( -6.013306294175152722, -75.45452850542925205, -4.245374608440613429 ) ) ;
#6229=CARTESIAN_POINT ( 'NONE',  ( 1.686450176301638182, -93.79547149457076216, 2.482926158054096000 ) ) ;
#6233=CARTESIAN_POINT ( 'NONE',  ( 4.784657899331211439, -92.10452850542925773, 1.454677039711774533 ) ) ;
#6234=CARTESIAN_POINT ( 'NONE',  ( -1.840261337453252155, -72.30452850542926058, -2.371175808195547852 ) ) ;
#6235=CARTESIAN_POINT ( 'NONE',  ( -7.360235569667860744, -60.75452850542924921, 0.09995255151731782806 ) ) ;
#6237=CARTESIAN_POINT ( 'NONE',  ( -6.013306294175058575, -84.04547149457074795, 4.245374608440741326 ) ) ;
#6238=CARTESIAN_POINT ( 'NONE',  ( 3.015831842038236399, -94.80452850542924637, 3.989209796945429432 ) ) ;
#6239=CARTESIAN_POINT ( 'NONE',  ( 4.784657899331179465, -91.39547149457075648, -1.454677039711874009 ) ) ;
#6240=CARTESIAN_POINT ( 'NONE',  ( -1.069819614139536412, -90.15452850542926910, -2.969112962950023249 ) ) ;
#6244=COLOUR_RGB ( '', 0.09019608, 0.27058824, 0.51372549) ;
#6247=CARTESIAN_POINT ( 'NONE',  ( -1.529537955723672349, -58.35452850542924352, 5.030887037049979860 ) ) ;
#6248=CARTESIAN_POINT ( 'NONE',  ( 2.179377348189628361, -69.64547149457072805, 7.030887037049939003 ) ) ;
#6250=CARTESIAN_POINT ( 'NONE',  ( 5.478861521945414204, -97.00000000000005684, 0.9668479938647240868 ) ) ;
#6251=CARTESIAN_POINT ( 'NONE',  ( -4.784657899331159037, -68.89547149457074227, 1.454677039711874675 ) ) ;
#6252=CARTESIAN_POINT ( 'NONE',  ( -1.529537955723778042, -65.14547149457074227, -5.030887037049945221 ) ) ;
#6254=CARTESIAN_POINT ( 'NONE',  ( -4.194503406049321370, -58.05452850542925347, 3.171033256558100533 ) ) ;
#6257=CARTESIAN_POINT ( 'NONE',  ( -4.312004677471057867, -72.45452850542922363, -3.009306630940844052 ) ) ;
#6259=CARTESIAN_POINT ( 'NONE',  ( -1.529537955723778486, -62.14547149457074227, -5.030887037049945221 ) ) ;
#6261=CLOSED_SHELL ( 'NONE', ( #1589, #4700, #3945, #4333, #3654 ) ) ;
#6265=CARTESIAN_POINT ( 'NONE',  ( -0.09506052544083767875, -96.00452850542926342, -4.999999999999997335 ) ) ;
#6266=CARTESIAN_POINT ( 'NONE',  ( -1.719659006605371854, -78.15452850542925489, -4.969112962950016588 ) ) ;
#6267=CARTESIAN_POINT ( 'NONE',  ( -3.015831842038127153, -90.19547149457073942, 3.989209796945492048 ) ) ;
#6268=CARTESIAN_POINT ( 'NONE',  ( -4.725907263620324095, -57.90452850542925489, 1.635492904037698647 ) ) ;
#6269=CARTESIAN_POINT ( 'NONE',  ( -2.493201789345290464, -83.44547149457073942, -1.934965279058240561 ) ) ;
#6270=CARTESIAN_POINT ( 'NONE',  ( -6.013306294175152722, -75.45452850542925205, -4.245374608440613429 ) ) ;
#6271=CARTESIAN_POINT ( 'NONE',  ( -4.194503406049383543, -83.44547149457071100, -3.171033256558012159 ) ) ;
#6272=CARTESIAN_POINT ( 'NONE',  ( -4.312004677471060532, -63.45452850542926626, -3.009306630940844052 ) ) ;
#6273=CARTESIAN_POINT ( 'NONE',  ( 7.360235569667877620, -74.25452850542924921, -0.09995255151731691212 ) ) ;
#6274=CARTESIAN_POINT ( 'NONE',  ( 0.09506052544077819855, -91.99547149457075079, -2.999999999999997780 ) ) ;
#6279=CARTESIAN_POINT ( 'NONE',  ( 5.257311121191343695, -89.25452850542923500, -0.09995255151729466603 ) ) ;
#6280=CARTESIAN_POINT ( 'NONE',  ( -2.610703060766966566, -66.45452850542925205, -1.773238653441072232 ) ) ;
#6281=CARTESIAN_POINT ( 'NONE',  ( 1.719659006605392504, -91.65452850542925489, 4.969112962950016588 ) ) ;
#6282=CARTESIAN_POINT ( 'NONE',  ( 0.09506052544073390065, -73.99547149457075079, -6.999999999999997335 ) ) ;
#6283=CARTESIAN_POINT ( 'NONE',  ( 4.784657899331211439, -92.10452850542925773, 1.454677039711774533 ) ) ;
#6284=CARTESIAN_POINT ( 'NONE',  ( 4.312004677471013459, -82.54547149457073374, -3.009306630940932425 ) ) ;
#6285=CARTESIAN_POINT ( 'NONE',  ( -0.09506052544081930455, -75.00452850542926342, -2.999999999999997780 ) ) ;
#6289=( NAMED_UNIT ( * ) PLANE_ANGLE_UNIT ( ) SI_UNIT ( $, .RADIAN. ) );
#6290=CARTESIAN_POINT ( 'NONE',  ( -0.8796985632578772085, -94.35452850542925773, 3.030887037049973198 ) ) ;
#6291=CARTESIAN_POINT ( 'NONE',  ( 4.191402346623077868, -73.69547149457073942, -5.607243785695398941 ) ) ;
#6293=CARTESIAN_POINT ( 'NONE',  ( 4.312004677471009906, -64.54547149457073374, -3.009306630940932425 ) ) ;
#6294=CARTESIAN_POINT ( 'NONE',  ( -4.312004677470994807, -63.04547149457074084, 3.009306630940933758 ) ) ;
#6295=CARTESIAN_POINT ( 'NONE',  ( -3.015831842038216859, -60.30452850542926058, -3.989209796945429432 ) ) ;
#6298=CARTESIAN_POINT ( 'NONE',  ( -5.257311121191324155, -66.75452850542923500, 0.09995255151729526277 ) ) ;
#6299=CARTESIAN_POINT ( 'NONE',  ( 0.09506052544073689825, -97.99547149457075079, -6.999999999999997335 ) ) ;
#6305=CARTESIAN_POINT ( 'NONE',  ( -2.862020680886493640, -82.20452850542925205, 4.100960146804039752 ) ) ;
#6306=CARTESIAN_POINT ( 'NONE',  ( -2.862020680886579349, -86.29547149457074795, -4.100960146803977580 ) ) ;
#6307=CARTESIAN_POINT ( 'NONE',  ( 4.784657899331207886, -62.10452850542925063, 1.454677039711774533 ) ) ;
#6308=CARTESIAN_POINT ( 'NONE',  ( -1.840261337453201529, -69.19547149457073942, 2.371175808195584267 ) ) ;
#6310=CARTESIAN_POINT ( 'NONE',  ( -2.179377348189461827, -76.35452850542924352, 7.030887037049988741 ) ) ;
#6311=CARTESIAN_POINT ( 'NONE',  ( -1.719659006605264162, -90.34547149457074511, 4.969112962950051227 ) ) ;
#6312=CARTESIAN_POINT ( 'NONE',  ( 1.529537955723688780, -62.85452850542925063, -5.030887037049978971 ) ) ;
#6313=CARTESIAN_POINT ( 'NONE',  ( 4.037591185471442579, -77.70452850542925205, -5.718994135553947977 ) ) ;
#6315=CARTESIAN_POINT ( 'NONE',  ( -2.493201789345290020, -86.44547149457073942, -1.934965279058240561 ) ) ;
#6322=CARTESIAN_POINT ( 'NONE',  ( -3.015831842038213750, -90.30452850542926058, -3.989209796945429432 ) ) ;
#6323=CARTESIAN_POINT ( 'NONE',  ( 0.09506052544083691547, -61.50452850542925631, 2.999999999999997780 ) ) ;
#6325=CARTESIAN_POINT ( 'NONE',  ( 2.862020680886516288, -92.70452850542926626, -4.100960146804039752 ) ) ;
#6326=CARTESIAN_POINT ( 'NONE',  ( 6.628020296210686446, -70.09547149457073090, 2.253526892787472757 ) ) ;
#6327=CARTESIAN_POINT ( 'NONE',  ( 4.725907263620374721, -88.09547149457074511, 1.635492904037598283 ) ) ;
#6328=CARTESIAN_POINT ( 'NONE',  ( -3.154386672714789785, -75.75452850542926342, 0.09995255151727280851 ) ) ;
#6333=CARTESIAN_POINT ( 'NONE',  ( 0.8796985632578997460, -83.85452850542927195, -3.030887037049972310 ) ) ;
#6334=CARTESIAN_POINT ( 'NONE',  ( -6.628020296210667794, -71.59547149457071669, -2.253526892787471869 ) ) ;
#6336=CARTESIAN_POINT ( 'NONE',  ( -5.257311121191325043, -68.74547149457073658, -0.09995255151718372699 ) ) ;
#6337=CARTESIAN_POINT ( 'NONE',  ( -7.360235569667856304, -95.74547149457073658, -0.09995255151716124498 ) ) ;
#6338=CARTESIAN_POINT ( 'NONE',  ( -0.09506052544081666777, -96.00452850542926342, -2.999999999999997780 ) ) ;
#6340=CARTESIAN_POINT ( 'NONE',  ( 2.862020680886513180, -68.70452850542925205, -4.100960146804039752 ) ) ;
#6342=CARTESIAN_POINT ( 'NONE',  ( -5.895805022753475733, -95.44547149457075363, -4.407101234057782868 ) ) ;
#6344=EDGE_CURVE ( 'NONE', #4707, #6384, #4476, .T. ) ;
#6346=PRODUCT_CONTEXT ( 'NONE', #2019, 'mechanical' ) ;
#6349=CARTESIAN_POINT ( 'NONE',  ( 0.09506052544086007750, -76.50452850542924921, 4.999999999999997335 ) ) ;
#6350=CARTESIAN_POINT ( 'NONE',  ( -4.784657899331156372, -92.89547149457075648, 1.454677039711874675 ) ) ;
#6351=CARTESIAN_POINT ( 'NONE',  ( -3.015831842038217303, -57.30452850542925347, -3.989209796945429432 ) ) ;
#6352=CARTESIAN_POINT ( 'NONE',  ( -2.823794231030041235, -68.59547149457073090, -1.017458915287723364 ) ) ;
#6353=CARTESIAN_POINT ( 'NONE',  ( 4.037591185471442579, -74.70452850542925205, -5.718994135553947977 ) ) ;
#6354=CARTESIAN_POINT ( 'NONE',  ( -4.725907263620352516, -86.59547149457075932, -1.635492904037597617 ) ) ;
#6355=CARTESIAN_POINT ( 'NONE',  ( -2.862020680886496748, -58.20452850542925916, 4.100960146804039752 ) ) ;
#6357=CARTESIAN_POINT ( 'NONE',  ( -6.628020296210620721, -78.90452850542925489, 2.253526892787613978 ) ) ;
#6358=CARTESIAN_POINT ( 'NONE',  ( -3.154386672714787565, -92.74547149457073658, -0.09995255151720625064 ) ) ;
#6364=CARTESIAN_POINT ( 'NONE',  ( -4.312004677471056091, -90.45452850542926626, -3.009306630940843608 ) ) ;
#6365=CARTESIAN_POINT ( 'NONE',  ( 1.069819614139554842, -58.65452850542925489, 2.969112962950023249 ) ) ;
#6366=CARTESIAN_POINT ( 'NONE',  ( 7.360235569667875843, -59.25452850542926342, -0.09995255151731691212 ) ) ;
#6367=CARTESIAN_POINT ( 'NONE',  ( -6.686770931921460992, -65.89547149457074227, 2.072711028461789784 ) ) ;
#6368=CARTESIAN_POINT ( 'NONE',  ( -2.862020680886579349, -89.29547149457074795, -4.100960146803977580 ) ) ;
#6369=CARTESIAN_POINT ( 'NONE',  ( 1.840261337453270807, -76.80452850542926058, 2.371175808195547852 ) ) ;
#6371=CARTESIAN_POINT ( 'NONE',  ( 1.686450176301586668, -86.70452850542925205, -2.482926158054133303 ) ) ;
#6372=CARTESIAN_POINT ( 'NONE',  ( 4.191402346623076980, -61.69547149457074653, -5.607243785695398941 ) ) ;
#6373=CARTESIAN_POINT ( 'NONE',  ( 5.283807651323763288, -96.99999999999990052, -2.555618791970358572 ) ) ;
#6374=CARTESIAN_POINT ( 'NONE',  ( -0.09506052544073617661, -69.49547149457075079, 4.999999999999997335 ) ) ;
#6375=CARTESIAN_POINT ( 'NONE',  ( 2.179377348189632357, -96.64547149457075648, 7.030887037049939003 ) ) ;
#6376=CARTESIAN_POINT ( 'NONE',  ( 3.015831842038231958, -58.80452850542925347, 3.989209796945429432 ) ) ;
#6380=CARTESIAN_POINT ( 'NONE',  ( 1.529537955723689002, -65.85452850542924352, -5.030887037049978971 ) ) ;
#6381=CARTESIAN_POINT ( 'NONE',  ( -4.191402346623055664, -93.19547149457075363, 5.607243785695398941 ) ) ;
#6384=VERTEX_POINT ( 'NONE', #6265 ) ;
#6389=CARTESIAN_POINT ( 'NONE',  ( -0.09506052544083998246, -78.00452850542926342, -4.999999999999997335 ) ) ;
#6390=CARTESIAN_POINT ( 'NONE',  ( -4.194503406049383543, -86.44547149457071100, -3.171033256558012159 ) ) ;
#6392=CARTESIAN_POINT ( 'NONE',  ( 4.306376502030560438, -96.99999999999997158, 1.631842557598098375 ) ) ;
#6393=CARTESIAN_POINT ( 'NONE',  ( 1.069819614139494002, -73.84547149457073090, -2.969112962950042789 ) ) ;
#6394=CARTESIAN_POINT ( 'NONE',  ( 4.037591185471443467, -80.70452850542925205, -5.718994135553947977 ) ) ;
#6395=CARTESIAN_POINT ( 'NONE',  ( 4.194503406049402194, -87.94547149457072521, 3.171033256558012159 ) ) ;
#6396=CARTESIAN_POINT ( 'NONE',  ( 2.862020680886511848, -59.70452850542925205, -4.100960146804039752 ) ) ;
#6397=CARTESIAN_POINT ( 'NONE',  ( 6.686770931921523164, -74.10452850542924352, 2.072711028461649008 ) ) ;
#6398=CARTESIAN_POINT ( 'NONE',  ( 3.154386672714809770, -85.24547149457075079, 0.09995255151720662534 ) ) ;
#6403=CARTESIAN_POINT ( 'NONE',  ( -3.015831842038214194, -81.30452850542926058, -3.989209796945429432 ) ) ;
#6404=CARTESIAN_POINT ( 'NONE',  ( -0.8796985632578812053, -61.35452850542925773, 3.030887037049973198 ) ) ;
#6406=CARTESIAN_POINT ( 'NONE',  ( -6.686770931921507177, -60.60452850542926484, -2.072711028461647675 ) ) ;
#6407=CARTESIAN_POINT ( 'NONE',  ( -5.895805022753477509, -74.44547149457072521, -4.407101234057782868 ) ) ;
#6408=CARTESIAN_POINT ( 'NONE',  ( -0.09506052544073352595, -90.49547149457073658, 4.999999999999997335 ) ) ;
#6409=CARTESIAN_POINT ( 'NONE',  ( 1.069819614139556840, -73.65452850542925489, 2.969112962950023249 ) ) ;
#6411=CARTESIAN_POINT ( 'NONE',  ( 2.610703060766984773, -85.95452850542925205, 1.773238653441072232 ) ) ;
#6412=CARTESIAN_POINT ( 'NONE',  ( 4.037591185471560706, -60.79547149457074084, 5.718994135553860936 ) ) ;
#6414=CARTESIAN_POINT ( 'NONE',  ( -4.725907263620355181, -65.59547149457073090, -1.635492904037597617 ) ) ;
#6415=CARTESIAN_POINT ( 'NONE',  ( 3.015831842038146693, -61.69547149457073942, -3.989209796945492048 ) ) ;
#6419=CARTESIAN_POINT ( 'NONE',  ( 1.529537955723688780, -62.85452850542925063, -5.030887037049978971 ) ) ;
#6420=CARTESIAN_POINT ( 'NONE',  ( -6.013306294175058575, -93.04547149457074795, 4.245374608440741326 ) ) ;
#6427=CARTESIAN_POINT ( 'NONE',  ( 4.784657899331209663, -74.10452850542925773, 1.454677039711774533 ) ) ;
#6428=CARTESIAN_POINT ( 'NONE',  ( -1.529537955723776488, -83.14547149457071384, -5.030887037049945221 ) ) ;
#6429=CARTESIAN_POINT ( 'NONE',  ( 4.227511635438607307, -96.99999999999997158, 2.381263360235327919 ) ) ;
#6430=CARTESIAN_POINT ( 'NONE',  ( -2.823794231030041235, -71.59547149457071669, -1.017458915287723364 ) ) ;
#6431=CARTESIAN_POINT ( 'NONE',  ( -4.191402346623180009, -69.30452850542926058, -5.607243785695311900 ) ) ;
#6432=CARTESIAN_POINT ( 'NONE',  ( 4.194503406049402194, -78.94547149457071100, 3.171033256558012159 ) ) ;
#6435=CARTESIAN_POINT ( 'NONE',  ( -5.895805022753386027, -73.05452850542926058, 4.407101234057909878 ) ) ;
#6436=CARTESIAN_POINT ( 'NONE',  ( -2.823794231030038571, -89.59547149457074511, -1.017458915287723364 ) ) ;
#6438=CARTESIAN_POINT ( 'NONE',  ( -4.481820730511953954E-14, -57.99999999999999289, -4.999999999999997335 ) ) ;
#6440=CARTESIAN_POINT ( 'NONE',  ( -4.784657899331190123, -84.60452850542927195, -1.454677039711773867 ) ) ;
#6442=CARTESIAN_POINT ( 'NONE',  ( -4.312004677471056979, -84.45452850542923784, -3.009306630940843608 ) ) ;
#6443=CARTESIAN_POINT ( 'NONE',  ( 0.09506052544083654077, -58.50452850542925631, 2.999999999999997780 ) ) ;
#6445=CARTESIAN_POINT ( 'NONE',  ( -1.529537955723669684, -82.35452850542922931, 5.030887037049979860 ) ) ;
#6446=CARTESIAN_POINT ( 'NONE',  ( -4.037591185471545607, -71.29547149457074795, -5.718994135553860936 ) ) ;
#6449=CARTESIAN_POINT ( 'NONE',  ( -1.719659006605265050, -81.34547149457073090, 4.969112962950051227 ) ) ;
#6450=CARTESIAN_POINT ( 'NONE',  ( -2.493201789345251829, -76.05452850542926058, 1.934965279058294518 ) ) ;
#6454=CARTESIAN_POINT ( 'NONE',  ( -2.610703060766962569, -90.45452850542926626, -1.773238653441072232 ) ) ;
#6455=CARTESIAN_POINT ( 'NONE',  ( 6.686770931921476979, -64.39547149457074227, -2.072711028461788896 ) ) ;
#6458=CARTESIAN_POINT ( 'NONE',  ( -2.862020680886494084, -79.20452850542925205, 4.100960146804039752 ) ) ;
#6459=CARTESIAN_POINT ( 'NONE',  ( 4.194503406049400418, -60.94547149457072521, 3.171033256558012159 ) ) ;
#6463=CARTESIAN_POINT ( 'NONE',  ( 0.09506052544085781542, -58.50452850542925631, 4.999999999999997335 ) ) ;
#6464=CARTESIAN_POINT ( 'NONE',  ( 6.013306294175080779, -94.54547149457073374, -4.245374608440741326 ) ) ;
#6466=CARTESIAN_POINT ( 'NONE',  ( -3.015831842038215527, -72.30452850542926058, -3.989209796945429432 ) ) ;
#6470=CARTESIAN_POINT ( 'NONE',  ( -4.725907263620353405, -77.59547149457074511, -1.635492904037597617 ) ) ;
#6472=CARTESIAN_POINT ( 'NONE',  ( 4.784657899331180353, -97.39547149457074227, -1.454677039711874009 ) ) ;
#6473=CARTESIAN_POINT ( 'NONE',  ( 2.179377348189481367, -71.85452850542924352, -7.030887037049986077 ) ) ;
#6475=CARTESIAN_POINT ( 'NONE',  ( -1.529537955723776488, -83.14547149457071384, -5.030887037049945221 ) ) ;
#6476=CARTESIAN_POINT ( 'NONE',  ( 1.719659006605388285, -58.65452850542924068, 4.969112962950016588 ) ) ;
#6478=CARTESIAN_POINT ( 'NONE',  ( 2.369498399071223727, -64.65452850542924068, 6.969112962950009482 ) ) ;
#6479=CARTESIAN_POINT ( 'NONE',  ( -1.686450176301616199, -83.29547149457074795, -2.482926158054096000 ) ) ;
#6482=CARTESIAN_POINT ( 'NONE',  ( 4.784657899331211439, -92.10452850542925773, 1.454677039711774533 ) ) ;
#6483=CARTESIAN_POINT ( 'NONE',  ( -5.257311121191322378, -90.75452850542924921, 0.09995255151729526277 ) ) ;
#6485=CARTESIAN_POINT ( 'NONE',  ( -2.862020680886493640, -82.20452850542925205, 4.100960146804039752 ) ) ;
#6486=CARTESIAN_POINT ( 'NONE',  ( 2.823794231030062551, -97.09547149457074511, 1.017458915287723809 ) ) ;
#6488=CARTESIAN_POINT ( 'NONE',  ( 4.725907263620340970, -83.40452850542925489, -1.635492904037697981 ) ) ;
#6489=CARTESIAN_POINT ( 'NONE',  ( -5.895805022753479285, -62.44547149457074653, -4.407101234057782868 ) ) ;
#6490=CARTESIAN_POINT ( 'NONE',  ( -2.823794231030022583, -63.90452850542925489, 1.017458915287783316 ) ) ;
#6493=CARTESIAN_POINT ( 'NONE',  ( 2.493201789345272257, -83.55452850542926058, -1.934965279058294518 ) ) ;
#6494=CARTESIAN_POINT ( 'NONE',  ( -0.09506052544071567911, -63.49547149457075079, 6.999999999999997335 ) ) ;
#6497=CARTESIAN_POINT ( 'NONE',  ( -4.725907263620320542, -78.90452850542925489, 1.635492904037698647 ) ) ;
#6498=CARTESIAN_POINT ( 'NONE',  ( 7.360235569667880284, -88.24547149457073658, 0.09995255151716216091 ) ) ;
#6501=CARTESIAN_POINT ( 'NONE',  ( 3.015831842038231958, -58.80452850542925347, 3.989209796945429432 ) ) ;
#6503=CARTESIAN_POINT ( 'NONE',  ( -2.369498399071054529, -93.34547149457073090, 6.969112962950058332 ) ) ;
#6505=CARTESIAN_POINT ( 'NONE',  ( 1.719659006605390283, -73.65452850542924068, 4.969112962950016588 ) ) ;
#6512=CARTESIAN_POINT ( 'NONE',  ( -0.09506052544073428923, -84.49547149457075079, 4.999999999999997335 ) ) ;
#6514=CARTESIAN_POINT ( 'NONE',  ( -2.882544866740859746, -59.89547149457074937, 0.8366430509619596778 ) ) ;
#6515=CARTESIAN_POINT ( 'NONE',  ( 6.628020296210639373, -65.40452850542925489, -2.253526892787612645 ) ) ;
#6517=CARTESIAN_POINT ( 'NONE',  ( 2.862020680886599333, -75.79547149457074795, 4.100960146803977580 ) ) ;
#6518=CARTESIAN_POINT ( 'NONE',  ( -0.09506052544084261924, -57.00452850542924921, -4.999999999999997335 ) ) ;
#6519=CARTESIAN_POINT ( 'NONE',  ( 1.529537955723691889, -86.85452850542921510, -5.030887037049978971 ) ) ;
#6520=CARTESIAN_POINT ( 'NONE',  ( -5.895805022753386915, -64.05452850542924637, 4.407101234057909878 ) ) ;
#6522=CARTESIAN_POINT ( 'NONE',  ( -2.493201789345291353, -74.44547149457072521, -1.934965279058240561 ) ) ;
#6527=CARTESIAN_POINT ( 'NONE',  ( -4.194503406049315153, -88.05452850542921794, 3.171033256558100533 ) ) ;
#6529=CARTESIAN_POINT ( 'NONE',  ( 3.015831842038234623, -82.80452850542926058, 3.989209796945429432 ) ) ;
#6530=CARTESIAN_POINT ( 'NONE',  ( 2.823794231030062107, -94.09547149457074511, 1.017458915287723809 ) ) ;
#6532=CARTESIAN_POINT ( 'NONE',  ( -4.312004677471056091, -87.45452850542925205, -3.009306630940844052 ) ) ;
#6533=CARTESIAN_POINT ( 'NONE',  ( -0.09506052544085875911, -96.00452850542926342, -6.999999999999997335 ) ) ;
#6534=CARTESIAN_POINT ( 'NONE',  ( -0.09506052544082008171, -69.00452850542926342, -2.999999999999997780 ) ) ;
#6537=CARTESIAN_POINT ( 'NONE',  ( 2.882544866740897049, -80.10452850542927195, 0.8366430509618999478 ) ) ;
#6538=CARTESIAN_POINT ( 'NONE',  ( -6.628020296210618056, -93.90452850542926910, 2.253526892787613978 ) ) ;
#6540=CARTESIAN_POINT ( 'NONE',  ( 4.194503406049337357, -74.55452850542923215, -3.171033256558100089 ) ) ;
#6541=CARTESIAN_POINT ( 'NONE',  ( 7.360235569667880284, -91.24547149457073658, 0.09995255151716216091 ) ) ;
#6544=CARTESIAN_POINT ( 'NONE',  ( -3.154386672714791118, -68.74547149457075079, -0.09995255151720625064 ) ) ;
#6545=CARTESIAN_POINT ( 'NONE',  ( -0.09506052544084224454, -60.00452850542925631, -4.999999999999997335 ) ) ;
#6547=CARTESIAN_POINT ( 'NONE',  ( -4.191402346623055664, -90.19547149457073942, 5.607243785695398941 ) ) ;
#6549=CARTESIAN_POINT ( 'NONE',  ( -4.784657899331190123, -75.60452850542925773, -1.454677039711773867 ) ) ;
#6552=CARTESIAN_POINT ( 'NONE',  ( 1.529537955723796028, -84.64547149457074227, 5.030887037049945221 ) ) ;
#6553=CARTESIAN_POINT ( 'NONE',  ( 4.230555499402125719, -97.00000000000000000, 2.192008249831833400 ) ) ;
#6554=CARTESIAN_POINT ( 'NONE',  ( 2.610703060766943029, -64.54547149457073374, -1.773238653441125523 ) ) ;
#6555=CARTESIAN_POINT ( 'NONE',  ( 6.628020296210639373, -68.40452850542925489, -2.253526892787612645 ) ) ;
#6557=CARTESIAN_POINT ( 'NONE',  ( -4.312004677470993030, -75.04547149457074795, 3.009306630940933758 ) ) ;
#6559=CARTESIAN_POINT ( 'NONE',  ( 5.257311121191342806, -86.25452850542924921, -0.09995255151729465215 ) ) ;
#6560=CARTESIAN_POINT ( 'NONE',  ( -5.895805022753386915, -70.05452850542926058, 4.407101234057909878 ) ) ;
#6562=CARTESIAN_POINT ( 'NONE',  ( -0.8796985632579428227, -77.14547149457074227, -3.030887037049952326 ) ) ;
#6567=CARTESIAN_POINT ( 'NONE',  ( -4.784657899331189235, -90.60452850542925773, -1.454677039711773867 ) ) ;
#6569=CARTESIAN_POINT ( 'NONE',  ( 1.529537955723690335, -77.85452850542924352, -5.030887037049978971 ) ) ;
#6570=CARTESIAN_POINT ( 'NONE',  ( 1.686450176301637960, -90.79547149457074795, 2.482926158054096000 ) ) ;
#6572=CARTESIAN_POINT ( 'NONE',  ( 2.862020680886515844, -89.70452850542926626, -4.100960146804039752 ) ) ;
#6573=CARTESIAN_POINT ( 'NONE',  ( -5.895805022753383362, -94.05452850542926058, 4.407101234057909878 ) ) ;
#6574=CARTESIAN_POINT ( 'NONE',  ( -2.610703060766966566, -63.45452850542924494, -1.773238653441072232 ) ) ;
#6577=CARTESIAN_POINT ( 'NONE',  ( -1.840261337453251489, -78.30452850542926058, -2.371175808195547852 ) ) ;
#6578=CARTESIAN_POINT ( 'NONE',  ( 2.369498399071226835, -88.65452850542926910, 6.969112962950009482 ) ) ;
#6581=CARTESIAN_POINT ( 'NONE',  ( -4.191402346623057440, -84.19547149457073942, 5.607243785695398941 ) ) ;
#6584=CARTESIAN_POINT ( 'NONE',  ( -2.882544866740858414, -68.89547149457074227, 0.8366430509619596778 ) ) ;
#6589=CARTESIAN_POINT ( 'NONE',  ( -3.015831842038215971, -69.30452850542926058, -3.989209796945429432 ) ) ;
#6590=CARTESIAN_POINT ( 'NONE',  ( -0.09506052544071304233, -84.49547149457075079, 6.999999999999997335 ) ) ;
#6593=CARTESIAN_POINT ( 'NONE',  ( 4.784657899331208775, -71.10452850542925773, 1.454677039711774533 ) ) ;
#6596=CARTESIAN_POINT ( 'NONE',  ( -1.719659006605267049, -66.34547149457073090, 4.969112962950051227 ) ) ;
#6598=CARTESIAN_POINT ( 'NONE',  ( 4.194503406049402194, -96.94547149457073942, 3.171033256558012159 ) ) ;
#6599=CARTESIAN_POINT ( 'NONE',  ( 4.037591185471441690, -68.70452850542925205, -5.718994135553947977 ) ) ;
#6601=CARTESIAN_POINT ( 'NONE',  ( -4.194503406049315153, -88.05452850542921794, 3.171033256558100533 ) ) ;
#6602=( GEOMETRIC_REPRESENTATION_CONTEXT ( 3 ) GLOBAL_UNCERTAINTY_ASSIGNED_CONTEXT ( ( #1656 ) ) GLOBAL_UNIT_ASSIGNED_CONTEXT ( ( #4224, #509, #1621 ) ) REPRESENTATION_CONTEXT ( 'NONE', 'WORKASPACE' ) );
#6603=CARTESIAN_POINT ( 'NONE',  ( 7.360235569667877620, -65.25452850542926342, -0.09995255151731691212 ) ) ;
#6604=CARTESIAN_POINT ( 'NONE',  ( 1.686450176301636850, -81.79547149457074795, 2.482926158054096000 ) ) ;
#6607=CARTESIAN_POINT ( 'NONE',  ( 4.725907263620342746, -95.40452850542925489, -1.635492904037697981 ) ) ;
#6608=CARTESIAN_POINT ( 'NONE',  ( -4.784657899331189235, -87.60452850542925773, -1.454677039711773867 ) ) ;
#6610=CARTESIAN_POINT ( 'NONE',  ( -4.725907263620321430, -72.90452850542925489, 1.635492904037698647 ) ) ;
#6611=CARTESIAN_POINT ( 'NONE',  ( -0.8796985632579410463, -92.14547149457074227, -3.030887037049952326 ) ) ;
#6613=CARTESIAN_POINT ( 'NONE',  ( -1.529537955723668796, -85.35452850542924352, 5.030887037049979860 ) ) ;
#6614=CARTESIAN_POINT ( 'NONE',  ( 5.895805022753492608, -63.94547149457074653, 4.407101234057782868 ) ) ;
#6615=CARTESIAN_POINT ( 'NONE',  ( 1.069819614139555730, -64.65452850542924068, 2.969112962950023249 ) ) ;
#6619=CARTESIAN_POINT ( 'NONE',  ( 2.610703060766983885, -76.95452850542926626, 1.773238653441072232 ) ) ;
#6620=CARTESIAN_POINT ( 'NONE',  ( 0.09506052544088325340, -91.50452850542926342, 6.999999999999997335 ) ) ;
#6621=CARTESIAN_POINT ( 'NONE',  ( -7.360235569667858080, -86.74547149457075079, -0.09995255151716124498 ) ) ;
#6624=CARTESIAN_POINT ( 'NONE',  ( 1.840261337453218848, -64.69547149457073942, -2.371175808195584267 ) ) ;
#6627=CARTESIAN_POINT ( 'NONE',  ( -4.725907263620322318, -69.90452850542925489, 1.635492904037698647 ) ) ;
#6628=CARTESIAN_POINT ( 'NONE',  ( -5.895805022753477509, -77.44547149457073942, -4.407101234057782868 ) ) ;
#6630=CARTESIAN_POINT ( 'NONE',  ( -4.725907263620323207, -60.90452850542925489, 1.635492904037698647 ) ) ;
#6634=CARTESIAN_POINT ( 'NONE',  ( -0.09506052544073578803, -72.49547149457075079, 4.999999999999997335 ) ) ;
#6636=CARTESIAN_POINT ( 'NONE',  ( -2.493201789345292241, -65.44547149457075363, -1.934965279058240561 ) ) ;
#6637=CARTESIAN_POINT ( 'NONE',  ( 4.191402346623195996, -64.80452850542926058, 5.607243785695311900 ) ) ;
#6642=CARTESIAN_POINT ( 'NONE',  ( -5.257311121191323267, -81.75452850542926342, 0.09995255151729526277 ) ) ;
#6643=CARTESIAN_POINT ( 'NONE',  ( 6.013306294175167821, -61.95452850542925916, 4.245374608440616093 ) ) ;
#6644=CARTESIAN_POINT ( 'NONE',  ( -0.8796985632579424896, -80.14547149457074227, -3.030887037049952326 ) ) ;
#6650=CARTESIAN_POINT ( 'NONE',  ( -3.015831842038214639, -78.30452850542926058, -3.989209796945429432 ) ) ;
#6652=CARTESIAN_POINT ( 'NONE',  ( -4.312004677471057867, -75.45452850542926626, -3.009306630940843608 ) ) ;
#6653=CARTESIAN_POINT ( 'NONE',  ( 0.09506052544077779609, -88.99547149457075079, -2.999999999999997780 ) ) ;
#6655=CARTESIAN_POINT ( 'NONE',  ( 4.194503406049402194, -96.94547149457073942, 3.171033256558012159 ) ) ;
#6656=CARTESIAN_POINT ( 'NONE',  ( -4.191402346623060104, -63.19547149457074653, 5.607243785695398941 ) ) ;
#6657=CARTESIAN_POINT ( 'NONE',  ( 0.09506052544083806732, -70.50452850542926342, 2.999999999999997780 ) ) ;
#6661=CARTESIAN_POINT ( 'NONE',  ( 2.823794231030040791, -77.40452850542925489, -1.017458915287783316 ) ) ;
#6662=CARTESIAN_POINT ( 'NONE',  ( -6.686770931921503625, -93.60452850542925773, -2.072711028461647675 ) ) ;
#6663=CARTESIAN_POINT ( 'NONE',  ( 2.179377348189631025, -90.64547149457075648, 7.030887037049939003 ) ) ;
#6666=CARTESIAN_POINT ( 'NONE',  ( 1.069819614139493114, -67.84547149457071669, -2.969112962950042789 ) ) ;
#6669=CARTESIAN_POINT ( 'NONE',  ( 4.194503406049335581, -65.55452850542923215, -3.171033256558100089 ) ) ;
#6670=CARTESIAN_POINT ( 'NONE',  ( 5.895805022753496161, -75.94547149457073942, 4.407101234057782868 ) ) ;
#6671=( NAMED_UNIT ( * ) SI_UNIT ( $, .STERADIAN. ) SOLID_ANGLE_UNIT ( ) );
#6673=CARTESIAN_POINT ( 'NONE',  ( -5.257311121191324155, -69.75452850542926342, 0.09995255151729526277 ) ) ;
#6676=CARTESIAN_POINT ( 'NONE',  ( 0.09506052544075450916, -70.99547149457075079, -4.999999999999997335 ) ) ;
#6678=CARTESIAN_POINT ( 'NONE',  ( -2.862020680886578461, -95.29547149457074795, -4.100960146803977580 ) ) ;
#6679=CARTESIAN_POINT ( 'NONE',  ( 2.369498399071223727, -64.65452850542924068, 6.969112962950009482 ) ) ;
#6682=CARTESIAN_POINT ( 'NONE',  ( 3.015831842038235067, -85.80452850542926058, 3.989209796945429432 ) ) ;
#6683=EDGE_LOOP ( 'NONE', ( #5468, #4938, #5619 ) ) ;
#6685=CARTESIAN_POINT ( 'NONE',  ( 4.194503406049339134, -86.55452850542926058, -3.171033256558100089 ) ) ;
#6686=CARTESIAN_POINT ( 'NONE',  ( -2.862020680886494528, -76.20452850542926626, 4.100960146804039752 ) ) ;
#6688=CARTESIAN_POINT ( 'NONE',  ( 4.784657899331208775, -71.10452850542925773, 1.454677039711774533 ) ) ;
#6689=CARTESIAN_POINT ( 'NONE',  ( 1.686450176301637516, -87.79547149457074795, 2.482926158054096000 ) ) ;
#6690=CARTESIAN_POINT ( 'NONE',  ( -1.069819614139476460, -63.34547149457073800, 2.969112962950044121 ) ) ;
#6691=CARTESIAN_POINT ( 'NONE',  ( 1.529537955723690112, -77.85452850542922931, -5.030887037049978971 ) ) ;
#6692=CARTESIAN_POINT ( 'NONE',  ( -0.09506052544085952238, -90.00452850542926342, -6.999999999999997335 ) ) ;
#6694=CARTESIAN_POINT ( 'NONE',  ( -2.882544866740879286, -60.60452850542926484, -0.8366430509618996147 ) ) ;
#6698=CARTESIAN_POINT ( 'NONE',  ( -2.882544866740877509, -75.60452850542924352, -0.8366430509618996147 ) ) ;
#6699=CARTESIAN_POINT ( 'NONE',  ( -4.191402346623177344, -87.30452850542926058, -5.607243785695311900 ) ) ;
#6700=CARTESIAN_POINT ( 'NONE',  ( -4.037591185471544719, -80.29547149457074795, -5.718994135553860936 ) ) ;
#6703=CARTESIAN_POINT ( 'NONE',  ( 1.686450176301634185, -63.79547149457074084, 2.482926158054096000 ) ) ;
#6709=CARTESIAN_POINT ( 'NONE',  ( 1.719659006605389173, -64.65452850542925489, 4.969112962950016588 ) ) ;
#6711=CARTESIAN_POINT ( 'NONE',  ( -4.191402346623057440, -84.19547149457073942, 5.607243785695398941 ) ) ;
#6714=CARTESIAN_POINT ( 'NONE',  ( 5.257311121191341030, -76.24547149457073658, 0.09995255151718437925 ) ) ;
#6715=CARTESIAN_POINT ( 'NONE',  ( 0.09506052544075488386, -73.99547149457075079, -4.999999999999997335 ) ) ;
#6716=CARTESIAN_POINT ( 'NONE',  ( -2.862020680886495416, -70.20452850542925205, 4.100960146804039752 ) ) ;
#6720=CARTESIAN_POINT ( 'NONE',  ( -4.194503406049384431, -74.44547149457071100, -3.171033256558012159 ) ) ;
#6722=CARTESIAN_POINT ( 'NONE',  ( 0.09506052544087986722, -64.50452850542926342, 6.999999999999997335 ) ) ;
#6728=CARTESIAN_POINT ( 'NONE',  ( 5.257311121191342806, -86.25452850542924921, -0.09995255151729465215 ) ) ;
#6729=CARTESIAN_POINT ( 'NONE',  ( -4.194503406049316041, -79.05452850542921794, 3.171033256558100533 ) ) ;
#6731=CARTESIAN_POINT ( 'NONE',  ( -4.784657899331190123, -75.60452850542925773, -1.454677039711773867 ) ) ;
#6732=CARTESIAN_POINT ( 'NONE',  ( 2.493201789345310893, -84.94547149457073942, 1.934965279058241006 ) ) ;
#6734=CARTESIAN_POINT ( 'NONE',  ( 0.09506052544077440991, -61.99547149457073658, -2.999999999999997780 ) ) ;
#6735=CARTESIAN_POINT ( 'NONE',  ( 4.784657899331209663, -77.10452850542925773, 1.454677039711774533 ) ) ;
#6736=CARTESIAN_POINT ( 'NONE',  ( 5.895805022753407343, -86.55452850542926058, -4.407101234057908989 ) ) ;
#6737=CARTESIAN_POINT ( 'NONE',  ( -2.493201789345254049, -61.05452850542925347, 1.934965279058294518 ) ) ;
#6742=CARTESIAN_POINT ( 'NONE',  ( 3.154386672714807105, -65.25452850542926342, -0.09995255151727241993 ) ) ;
#6743=CARTESIAN_POINT ( 'NONE',  ( -5.895805022753386027, -79.05452850542926058, 4.407101234057909878 ) ) ;
#6744=CARTESIAN_POINT ( 'NONE',  ( 5.895805022753496161, -81.94547149457073942, 4.407101234057782868 ) ) ;
#6748=CARTESIAN_POINT ( 'NONE',  ( -0.8796985632578782077, -85.35452850542924352, 3.030887037049973198 ) ) ;
#6751=CARTESIAN_POINT ( 'NONE',  ( 5.257311121191341918, -68.25452850542926342, -0.09995255151729465215 ) ) ;
#6752=CARTESIAN_POINT ( 'NONE',  ( 0.09506052544073424759, -76.99547149457075079, -6.999999999999997335 ) ) ;
#6755=CARTESIAN_POINT ( 'NONE',  ( -2.862020680886580681, -77.29547149457074795, -4.100960146803977580 ) ) ;
#6756=CARTESIAN_POINT ( 'NONE',  ( 1.719659006605284590, -67.84547149457070248, -4.969112962950050338 ) ) ;
#6757=CARTESIAN_POINT ( 'NONE',  ( 4.312004677471073855, -64.95452850542926626, 3.009306630940844496 ) ) ;
#6760=CARTESIAN_POINT ( 'NONE',  ( 4.784657899331176800, -70.39547149457074227, -1.454677039711874009 ) ) ;
#6761=CARTESIAN_POINT ( 'NONE',  ( 6.013306294175167821, -64.95452850542926626, 4.245374608440616093 ) ) ;
#6766=CARTESIAN_POINT ( 'NONE',  ( 4.725907263620340970, -83.40452850542925489, -1.635492904037697981 ) ) ;
#6767=CARTESIAN_POINT ( 'NONE',  ( -1.529537955723670128, -79.35452850542925773, 5.030887037049979860 ) ) ;
#6769=CARTESIAN_POINT ( 'NONE',  ( -1.529537955723670350, -76.35452850542925773, 5.030887037049979860 ) ) ;
#6770=CARTESIAN_POINT ( 'NONE',  ( 1.686450176301636183, -78.79547149457074795, 2.482926158054096000 ) ) ;
#6771=CARTESIAN_POINT ( 'NONE',  ( 1.069819614139492447, -61.84547149457074511, -2.969112962950042789 ) ) ;
#6772=CARTESIAN_POINT ( 'NONE',  ( 5.257311121191341918, -71.25452850542923500, -0.09995255151729465215 ) ) ;
#6773=CARTESIAN_POINT ( 'NONE',  ( -2.369498399071205075, -90.15452850542926910, -6.969112962950009482 ) ) ;
#6777=CARTESIAN_POINT ( 'NONE',  ( -1.840261337453198198, -93.19547149457075363, 2.371175808195584267 ) ) ;
#6784=CARTESIAN_POINT ( 'NONE',  ( -2.882544866740877954, -72.60452850542924352, -0.8366430509618996147 ) ) ;
#6785=CARTESIAN_POINT ( 'NONE',  ( 0.09506052544073462229, -79.99547149457075079, -6.999999999999997335 ) ) ;
#6787=CARTESIAN_POINT ( 'NONE',  ( -3.015831842038126709, -93.19547149457075363, 3.989209796945492048 ) ) ;
#6788=CARTESIAN_POINT ( 'NONE',  ( 2.493201789345272701, -89.55452850542926058, -1.934965279058294518 ) ) ;
#6794=CARTESIAN_POINT ( 'NONE',  ( -4.312004677471061420, -57.45452850542925916, -3.009306630940844052 ) ) ;
#6795=CARTESIAN_POINT ( 'NONE',  ( -2.369498399071058969, -66.34547149457073090, 6.969112962950058332 ) ) ;
#6797=CARTESIAN_POINT ( 'NONE',  ( 3.015831842038149357, -79.69547149457075363, -3.989209796945492048 ) ) ;
#6798=CARTESIAN_POINT ( 'NONE',  ( 4.312004677471011682, -67.54547149457074795, -3.009306630940933314 ) ) ;
#6799=CARTESIAN_POINT ( 'NONE',  ( -4.312004677471058756, -66.45452850542925205, -3.009306630940844052 ) ) ;
#6801=CARTESIAN_POINT ( 'NONE',  ( 4.725907263620371168, -61.09547149457074511, 1.635492904037598283 ) ) ;
#6803=CARTESIAN_POINT ( 'NONE',  ( 4.191402346623195996, -61.80452850542926058, 5.607243785695311900 ) ) ;
#6808=CARTESIAN_POINT ( 'NONE',  ( 3.015831842038234623, -82.80452850542926058, 3.989209796945429432 ) ) ;
#6809=CARTESIAN_POINT ( 'NONE',  ( 3.015831842038233734, -73.80452850542926058, 3.989209796945429432 ) ) ;
#6811=CARTESIAN_POINT ( 'NONE',  ( 4.725907263620339194, -62.40452850542925489, -1.635492904037697981 ) ) ;
#6812=CARTESIAN_POINT ( 'NONE',  ( 2.610703060766945693, -76.54547149457074795, -1.773238653441125523 ) ) ;
#6813=CARTESIAN_POINT ( 'NONE',  ( 5.257311121191342806, -94.24547149457070816, 0.09995255151718437925 ) ) ;
#6815=CARTESIAN_POINT ( 'NONE',  ( -0.09506052544084073186, -72.00452850542926342, -4.999999999999997335 ) ) ;
#6816=CARTESIAN_POINT ( 'NONE',  ( 6.013306294175171374, -91.95452850542925205, 4.245374608440616093 ) ) ;
#6817=CARTESIAN_POINT ( 'NONE',  ( -1.686450176301614645, -95.29547149457076216, -2.482926158054096000 ) ) ;
#6821=CARTESIAN_POINT ( 'NONE',  ( 4.784657899331211439, -86.10452850542925773, 1.454677039711774533 ) ) ;
#6822=CARTESIAN_POINT ( 'NONE',  ( 0.8796985632578985248, -71.85452850542924352, -3.030887037049972310 ) ) ;
#6823=CARTESIAN_POINT ( 'NONE',  ( 2.179377348189629249, -75.64547149457072805, 7.030887037049939003 ) ) ;
#6824=CARTESIAN_POINT ( 'NONE',  ( 2.862020680886516288, -92.70452850542926626, -4.100960146804039752 ) ) ;
#6825=CARTESIAN_POINT ( 'NONE',  ( -1.529537955723774934, -92.14547149457074227, -5.030887037049945221 ) ) ;
#6826=CARTESIAN_POINT ( 'NONE',  ( 1.686450176301586223, -83.70452850542925205, -2.482926158054133303 ) ) ;
#6832=CARTESIAN_POINT ( 'NONE',  ( -3.015831842038217303, -57.30452850542925347, -3.989209796945429432 ) ) ;
#6833=CARTESIAN_POINT ( 'NONE',  ( -2.179377348189611485, -74.14547149457074227, -7.030887037049939003 ) ) ;
#6835=CARTESIAN_POINT ( 'NONE',  ( 3.372186075517463966, -96.99999999999994316, -4.939745490940889994 ) ) ;
#6836=CARTESIAN_POINT ( 'NONE',  ( 2.862020680886599333, -72.79547149457074795, 4.100960146803977580 ) ) ;
#6837=CARTESIAN_POINT ( 'NONE',  ( -4.312004677470994807, -66.04547149457074795, 3.009306630940933758 ) ) ;
#6838=CARTESIAN_POINT ( 'NONE',  ( -4.312004677471060532, -60.45452850542923784, -3.009306630940844052 ) ) ;
#6841=CARTESIAN_POINT ( 'NONE',  ( -4.725907263620356069, -59.59547149457074511, -1.635492904037597617 ) ) ;
#6842=CARTESIAN_POINT ( 'NONE',  ( -4.312004677471055203, -93.45452850542922363, -3.009306630940844052 ) ) ;
#6851=CARTESIAN_POINT ( 'NONE',  ( 4.784657899331211439, -86.10452850542925773, 1.454677039711774533 ) ) ;
#6852=CARTESIAN_POINT ( 'NONE',  ( -0.09506052544073315125, -93.49547149457073658, 4.999999999999997335 ) ) ;
#6853=CARTESIAN_POINT ( 'NONE',  ( 5.257311121191341030, -65.25452850542926342, -0.09995255151729466603 ) ) ;
#6854=CARTESIAN_POINT ( 'NONE',  ( 2.882544866740877954, -79.39547149457074227, -0.8366430509619593447 ) ) ;
#6855=CARTESIAN_POINT ( 'NONE',  ( -4.784657899331156372, -89.89547149457075648, 1.454677039711874675 ) ) ;
#6856=CARTESIAN_POINT ( 'NONE',  ( 4.194503406049335581, -68.55452850542926058, -3.171033256558100089 ) ) ;
#6858=CARTESIAN_POINT ( 'NONE',  ( 4.191402346623198660, -85.80452850542926058, 5.607243785695311900 ) ) ;
#6859=CARTESIAN_POINT ( 'NONE',  ( -2.610703060766923933, -96.04547149457074795, 1.773238653441125745 ) ) ;
#6863=CARTESIAN_POINT ( 'NONE',  ( 4.725907263620341858, -92.40452850542925489, -1.635492904037697981 ) ) ;
#6864=CARTESIAN_POINT ( 'NONE',  ( 1.840261337453269253, -64.80452850542926058, 2.371175808195547852 ) ) ;
#6865=CARTESIAN_POINT ( 'NONE',  ( -1.719659006605370744, -93.15452850542925489, -4.969112962950016588 ) ) ;
#6866=CARTESIAN_POINT ( 'NONE',  ( -6.686770931921459216, -74.89547149457074227, 2.072711028461789784 ) ) ;
#6867=CARTESIAN_POINT ( 'NONE',  ( 1.719659006605392504, -94.65452850542921226, 4.969112962950016588 ) ) ;
#6869=CARTESIAN_POINT ( 'NONE',  ( 2.882544866740897493, -86.10452850542924352, 0.8366430509618999478 ) ) ;
#6873=SURFACE_SIDE_STYLE ('',( #1272 ) ) ;
#6874=CARTESIAN_POINT ( 'NONE',  ( 4.784657899331207886, -59.10452850542925773, 1.454677039711774533 ) ) ;
#6875=CARTESIAN_POINT ( 'NONE',  ( 6.013306294175077227, -73.54547149457074795, -4.245374608440741326 ) ) ;
#6876=CARTESIAN_POINT ( 'NONE',  ( 4.781359098026989329, -97.00000000000001421, -3.455279123890548032 ) ) ;
#6877=CARTESIAN_POINT ( 'NONE',  ( 0.09506052544075525856, -76.99547149457073658, -4.999999999999997335 ) ) ;
#6878=CARTESIAN_POINT ( 'NONE',  ( -0.09506052544073617661, -69.49547149457075079, 4.999999999999997335 ) ) ;
#6879=CARTESIAN_POINT ( 'NONE',  ( -0.8796985632578775416, -91.35452850542925773, 3.030887037049973198 ) ) ;
#6881=CARTESIAN_POINT ( 'NONE',  ( 4.312004677471074743, -70.95452850542925205, 3.009306630940844496 ) ) ;
#6882=CARTESIAN_POINT ( 'NONE',  ( -0.09506052544073731458, -60.49547149457074369, 4.999999999999997335 ) ) ;
#6887=CARTESIAN_POINT ( 'NONE',  ( 0.09506052544085971667, -73.50452850542924921, 4.999999999999997335 ) ) ;
#6888=CARTESIAN_POINT ( 'NONE',  ( 1.719659006605287033, -91.84547149457074511, -4.969112962950050338 ) ) ;
#6890=CARTESIAN_POINT ( 'NONE',  ( 5.257311121191341030, -62.25452850542924210, -0.09995255151729466603 ) ) ;
#6892=CARTESIAN_POINT ( 'NONE',  ( -0.8796985632579428227, -77.14547149457074227, -3.030887037049952326 ) ) ;
#6893=CARTESIAN_POINT ( 'NONE',  ( -7.360235569667858968, -78.75452850542926342, 0.09995255151731782806 ) ) ;
#6894=CARTESIAN_POINT ( 'NONE',  ( -4.784657899331157260, -83.89547149457074227, 1.454677039711874675 ) ) ;
#6895=CARTESIAN_POINT ( 'NONE',  ( -4.725907263620323207, -63.90452850542925489, 1.635492904037698647 ) ) ;
#6896=CARTESIAN_POINT ( 'NONE',  ( 5.895805022753406455, -77.55452850542926058, -4.407101234057908989 ) ) ;
#6897=CARTESIAN_POINT ( 'NONE',  ( -0.09506052544075481447, -90.49547149457075079, 2.999999999999997780 ) ) ;
#6902=CARTESIAN_POINT ( 'NONE',  ( 4.194503406049340022, -89.55452850542926058, -3.171033256558100977 ) ) ;
#6903=CARTESIAN_POINT ( 'NONE',  ( -0.09506052544082008171, -69.00452850542926342, -2.999999999999997780 ) ) ;
#6904=CARTESIAN_POINT ( 'NONE',  ( -6.628020296210623385, -60.90452850542925489, 2.253526892787613978 ) ) ;
#6907=CARTESIAN_POINT ( 'NONE',  ( -2.179377348189611485, -74.14547149457074227, -7.030887037049939003 ) ) ;
#6908=CARTESIAN_POINT ( 'NONE',  ( -0.09506052544083808120, -93.00452850542926342, -4.999999999999997335 ) ) ;
#6909=CARTESIAN_POINT ( 'NONE',  ( 0.09506052544075600796, -82.99547149457075079, -4.999999999999997335 ) ) ;
#6910=CARTESIAN_POINT ( 'NONE',  ( -1.686450176301564241, -88.20452850542925205, 2.482926158054133303 ) ) ;
#6917=CARTESIAN_POINT ( 'NONE',  ( 2.882544866740898826, -95.10452850542925773, 0.8366430509618999478 ) ) ;
#6918=CARTESIAN_POINT ( 'NONE',  ( 6.628020296210686446, -70.09547149457073090, 2.253526892787472757 ) ) ;
#6919=CARTESIAN_POINT ( 'NONE',  ( 5.396415032409674239, -97.00000000000004263, 1.209399173379465786 ) ) ;
#6920=CARTESIAN_POINT ( 'NONE',  ( -0.09506052544073692601, -63.49547149457074369, 4.999999999999997335 ) ) ;
#6921=CARTESIAN_POINT ( 'NONE',  ( 4.784657899331175912, -64.39547149457074227, -1.454677039711874009 ) ) ;
#6923=CARTESIAN_POINT ( 'NONE',  ( 1.840261337453273249, -94.80452850542926058, 2.371175808195547852 ) ) ;
#6926=CARTESIAN_POINT ( 'NONE',  ( -0.09506052544084073186, -72.00452850542926342, -4.999999999999997335 ) ) ;
#6927=CARTESIAN_POINT ( 'NONE',  ( 6.628020296210689999, -97.09547149457074511, 2.253526892787472757 ) ) ;
#6933=CARTESIAN_POINT ( 'NONE',  ( -4.725907263620321430, -72.90452850542925489, 1.635492904037698647 ) ) ;
#6934=CARTESIAN_POINT ( 'NONE',  ( 5.257311121191342806, -88.24547149457073658, 0.09995255151718437925 ) ) ;
#6935=CARTESIAN_POINT ( 'NONE',  ( -1.529537955723671683, -64.35452850542924352, 5.030887037049979860 ) ) ;
#6936=CARTESIAN_POINT ( 'NONE',  ( -2.493201789345291797, -71.44547149457072521, -1.934965279058240561 ) ) ;
#6937=CARTESIAN_POINT ( 'NONE',  ( 4.037591185471442579, -77.70452850542925205, -5.718994135553947977 ) ) ;
#6938=CARTESIAN_POINT ( 'NONE',  ( -1.529537955723775156, -89.14547149457074227, -5.030887037049945221 ) ) ;
#6939=CARTESIAN_POINT ( 'NONE',  ( -1.529537955723671239, -70.35452850542925773, 5.030887037049979860 ) ) ;
#6940=CARTESIAN_POINT ( 'NONE',  ( 2.369498399071224615, -73.65452850542925489, 6.969112962950009482 ) ) ;
#6941=CARTESIAN_POINT ( 'NONE',  ( 0.09506052544077742139, -85.99547149457075079, -2.999999999999997780 ) ) ;
#6945=DIRECTION ( 'NONE',  ( 0.09506052544079829358, -0.9954714945707482388, 0.000000000000000000 ) ) ;
#6947=CARTESIAN_POINT ( 'NONE',  ( 4.312004677471078296, -91.95452850542926626, 3.009306630940844052 ) ) ;
#6948=CARTESIAN_POINT ( 'NONE',  ( -0.09506052544075405120, -96.49547149457075079, 2.999999999999997780 ) ) ;
#6949=CARTESIAN_POINT ( 'NONE',  ( -2.179377348189463603, -61.35452850542925773, 7.030887037049988741 ) ) ;
#6950=CARTESIAN_POINT ( 'NONE',  ( 6.013306294175077227, -67.54547149457074795, -4.245374608440741326 ) ) ;
#6951=CARTESIAN_POINT ( 'NONE',  ( 1.719659006605286367, -82.84547149457074511, -4.969112962950050338 ) ) ;
#6952=CARTESIAN_POINT ( 'NONE',  ( 2.823794231030040791, -80.40452850542925489, -1.017458915287783316 ) ) ;
#6956=FILL_AREA_STYLE_COLOUR ( '', #6244 ) ;
#6957=CARTESIAN_POINT ( 'NONE',  ( 3.015831842038231958, -58.80452850542925347, 3.989209796945429432 ) ) ;
#6958=CARTESIAN_POINT ( 'NONE',  ( 5.895805022753492608, -69.94547149457073942, 4.407101234057782868 ) ) ;
#6960=CARTESIAN_POINT ( 'NONE',  ( 4.479395550549687854, -97.00000000000000000, -3.869080787693377932 ) ) ;
#6961=CARTESIAN_POINT ( 'NONE',  ( 4.784657899331175912, -61.39547149457074227, -1.454677039711874009 ) ) ;
#6962=CARTESIAN_POINT ( 'NONE',  ( 0.09506052544073689825, -97.99547149457075079, -6.999999999999997335 ) ) ;
#6963=CARTESIAN_POINT ( 'NONE',  ( -0.09506052544084261924, -57.00452850542924921, -4.999999999999997335 ) ) ;
#6966=CARTESIAN_POINT ( 'NONE',  ( -5.257311121191324155, -69.75452850542926342, 0.09995255151729526277 ) ) ;
#6967=CARTESIAN_POINT ( 'NONE',  ( -4.191402346623055664, -96.19547149457075363, 5.607243785695398941 ) ) ;
#6974=CARTESIAN_POINT ( 'NONE',  ( -4.725907263620320542, -78.90452850542925489, 1.635492904037698647 ) ) ;
#6975=CARTESIAN_POINT ( 'NONE',  ( -4.312004677470991254, -90.04547149457071953, 3.009306630940933758 ) ) ;
#6976=CARTESIAN_POINT ( 'NONE',  ( 4.194503406049335581, -59.55452850542925347, -3.171033256558100977 ) ) ;
#6977=CARTESIAN_POINT ( 'NONE',  ( 1.686450176301635517, -72.79547149457074795, 2.482926158054096000 ) ) ;
#6979=CARTESIAN_POINT ( 'NONE',  ( -4.191402346623179120, -78.30452850542926058, -5.607243785695311900 ) ) ;
#6980=CARTESIAN_POINT ( 'NONE',  ( 2.862020680886600665, -87.79547149457074795, 4.100960146803977580 ) ) ;
#6982=CARTESIAN_POINT ( 'NONE',  ( -6.686770931921504513, -81.60452850542927195, -2.072711028461647675 ) ) ;
#6985=CARTESIAN_POINT ( 'NONE',  ( -1.069819614139473352, -87.34547149457073090, 2.969112962950044121 ) ) ;
#6991=CARTESIAN_POINT ( 'NONE',  ( 4.784657899331211439, -89.10452850542925773, 1.454677039711774533 ) ) ;
#6992=CARTESIAN_POINT ( 'NONE',  ( 0.09506052544077894795, -97.99547149457075079, -2.999999999999997780 ) ) ;
#6994=CARTESIAN_POINT ( 'NONE',  ( 2.369498399071222838, -61.65452850542925489, 6.969112962950009482 ) ) ;
#6995=CARTESIAN_POINT ( 'NONE',  ( -6.013306294175061240, -66.04547149457074795, 4.245374608440741326 ) ) ;
#6996=CARTESIAN_POINT ( 'NONE',  ( 1.529537955723796472, -84.64547149457074227, 5.030887037049945221 ) ) ;
#6997=CARTESIAN_POINT ( 'NONE',  ( 0.09506052544083844202, -73.50452850542924921, 2.999999999999997780 ) ) ;
#7001=CARTESIAN_POINT ( 'NONE',  ( -3.154386672714787565, -90.75452850542924921, 0.09995255151727280851 ) ) ;
#7002=CARTESIAN_POINT ( 'NONE',  ( -6.686770931921460992, -65.89547149457074227, 2.072711028461789784 ) ) ;
#7005=COLOUR_RGB ( '', 0.09019608, 0.27058824, 0.51372549) ;
#7006=CARTESIAN_POINT ( 'NONE',  ( -3.015831842038130262, -66.19547149457075363, 3.989209796945492048 ) ) ;
#7007=CARTESIAN_POINT ( 'NONE',  ( -4.784657899331160813, -59.89547149457074227, 1.454677039711874675 ) ) ;
#7008=CARTESIAN_POINT ( 'NONE',  ( -2.610703060766962569, -93.45452850542926626, -1.773238653441072232 ) ) ;
#7011=CARTESIAN_POINT ( 'NONE',  ( -1.529537955723671683, -67.35452850542925773, 5.030887037049979860 ) ) ;
#7012=CARTESIAN_POINT ( 'NONE',  ( 5.895805022753496161, -93.94547149457073942, 4.407101234057782868 ) ) ;
#7019=CARTESIAN_POINT ( 'NONE',  ( 4.725907263620340970, -80.40452850542925489, -1.635492904037697981 ) ) ;
#7020=CARTESIAN_POINT ( 'NONE',  ( -0.09506052544073352595, -90.49547149457073658, 4.999999999999997335 ) ) ;
#7021=CARTESIAN_POINT ( 'NONE',  ( -1.719659006605374962, -57.15452850542924779, -4.969112962950015699 ) ) ;
#7022=CARTESIAN_POINT ( 'NONE',  ( -2.823794231030040791, -74.59547149457071669, -1.017458915287723364 ) ) ;
#7023=CARTESIAN_POINT ( 'NONE',  ( -2.369498399071206851, -75.15452850542922647, -6.969112962950009482 ) ) ;
#7024=CARTESIAN_POINT ( 'NONE',  ( 4.784657899331179465, -88.39547149457074227, -1.454677039711874009 ) ) ;
#7026=CARTESIAN_POINT ( 'NONE',  ( 5.895805022753406455, -80.55452850542926058, -4.407101234057908989 ) ) ;
#7027=CARTESIAN_POINT ( 'NONE',  ( 1.840261337453221291, -85.69547149457073942, -2.371175808195584267 ) ) ;
#7030=CARTESIAN_POINT ( 'NONE',  ( -4.194503406049385319, -59.44547149457074653, -3.171033256558012159 ) ) ;
#7033=CARTESIAN_POINT ( 'NONE',  ( -4.725907263620320542, -78.90452850542925489, 1.635492904037698647 ) ) ;
#7034=CARTESIAN_POINT ( 'NONE',  ( -0.09506052544082121969, -60.00452850542925631, -2.999999999999997780 ) ) ;
#7036=CARTESIAN_POINT ( 'NONE',  ( 4.784657899331211439, -92.10452850542925773, 1.454677039711774533 ) ) ;
#7037=CARTESIAN_POINT ( 'NONE',  ( -2.369498399071057637, -72.34547149457073090, 6.969112962950058332 ) ) ;
#7038=CARTESIAN_POINT ( 'NONE',  ( -0.09506052544073428923, -84.49547149457075079, 4.999999999999997335 ) ) ;
#7039=CARTESIAN_POINT ( 'NONE',  ( -2.610703060766964345, -78.45452850542925205, -1.773238653441072232 ) ) ;
#7042=CARTESIAN_POINT ( 'NONE',  ( 1.840261337453272805, -91.80452850542926058, 2.371175808195547852 ) ) ;
#7043=CARTESIAN_POINT ( 'NONE',  ( -5.895805022753479285, -62.44547149457074653, -4.407101234057782868 ) ) ;
#7046=CARTESIAN_POINT ( 'NONE',  ( -4.725907263620355181, -62.59547149457074511, -1.635492904037597617 ) ) ;
#7047=CARTESIAN_POINT ( 'NONE',  ( 4.194503406049400418, -63.94547149457075363, 3.171033256558012159 ) ) ;
#7052=CARTESIAN_POINT ( 'NONE',  ( 2.862020680886513624, -71.70452850542925205, -4.100960146804039752 ) ) ;
#7053=CARTESIAN_POINT ( 'NONE',  ( 6.628020296210689111, -88.09547149457074511, 2.253526892787472757 ) ) ;
#7060=CARTESIAN_POINT ( 'NONE',  ( 4.725907263620340082, -74.40452850542925489, -1.635492904037697981 ) ) ;
#7061=CARTESIAN_POINT ( 'NONE',  ( 5.257311121191341918, -82.24547149457070816, 0.09995255151718437925 ) ) ;
#7063=CARTESIAN_POINT ( 'NONE',  ( -1.069819614139475350, -72.34547149457073090, 2.969112962950044121 ) ) ;
#7064=CARTESIAN_POINT ( 'NONE',  ( 4.037591185471441690, -65.70452850542925205, -5.718994135553947977 ) ) ;
#7065=CARTESIAN_POINT ( 'NONE',  ( 5.257311121191341918, -79.24547149457075079, 0.09995255151718437925 ) ) ;
#7066=CARTESIAN_POINT ( 'NONE',  ( 4.194503406049334693, -59.55452850542926058, -3.171033256558100089 ) ) ;
#7067=CARTESIAN_POINT ( 'NONE',  ( 2.862020680886516732, -95.70452850542926626, -4.100960146804039752 ) ) ;
#7068=CARTESIAN_POINT ( 'NONE',  ( 6.686770931921523164, -77.10452850542924352, 2.072711028461649008 ) ) ;
#7069=CARTESIAN_POINT ( 'NONE',  ( -0.8796985632579410463, -92.14547149457074227, -3.030887037049952326 ) ) ;
#7073=CARTESIAN_POINT ( 'NONE',  ( -3.015831842038131150, -60.19547149457074653, 3.989209796945492048 ) ) ;
#7074=CARTESIAN_POINT ( 'NONE',  ( -1.719659006605370744, -87.15452850542926910, -4.969112962950016588 ) ) ;
#7076=CARTESIAN_POINT ( 'NONE',  ( 3.015831842038233734, -76.80452850542926058, 3.989209796945429432 ) ) ;
#7077=CARTESIAN_POINT ( 'NONE',  ( -2.610703060766967010, -60.45452850542925916, -1.773238653441072232 ) ) ;
#7079=CARTESIAN_POINT ( 'NONE',  ( 4.784657899331210551, -83.10452850542927195, 1.454677039711774533 ) ) ;
#7080=CARTESIAN_POINT ( 'NONE',  ( -2.179377348189612817, -65.14547149457074227, -7.030887037049939003 ) ) ;
#7081=CARTESIAN_POINT ( 'NONE',  ( 4.784657899331179465, -88.39547149457074227, -1.454677039711874009 ) ) ;
#7082=CARTESIAN_POINT ( 'NONE',  ( -0.09506052544081970701, -72.00452850542926342, -2.999999999999997780 ) ) ;
#7085=CARTESIAN_POINT ( 'NONE',  ( 2.493201789345272701, -89.55452850542926058, -1.934965279058294518 ) ) ;
#7086=CARTESIAN_POINT ( 'NONE',  ( -6.628020296210670459, -59.59547149457074511, -2.253526892787471869 ) ) ;
#7088=CARTESIAN_POINT ( 'NONE',  ( -4.312004677470994807, -66.04547149457073374, 3.009306630940933314 ) ) ;
#7089=CARTESIAN_POINT ( 'NONE',  ( 1.529537955723794251, -63.64547149457074227, 5.030887037049945221 ) ) ;
#7092=CARTESIAN_POINT ( 'NONE',  ( 3.015831842038231958, -61.80452850542926058, 3.989209796945429432 ) ) ;
#7094=CARTESIAN_POINT ( 'NONE',  ( -6.013306294175058575, -90.04547149457074795, 4.245374608440741326 ) ) ;
#7097=CARTESIAN_POINT ( 'NONE',  ( 4.725907263620340082, -74.40452850542925489, -1.635492904037697981 ) ) ;
#7102=CARTESIAN_POINT ( 'NONE',  ( 4.784657899331178577, -82.39547149457074227, -1.454677039711874009 ) ) ;
#7103=CARTESIAN_POINT ( 'NONE',  ( 1.836369172260436056, -96.99999999999992895, -3.600965674691625207 ) ) ;
#7104=CARTESIAN_POINT ( 'NONE',  ( -1.686450176301617310, -74.29547149457074795, -2.482926158054096000 ) ) ;
#7105=CARTESIAN_POINT ( 'NONE',  ( -2.179377348189461827, -70.35452850542922931, 7.030887037049988741 ) ) ;
#7108=CARTESIAN_POINT ( 'NONE',  ( -4.725907263620353405, -80.59547149457074511, -1.635492904037597617 ) ) ;
#7109=CARTESIAN_POINT ( 'NONE',  ( -0.09506052544084224454, -60.00452850542925631, -4.999999999999997335 ) ) ;
#7111=CARTESIAN_POINT ( 'NONE',  ( 5.895805022753404678, -65.55452850542926058, -4.407101234057908989 ) ) ;
#7112=CARTESIAN_POINT ( 'NONE',  ( -0.09506052544075593858, -81.49547149457075079, 2.999999999999997780 ) ) ;
#7116=CARTESIAN_POINT ( 'NONE',  ( -3.015831842038213750, -84.30452850542926058, -3.989209796945429432 ) ) ;
#7118=CARTESIAN_POINT ( 'NONE',  ( -1.719659006605372076, -78.15452850542926910, -4.969112962950015699 ) ) ;
#7119=CARTESIAN_POINT ( 'NONE',  ( -3.154386672714791118, -63.75452850542926342, 0.09995255151727280851 ) ) ;
#7121=CARTESIAN_POINT ( 'NONE',  ( 4.194503406049338246, -83.55452850542921794, -3.171033256558100089 ) ) ;
#7122=CARTESIAN_POINT ( 'NONE',  ( 6.628020296210686446, -61.09547149457074511, 2.253526892787472757 ) ) ;
#7124=CARTESIAN_POINT ( 'NONE',  ( -1.529537955723776710, -80.14547149457072805, -5.030887037049945221 ) ) ;
#7125=CARTESIAN_POINT ( 'NONE',  ( 2.493201789345271369, -77.55452850542926058, -1.934965279058294518 ) ) ;
#7129=CARTESIAN_POINT ( 'NONE',  ( -1.069819614139537522, -84.15452850542925489, -2.969112962950023249 ) ) ;
#7131=CARTESIAN_POINT ( 'NONE',  ( 4.191402346623076980, -64.69547149457073942, -5.607243785695398941 ) ) ;
#7133=CARTESIAN_POINT ( 'NONE',  ( 0.09506052544086007750, -76.50452850542924921, 4.999999999999997335 ) ) ;
#7134=CARTESIAN_POINT ( 'NONE',  ( -2.179377348189609265, -86.14547149457072805, -7.030887037049939003 ) ) ;
#7136=MANIFOLD_SOLID_BREP ( 'Cavity1', #6261 ) ;
#7139=CARTESIAN_POINT ( 'NONE',  ( -4.725907263620323207, -60.90452850542925489, 1.635492904037698647 ) ) ;
#7141=CARTESIAN_POINT ( 'NONE',  ( 5.895805022753496161, -87.94547149457073942, 4.407101234057782868 ) ) ;
#7143=CARTESIAN_POINT ( 'NONE',  ( -1.719659006605372964, -72.15452850542921226, -4.969112962950016588 ) ) ;
#7148=CARTESIAN_POINT ( 'NONE',  ( -3.015831842038128485, -81.19547149457073942, 3.989209796945492048 ) ) ;
#7149=CARTESIAN_POINT ( 'NONE',  ( 4.241803400547042635, -96.99999999999998579, 2.098537186797552412 ) ) ;
#7150=CARTESIAN_POINT ( 'NONE',  ( -2.493201789345293129, -59.44547149457074653, -1.934965279058240561 ) ) ;
#7151=CARTESIAN_POINT ( 'NONE',  ( -7.360235569667858968, -66.75452850542926342, 0.09995255151731782806 ) ) ;
#7153=CARTESIAN_POINT ( 'NONE',  ( -1.719659006605264828, -81.34547149457074511, 4.969112962950051227 ) ) ;
#7154=CARTESIAN_POINT ( 'NONE',  ( -3.015831842038217303, -57.30452850542925347, -3.989209796945429432 ) ) ;
#7155=CARTESIAN_POINT ( 'NONE',  ( -4.312004677471056091, -90.45452850542926626, -3.009306630940844052 ) ) ;
#7156=CARTESIAN_POINT ( 'NONE',  ( -6.628020296210622497, -66.90452850542925489, 2.253526892787613978 ) ) ;
#7157=CARTESIAN_POINT ( 'NONE',  ( -2.823794231030040791, -74.59547149457071669, -1.017458915287723364 ) ) ;
#7160=CARTESIAN_POINT ( 'NONE',  ( -0.09506052544083808120, -93.00452850542926342, -4.999999999999997335 ) ) ;
#7161=CARTESIAN_POINT ( 'NONE',  ( -4.725907263620320542, -84.90452850542925489, 1.635492904037698647 ) ) ;
#7163=CARTESIAN_POINT ( 'NONE',  ( 1.529537955723691223, -83.85452850542927195, -5.030887037049978971 ) ) ;
#7164=CARTESIAN_POINT ( 'NONE',  ( -2.610703060766923933, -93.04547149457074795, 1.773238653441125745 ) ) ;
#7166=CARTESIAN_POINT ( 'NONE',  ( 1.529537955723691001, -83.85452850542927195, -5.030887037049978971 ) ) ;
#7167=CARTESIAN_POINT ( 'NONE',  ( -2.369498399071059414, -60.34547149457074511, 6.969112962950058332 ) ) ;
#7168=CARTESIAN_POINT ( 'NONE',  ( -3.154386672714791118, -63.75452850542926342, 0.09995255151727280851 ) ) ;
#7171=CARTESIAN_POINT ( 'NONE',  ( 0.09506052544084069023, -91.50452850542926342, 2.999999999999997780 ) ) ;
#7172=CARTESIAN_POINT ( 'NONE',  ( 6.628020296210686446, -61.09547149457074511, 2.253526892787472757 ) ) ;
#7174=CARTESIAN_POINT ( 'NONE',  ( -4.194503406049316929, -76.05452850542926058, 3.171033256558100533 ) ) ;
#7175=CARTESIAN_POINT ( 'NONE',  ( 6.686770931921479644, -88.39547149457074227, -2.072711028461788896 ) ) ;
#7179=CARTESIAN_POINT ( 'NONE',  ( 2.493201789345309116, -69.94547149457073942, 1.934965279058241006 ) ) ;
#7182=CARTESIAN_POINT ( 'NONE',  ( 0.09506052544073539945, -85.99547149457075079, -6.999999999999997335 ) ) ;
#7185=CARTESIAN_POINT ( 'NONE',  ( 3.015831842038234178, -79.80452850542926058, 3.989209796945429432 ) ) ;
#7191=CARTESIAN_POINT ( 'NONE',  ( -4.784657899331157260, -83.89547149457074227, 1.454677039711874675 ) ) ;
#7193=CARTESIAN_POINT ( 'NONE',  ( 0.09506052544077400746, -58.99547149457073658, -2.999999999999997780 ) ) ;
#7194=CARTESIAN_POINT ( 'NONE',  ( 6.628020296210639373, -71.40452850542924068, -2.253526892787612645 ) ) ;
#7196=CARTESIAN_POINT ( 'NONE',  ( 3.015831842038149357, -79.69547149457075363, -3.989209796945492048 ) ) ;
#7198=CARTESIAN_POINT ( 'NONE',  ( -5.257311121191323267, -84.75452850542923500, 0.09995255151729526277 ) ) ;
#7199=CARTESIAN_POINT ( 'NONE',  ( -0.09506052544086217304, -69.00452850542926342, -6.999999999999997335 ) ) ;
#7201=CARTESIAN_POINT ( 'NONE',  ( 1.840261337453220847, -82.69547149457073942, -2.371175808195584267 ) ) ;
#7205=CARTESIAN_POINT ( 'NONE',  ( -0.09506052544083921918, -84.00452850542926342, -4.999999999999997335 ) ) ;
#7207=CARTESIAN_POINT ( 'NONE',  ( 2.862020680886514512, -77.70452850542926626, -4.100960146804039752 ) ) ;
#7208=CARTESIAN_POINT ( 'NONE',  ( 2.823794231030061663, -91.09547149457074511, 1.017458915287723809 ) ) ;
#7210=CARTESIAN_POINT ( 'NONE',  ( -1.719659006605371188, -84.15452850542925489, -4.969112962950016588 ) ) ;
#7211=CARTESIAN_POINT ( 'NONE',  ( 7.360235569667880284, -95.25452850542926342, -0.09995255151731691212 ) ) ;
#7213=CARTESIAN_POINT ( 'NONE',  ( -1.686450176301566684, -70.20452850542925205, 2.482926158054133303 ) ) ;
#7216=CARTESIAN_POINT ( 'NONE',  ( -3.154386672714789341, -78.75452850542926342, 0.09995255151727280851 ) ) ;
#7217=CARTESIAN_POINT ( 'NONE',  ( 5.895805022753407343, -92.55452850542926058, -4.407101234057908989 ) ) ;
#7219=CARTESIAN_POINT ( 'NONE',  ( 2.369498399071078953, -88.84547149457073090, -6.969112962950057444 ) ) ;
#7222=CARTESIAN_POINT ( 'NONE',  ( 0.09506052544077554789, -70.99547149457075079, -2.999999999999997780 ) ) ;
#7224=CARTESIAN_POINT ( 'NONE',  ( -4.784657899331191899, -63.60452850542925063, -1.454677039711773867 ) ) ;
#7226=CARTESIAN_POINT ( 'NONE',  ( 4.725907263620340082, -65.40452850542925489, -1.635492904037697981 ) ) ;
#7227=CARTESIAN_POINT ( 'NONE',  ( 0.09506052544073462229, -79.99547149457075079, -6.999999999999997335 ) ) ;
#7230=CARTESIAN_POINT ( 'NONE',  ( 0.09506052544085971667, -73.50452850542924921, 4.999999999999997335 ) ) ;
#7232=CARTESIAN_POINT ( 'NONE',  ( -4.784657899331158148, -77.89547149457074227, 1.454677039711874675 ) ) ;
#7234=CARTESIAN_POINT ( 'NONE',  ( -3.154386672714792006, -62.74547149457073658, -0.09995255151720625064 ) ) ;
#7235=CARTESIAN_POINT ( 'NONE',  ( 4.191402346623196884, -67.80452850542926058, 5.607243785695311900 ) ) ;
#7237=CARTESIAN_POINT ( 'NONE',  ( -0.09506052544073503863, -78.49547149457073658, 4.999999999999997335 ) ) ;
#7239=CARTESIAN_POINT ( 'NONE',  ( -1.529537955723669684, -82.35452850542922931, 5.030887037049979860 ) ) ;
#7240=CARTESIAN_POINT ( 'NONE',  ( 6.628020296210639373, -65.40452850542925489, -2.253526892787612645 ) ) ;
#7241=CARTESIAN_POINT ( 'NONE',  ( 3.154386672714809770, -82.24547149457073658, 0.09995255151720662534 ) ) ;
#7245=CARTESIAN_POINT ( 'NONE',  ( 4.725907263620341858, -89.40452850542926910, -1.635492904037697981 ) ) ;
#7247=CARTESIAN_POINT ( 'NONE',  ( -2.862020680886494972, -73.20452850542925205, 4.100960146804039752 ) ) ;
#7248=CARTESIAN_POINT ( 'NONE',  ( 3.154386672714811102, -94.24547149457075079, 0.09995255151720662534 ) ) ;
#7249=CARTESIAN_POINT ( 'NONE',  ( 4.312004677471078296, -88.95452850542922363, 3.009306630940844496 ) ) ;
#7250=CARTESIAN_POINT ( 'NONE',  ( 6.628020296210643814, -95.40452850542926910, -2.253526892787612645 ) ) ;
#7251=CARTESIAN_POINT ( 'NONE',  ( -2.882544866740878842, -66.60452850542924352, -0.8366430509618996147 ) ) ;
#7254=CARTESIAN_POINT ( 'NONE',  ( 1.840261337453271251, -79.80452850542926058, 2.371175808195547852 ) ) ;
#7255=CARTESIAN_POINT ( 'NONE',  ( -5.895805022753386027, -85.05452850542926058, 4.407101234057909878 ) ) ;
#7257=CARTESIAN_POINT ( 'NONE',  ( -4.037591185471542943, -92.29547149457074795, -5.718994135553860936 ) ) ;
#7260=CARTESIAN_POINT ( 'NONE',  ( 2.882544866740876621, -70.39547149457072805, -0.8366430509619593447 ) ) ;
#7264=CARTESIAN_POINT ( 'NONE',  ( 4.194503406049335581, -71.55452850542926058, -3.171033256558100089 ) ) ;
#7265=CARTESIAN_POINT ( 'NONE',  ( 4.191402346623079644, -82.69547149457073942, -5.607243785695398941 ) ) ;
#7268=CARTESIAN_POINT ( 'NONE',  ( 4.725907263620340082, -77.40452850542925489, -1.635492904037697981 ) ) ;
#7272=CARTESIAN_POINT ( 'NONE',  ( 4.194503406049401306, -69.94547149457071100, 3.171033256558012159 ) ) ;
#7274=CARTESIAN_POINT ( 'NONE',  ( 1.069819614139492669, -64.84547149457071669, -2.969112962950042789 ) ) ;
#7275=CARTESIAN_POINT ( 'NONE',  ( -6.686770931921507177, -63.60452850542924352, -2.072711028461647675 ) ) ;
#7278=CARTESIAN_POINT ( 'NONE',  ( -4.725907263620320542, -81.90452850542925489, 1.635492904037698647 ) ) ;
#7279=CARTESIAN_POINT ( 'NONE',  ( 2.179377348189480035, -62.85452850542923642, -7.030887037049986077 ) ) ;
#7280=CARTESIAN_POINT ( 'NONE',  ( -1.840261337453200197, -78.19547149457073942, 2.371175808195584267 ) ) ;
#7283=CARTESIAN_POINT ( 'NONE',  ( 5.257311121191343695, -95.25452850542924921, -0.09995255151729465215 ) ) ;
#7284=CARTESIAN_POINT ( 'NONE',  ( 5.257311121191341918, -77.25452850542926342, -0.09995255151729465215 ) ) ;
#7286=CARTESIAN_POINT ( 'NONE',  ( 4.725907263620340082, -68.40452850542925489, -1.635492904037697981 ) ) ;
#7287=CARTESIAN_POINT ( 'NONE',  ( -1.686450176301615311, -89.29547149457074795, -2.482926158054096000 ) ) ;
#7288=CARTESIAN_POINT ( 'NONE',  ( 2.823794231030057666, -61.09547149457074511, 1.017458915287723809 ) ) ;
#7289=CARTESIAN_POINT ( 'NONE',  ( -6.013306294175149169, -93.45452850542926626, -4.245374608440613429 ) ) ;
#7290=CARTESIAN_POINT ( 'NONE',  ( 0.8796985632578976366, -65.85452850542924352, -3.030887037049972310 ) ) ;
#7296=CARTESIAN_POINT ( 'NONE',  ( -2.882544866740876621, -81.60452850542927195, -0.8366430509618996147 ) ) ;
#7297=CARTESIAN_POINT ( 'NONE',  ( 6.628020296210642037, -86.40452850542926910, -2.253526892787612645 ) ) ;
#7298=CARTESIAN_POINT ( 'NONE',  ( -6.628020296210665130, -92.59547149457074511, -2.253526892787471869 ) ) ;
#7301=CARTESIAN_POINT ( 'NONE',  ( 2.493201789345309560, -72.94547149457073942, 1.934965279058241006 ) ) ;
#7306=CARTESIAN_POINT ( 'NONE',  ( -1.529537955723671683, -67.35452850542925773, 5.030887037049979860 ) ) ;
#7307=CARTESIAN_POINT ( 'NONE',  ( 6.628020296210687334, -76.09547149457073090, 2.253526892787472757 ) ) ;
#7309=CARTESIAN_POINT ( 'NONE',  ( 4.725907263620340082, -68.40452850542925489, -1.635492904037697981 ) ) ;
#7311=CARTESIAN_POINT ( 'NONE',  ( 2.862020680886598889, -69.79547149457074795, 4.100960146803977580 ) ) ;
#7313=CARTESIAN_POINT ( 'NONE',  ( -1.069819614139475794, -66.34547149457073090, 2.969112962950044121 ) ) ;
#7315=CARTESIAN_POINT ( 'NONE',  ( -4.037591185471424815, -58.20452850542925916, 5.718994135553947977 ) ) ;
#7319=CARTESIAN_POINT ( 'NONE',  ( -1.719659006605371632, -81.15452850542922647, -4.969112962950016588 ) ) ;
#7326=CARTESIAN_POINT ( 'NONE',  ( -1.529537955723668796, -85.35452850542924352, 5.030887037049979860 ) ) ;
#7327=CARTESIAN_POINT ( 'NONE',  ( -4.312004677471057867, -75.45452850542925205, -3.009306630940844052 ) ) ;
#7329=CARTESIAN_POINT ( 'NONE',  ( -3.015831842038215971, -69.30452850542926058, -3.989209796945429432 ) ) ;
#7330=CARTESIAN_POINT ( 'NONE',  ( -2.493201789345289132, -89.44547149457073942, -1.934965279058240561 ) ) ;
#7331=CARTESIAN_POINT ( 'NONE',  ( 1.529537955723797138, -93.64547149457074227, 5.030887037049945221 ) ) ;
#7332=CARTESIAN_POINT ( 'NONE',  ( 4.784657899331210551, -80.10452850542925773, 1.454677039711774533 ) ) ;
#7333=CARTESIAN_POINT ( 'NONE',  ( -6.686770931921503625, -90.60452850542925773, -2.072711028461647675 ) ) ;
#7334=CARTESIAN_POINT ( 'NONE',  ( 3.154386672714806217, -59.25452850542926342, -0.09995255151727241993 ) ) ;
#7339=CARTESIAN_POINT ( 'NONE',  ( -0.09506052544081930455, -75.00452850542926342, -2.999999999999997780 ) ) ;
#7340=CARTESIAN_POINT ( 'NONE',  ( -5.895805022753383362, -88.05452850542926058, 4.407101234057909878 ) ) ;
#7341=CARTESIAN_POINT ( 'NONE',  ( 2.369498399071077177, -76.84547149457073090, -6.969112962950057444 ) ) ;
#7345=CARTESIAN_POINT ( 'NONE',  ( 2.493201789345308228, -63.94547149457074653, 1.934965279058241006 ) ) ;
#7348=CARTESIAN_POINT ( 'NONE',  ( -3.015831842038216415, -66.30452850542926058, -3.989209796945429432 ) ) ;
#7349=CARTESIAN_POINT ( 'NONE',  ( 5.895805022753496161, -78.94547149457073942, 4.407101234057782868 ) ) ;
#7350=SURFACE_STYLE_USAGE ( .BOTH. , #4774 ) ;
#7352=CARTESIAN_POINT ( 'NONE',  ( -3.015831842038128929, -78.19547149457075363, 3.989209796945492048 ) ) ;
#7353=CARTESIAN_POINT ( 'NONE',  ( -3.015831842038216415, -66.30452850542926058, -3.989209796945429432 ) ) ;
#7355=CARTESIAN_POINT ( 'NONE',  ( 4.312004677471011682, -67.54547149457074795, -3.009306630940933314 ) ) ;
#7357=CARTESIAN_POINT ( 'NONE',  ( 0.09506052544075753452, -94.99547149457073658, -4.999999999999997335 ) ) ;
#7358=CARTESIAN_POINT ( 'NONE',  ( 2.369498399071222838, -61.65452850542925489, 6.969112962950009482 ) ) ;
#7362=CARTESIAN_POINT ( 'NONE',  ( -4.784657899331190123, -84.60452850542927195, -1.454677039711773867 ) ) ;
#7363=CARTESIAN_POINT ( 'NONE',  ( 0.09506052544086084077, -82.50452850542926342, 4.999999999999997335 ) ) ;
#7366=CARTESIAN_POINT ( 'NONE',  ( 4.194503406049336469, -68.55452850542926058, -3.171033256558100977 ) ) ;
#7367=CARTESIAN_POINT ( 'NONE',  ( -3.154386672714789341, -83.74547149457075079, -0.09995255151720625064 ) ) ;
#7368=CARTESIAN_POINT ( 'NONE',  ( 2.862020680886601554, -93.79547149457074795, 4.100960146803977580 ) ) ;
#7369=CARTESIAN_POINT ( 'NONE',  ( 3.015831842038234178, -79.80452850542926058, 3.989209796945429432 ) ) ;
#7370=CARTESIAN_POINT ( 'NONE',  ( 2.179377348189483143, -89.85452850542924352, -7.030887037049986077 ) ) ;
#7372=CARTESIAN_POINT ( 'NONE',  ( 0.09506052544077857325, -94.99547149457075079, -2.999999999999997780 ) ) ;
#7377=CARTESIAN_POINT ( 'NONE',  ( -0.8796985632578788739, -79.35452850542927195, 3.030887037049973198 ) ) ;
#7379=CARTESIAN_POINT ( 'NONE',  ( -7.360235569667856304, -90.75452850542924921, 0.09995255151731782806 ) ) ;
#7380=CARTESIAN_POINT ( 'NONE',  ( -5.895805022753477509, -77.44547149457073942, -4.407101234057782868 ) ) ;
#7383=CARTESIAN_POINT ( 'NONE',  ( -1.840261337453251267, -81.30452850542926058, -2.371175808195547852 ) ) ;
#7390=CARTESIAN_POINT ( 'NONE',  ( -1.719659006605373408, -69.15452850542924068, -4.969112962950016588 ) ) ;
#7392=CARTESIAN_POINT ( 'NONE',  ( 6.628020296210689111, -82.09547149457075932, 2.253526892787472757 ) ) ;
#7394=CARTESIAN_POINT ( 'NONE',  ( 4.725907263620372056, -73.09547149457074511, 1.635492904037598283 ) ) ;
#7395=CARTESIAN_POINT ( 'NONE',  ( -4.194503406049384431, -68.44547149457073942, -3.171033256558012159 ) ) ;
#7397=CARTESIAN_POINT ( 'NONE',  ( -0.09506052544084186984, -63.00452850542925631, -4.999999999999997335 ) ) ;
#7402=CARTESIAN_POINT ( 'NONE',  ( -4.725907263620354293, -71.59547149457074511, -1.635492904037597617 ) ) ;
#7405=CARTESIAN_POINT ( 'NONE',  ( -6.013306294175155386, -57.45452850542925916, -4.245374608440613429 ) ) ;
#7411=CARTESIAN_POINT ( 'NONE',  ( -3.015831842038213750, -90.30452850542926058, -3.989209796945429432 ) ) ;
#7412=CARTESIAN_POINT ( 'NONE',  ( -3.015831842038214194, -81.30452850542926058, -3.989209796945429432 ) ) ;
#7414=CARTESIAN_POINT ( 'NONE',  ( -1.529537955723671239, -70.35452850542927195, 5.030887037049979860 ) ) ;
#7415=CARTESIAN_POINT ( 'NONE',  ( -1.686450176301616866, -77.29547149457074795, -2.482926158054096000 ) ) ;
#7417=CARTESIAN_POINT ( 'NONE',  ( 1.686450176301633963, -60.79547149457074084, 2.482926158054096000 ) ) ;
#7418=CARTESIAN_POINT ( 'NONE',  ( -4.312004677471058756, -66.45452850542925205, -3.009306630940844052 ) ) ;
#7419=CARTESIAN_POINT ( 'NONE',  ( 0.09506052544088290646, -88.50452850542926342, 6.999999999999997335 ) ) ;
#7420=CARTESIAN_POINT ( 'NONE',  ( 2.610703060766947914, -94.54547149457073374, -1.773238653441125523 ) ) ;
#7425=CARTESIAN_POINT ( 'NONE',  ( 2.493201789345270480, -68.55452850542926058, -1.934965279058294518 ) ) ;
#7426=CARTESIAN_POINT ( 'NONE',  ( -0.09506052544071380561, -78.49547149457075079, 6.999999999999997335 ) ) ;
#7429=CARTESIAN_POINT ( 'NONE',  ( 3.154386672714809770, -83.25452850542926342, -0.09995255151727241993 ) ) ;
#7432=CARTESIAN_POINT ( 'NONE',  ( -0.09506052544084224454, -60.00452850542925631, -4.999999999999997335 ) ) ;
#7433=CARTESIAN_POINT ( 'NONE',  ( -4.037591185471545607, -71.29547149457074795, -5.718994135553860936 ) ) ;
#7436=CARTESIAN_POINT ( 'NONE',  ( 4.194503406049403083, -78.94547149457073942, 3.171033256558012159 ) ) ;
#7437=CARTESIAN_POINT ( 'NONE',  ( 4.194503406049401306, -69.94547149457071100, 3.171033256558012159 ) ) ;
#7438=CARTESIAN_POINT ( 'NONE',  ( -2.862020680886495860, -64.20452850542926626, 4.100960146804039752 ) ) ;
#7442=CARTESIAN_POINT ( 'NONE',  ( -0.09506052544073617661, -69.49547149457075079, 4.999999999999997335 ) ) ;
#7444=CARTESIAN_POINT ( 'NONE',  ( 4.194503406049340022, -95.55452850542921794, -3.171033256558100089 ) ) ;
#7445=ORIENTED_EDGE ( 'NONE', *, *, #5622, .T. ) ;
#7449=CARTESIAN_POINT ( 'NONE',  ( -4.194503406049316041, -85.05452850542926058, 3.171033256558100533 ) ) ;
#7451=CARTESIAN_POINT ( 'NONE',  ( -1.719659006605372076, -75.15452850542925489, -4.969112962950016588 ) ) ;
#7452=CARTESIAN_POINT ( 'NONE',  ( -4.312004677471060532, -57.45452850542925916, -3.009306630940843608 ) ) ;
#7453=CARTESIAN_POINT ( 'NONE',  ( -2.493201789345290464, -80.44547149457073942, -1.934965279058240561 ) ) ;
#7454=CARTESIAN_POINT ( 'NONE',  ( -3.015831842038126709, -96.19547149457075363, 3.989209796945492048 ) ) ;
#7455=CARTESIAN_POINT ( 'NONE',  ( 2.862020680886513624, -71.70452850542925205, -4.100960146804039752 ) ) ;
#7456=CARTESIAN_POINT ( 'NONE',  ( -2.179377348189460051, -85.35452850542924352, 7.030887037049988741 ) ) ;
#7459=CARTESIAN_POINT ( 'NONE',  ( -2.882544866740855749, -95.89547149457075648, 0.8366430509619596778 ) ) ;
#7466=CARTESIAN_POINT ( 'NONE',  ( -3.154386672714790674, -72.75452850542926342, 0.09995255151727280851 ) ) ;
#7468=CARTESIAN_POINT ( 'NONE',  ( 4.037591185471562483, -75.79547149457074795, 5.718994135553860936 ) ) ;
#7469=CARTESIAN_POINT ( 'NONE',  ( -4.194503406049314265, -94.05452850542926058, 3.171033256558100533 ) ) ;
#7471=CARTESIAN_POINT ( 'NONE',  ( -1.686450176301564907, -82.20452850542925205, 2.482926158054133303 ) ) ;
#7475=CARTESIAN_POINT ( 'NONE',  ( -4.784657899331191899, -60.60452850542925773, -1.454677039711773867 ) ) ;
#7476=CARTESIAN_POINT ( 'NONE',  ( 2.369498399071077177, -73.84547149457073090, -6.969112962950057444 ) ) ;
#7479=CARTESIAN_POINT ( 'NONE',  ( -1.529537955723777820, -71.14547149457072805, -5.030887037049945221 ) ) ;
#7480=CARTESIAN_POINT ( 'NONE',  ( -1.719659006605267049, -66.34547149457073090, 4.969112962950051227 ) ) ;
#7481=CARTESIAN_POINT ( 'NONE',  ( -1.529537955723671905, -61.35452850542925773, 5.030887037049979860 ) ) ;
#7483=CARTESIAN_POINT ( 'NONE',  ( 5.257311121191341918, -64.24547149457073658, 0.09995255151718437925 ) ) ;
#7485=CARTESIAN_POINT ( 'NONE',  ( -4.725907263620318766, -93.90452850542925489, 1.635492904037698647 ) ) ;
#7491=CARTESIAN_POINT ( 'NONE',  ( -2.862020680886492308, -91.20452850542926626, 4.100960146804039752 ) ) ;
#7492=CARTESIAN_POINT ( 'NONE',  ( -4.725907263620351628, -89.59547149457074511, -1.635492904037597617 ) ) ;
#7493=CARTESIAN_POINT ( 'NONE',  ( 0.09506052544085819012, -61.50452850542925631, 4.999999999999997335 ) ) ;
#7494=CARTESIAN_POINT ( 'NONE',  ( 1.686450176301636850, -81.79547149457074795, 2.482926158054096000 ) ) ;
#7495=CARTESIAN_POINT ( 'NONE',  ( 1.719659006605287033, -91.84547149457074511, -4.969112962950050338 ) ) ;
#7497=CARTESIAN_POINT ( 'NONE',  ( 4.312004677471074743, -70.95452850542925205, 3.009306630940844496 ) ) ;
#7498=CARTESIAN_POINT ( 'NONE',  ( 6.628020296210642037, -92.40452850542925489, -2.253526892787612645 ) ) ;
#7499=CARTESIAN_POINT ( 'NONE',  ( -3.154386672714792006, -60.75452850542924921, 0.09995255151727280851 ) ) ;
#7504=CARTESIAN_POINT ( 'NONE',  ( 2.862020680886515400, -86.70452850542925205, -4.100960146804039752 ) ) ;
#7505=CARTESIAN_POINT ( 'NONE',  ( -3.154386672714790674, -69.75452850542926342, 0.09995255151727280851 ) ) ;
#7506=CARTESIAN_POINT ( 'NONE',  ( -4.191402346623058328, -75.19547149457073942, 5.607243785695398941 ) ) ;
#7508=CARTESIAN_POINT ( 'NONE',  ( -4.194503406049380878, -95.44547149457073942, -3.171033256558012159 ) ) ;
#7509=CARTESIAN_POINT ( 'NONE',  ( -2.610703060766962569, -87.45452850542925205, -1.773238653441072232 ) ) ;
#7513=CARTESIAN_POINT ( 'NONE',  ( -1.719659006605374962, -57.15452850542924068, -4.969112962950016588 ) ) ;
#7514=CARTESIAN_POINT ( 'NONE',  ( 6.628020296210686446, -67.09547149457073090, 2.253526892787472757 ) ) ;
#7516=CARTESIAN_POINT ( 'NONE',  ( 4.312004677471010794, -70.54547149457074795, -3.009306630940932425 ) ) ;
#7517=CARTESIAN_POINT ( 'NONE',  ( -1.719659006605266827, -69.34547149457074511, 4.969112962950051227 ) ) ;
#7518=CARTESIAN_POINT ( 'NONE',  ( -3.154386672714787565, -93.75452850542926342, 0.09995255151727280851 ) ) ;
#7521=CARTESIAN_POINT ( 'NONE',  ( 1.719659006605389173, -64.65452850542925489, 4.969112962950016588 ) ) ;
#7522=CARTESIAN_POINT ( 'NONE',  ( -2.862020680886582458, -59.29547149457074084, -4.100960146803977580 ) ) ;
#7530=CARTESIAN_POINT ( 'NONE',  ( 1.529537955723690112, -77.85452850542922931, -5.030887037049978971 ) ) ;
#7531=CARTESIAN_POINT ( 'NONE',  ( 1.529537955723796916, -90.64547149457075648, 5.030887037049945221 ) ) ;
#7532=CARTESIAN_POINT ( 'NONE',  ( -5.257311121191325043, -63.75452850542925631, 0.09995255151729529053 ) ) ;
#7533=CARTESIAN_POINT ( 'NONE',  ( 3.154386672714809770, -85.24547149457075079, 0.09995255151720662534 ) ) ;
#7534=CARTESIAN_POINT ( 'NONE',  ( 2.179377348189482699, -80.85452850542925773, -7.030887037049986077 ) ) ;
#7535=CARTESIAN_POINT ( 'NONE',  ( -1.719659006605264384, -84.34547149457071669, 4.969112962950051227 ) ) ;
#7536=CARTESIAN_POINT ( 'NONE',  ( 2.862020680886512736, -65.70452850542925205, -4.100960146804039752 ) ) ;
#7538=CARTESIAN_POINT ( 'NONE',  ( -6.628020296210620721, -81.90452850542925489, 2.253526892787613978 ) ) ;
#7539=CARTESIAN_POINT ( 'NONE',  ( 2.882544866740878398, -85.39547149457074227, -0.8366430509619593447 ) ) ;
#7543=CARTESIAN_POINT ( 'NONE',  ( -4.784657899331189235, -90.60452850542925773, -1.454677039711773867 ) ) ;
#7544=CARTESIAN_POINT ( 'NONE',  ( -1.686450176301567350, -64.20452850542925205, 2.482926158054133303 ) ) ;
#7545=CARTESIAN_POINT ( 'NONE',  ( -4.194503406049314265, -94.05452850542926058, 3.171033256558100533 ) ) ;
#7546=CARTESIAN_POINT ( 'NONE',  ( 7.360235569667877620, -70.24547149457075079, 0.09995255151716216091 ) ) ;
#7547=CARTESIAN_POINT ( 'NONE',  ( 4.725907263620341858, -92.40452850542925489, -1.635492904037697981 ) ) ;
#7548=CARTESIAN_POINT ( 'NONE',  ( -4.194503406049382654, -86.44547149457072521, -3.171033256558012159 ) ) ;
#7549=CARTESIAN_POINT ( 'NONE',  ( -0.09506052544081818045, -84.00452850542926342, -2.999999999999997780 ) ) ;
#7553=CARTESIAN_POINT ( 'NONE',  ( 5.257311121191341918, -62.25452850542924921, -0.09995255151729465215 ) ) ;
#7554=CARTESIAN_POINT ( 'NONE',  ( -0.09506052544071491583, -69.49547149457075079, 6.999999999999997335 ) ) ;
#7557=CARTESIAN_POINT ( 'NONE',  ( -5.257311121191325043, -65.74547149457075079, -0.09995255151718372699 ) ) ;
#7558=CARTESIAN_POINT ( 'NONE',  ( 3.015831842038147137, -64.69547149457075363, -3.989209796945492048 ) ) ;
#7559=CARTESIAN_POINT ( 'NONE',  ( -3.015831842038217303, -57.30452850542925347, -3.989209796945429432 ) ) ;
#7561=CARTESIAN_POINT ( 'NONE',  ( -2.862020680886495416, -67.20452850542925205, 4.100960146804039752 ) ) ;
#7562=CARTESIAN_POINT ( 'NONE',  ( -2.862020680886582014, -62.29547149457074084, -4.100960146803977580 ) ) ;
#7567=CARTESIAN_POINT ( 'NONE',  ( -4.312004677471057867, -75.45452850542925205, -3.009306630940844052 ) ) ;
#7568=CARTESIAN_POINT ( 'NONE',  ( -1.719659006605264162, -90.34547149457074511, 4.969112962950051227 ) ) ;
#7569=CARTESIAN_POINT ( 'NONE',  ( -0.09506052544084148126, -66.00452850542926342, -4.999999999999997335 ) ) ;
#7570=CARTESIAN_POINT ( 'NONE',  ( -2.610703060766926598, -72.04547149457074795, 1.773238653441125745 ) ) ;
#7571=CARTESIAN_POINT ( 'NONE',  ( -0.09506052544086102118, -78.00452850542926342, -6.999999999999997335 ) ) ;
#7572=CARTESIAN_POINT ( 'NONE',  ( -1.719659006605264384, -87.34547149457074511, 4.969112962950051227 ) ) ;
#7573=CARTESIAN_POINT ( 'NONE',  ( -2.862020680886495416, -67.20452850542925205, 4.100960146804039752 ) ) ;
#7574=CARTESIAN_POINT ( 'NONE',  ( 4.037591185471442579, -74.70452850542925205, -5.718994135553947977 ) ) ;
#7575=CARTESIAN_POINT ( 'NONE',  ( -0.8796985632579418235, -86.14547149457072805, -3.030887037049952326 ) ) ;
#7579=FACE_OUTER_BOUND ( 'NONE', #5487, .T. ) ;
#7581=CARTESIAN_POINT ( 'NONE',  ( -4.312004677471056091, -87.45452850542925205, -3.009306630940843608 ) ) ;
#7582=CARTESIAN_POINT ( 'NONE',  ( 2.610703060766981665, -58.95452850542925916, 1.773238653441072232 ) ) ;
#7583=CARTESIAN_POINT ( 'NONE',  ( 3.015831842038236399, -94.80452850542924637, 3.989209796945429432 ) ) ;
#7586=CARTESIAN_POINT ( 'NONE',  ( 6.686770931921476979, -67.39547149457074227, -2.072711028461788896 ) ) ;
#7588=CARTESIAN_POINT ( 'NONE',  ( -4.784657899331156372, -89.89547149457075648, 1.454677039711874675 ) ) ;
#7589=CARTESIAN_POINT ( 'NONE',  ( -1.069819614139537967, -78.15452850542924068, -2.969112962950023249 ) ) ;
#7594=CARTESIAN_POINT ( 'NONE',  ( 4.725907263620339194, -59.40452850542926200, -1.635492904037697981 ) ) ;
#7595=CARTESIAN_POINT ( 'NONE',  ( 4.191402346623077868, -70.69547149457073942, -5.607243785695398941 ) ) ;
#7598=CARTESIAN_POINT ( 'NONE',  ( -1.529537955723778486, -65.14547149457074227, -5.030887037049945221 ) ) ;
#7599=CARTESIAN_POINT ( 'NONE',  ( -4.784657899331159925, -62.89547149457074227, 1.454677039711874675 ) ) ;
#7601=CARTESIAN_POINT ( 'NONE',  ( 4.784657899331207886, -59.10452850542925773, 1.454677039711774533 ) ) ;
#7603=CARTESIAN_POINT ( 'NONE',  ( 4.784657899331208775, -65.10452850542924352, 1.454677039711774533 ) ) ;
#7604=CARTESIAN_POINT ( 'NONE',  ( 1.529537955723794251, -63.64547149457074227, 5.030887037049945221 ) ) ;
#7611=CARTESIAN_POINT ( 'NONE',  ( 2.862020680886514512, -77.70452850542926626, -4.100960146804039752 ) ) ;
#7612=CARTESIAN_POINT ( 'NONE',  ( 4.194503406049402194, -84.94547149457073942, 3.171033256558012159 ) ) ;
#7613=CARTESIAN_POINT ( 'NONE',  ( 0.09506052544085781542, -58.50452850542925631, 4.999999999999997335 ) ) ;
#7614=CARTESIAN_POINT ( 'NONE',  ( 2.823794231030059887, -76.09547149457073090, 1.017458915287723809 ) ) ;
#7615=CARTESIAN_POINT ( 'NONE',  ( 0.09506052544088212930, -82.50452850542926342, 6.999999999999997335 ) ) ;
#7616=CARTESIAN_POINT ( 'NONE',  ( -4.312004677470991254, -90.04547149457071953, 3.009306630940933758 ) ) ;
#7618=CARTESIAN_POINT ( 'NONE',  ( 0.09506052544085781542, -58.50452850542925631, 4.999999999999997335 ) ) ;
#7619=CARTESIAN_POINT ( 'NONE',  ( -2.179377348189461827, -73.35452850542924352, 7.030887037049988741 ) ) ;
#7620=CARTESIAN_POINT ( 'NONE',  ( 2.882544866740879286, -91.39547149457074227, -0.8366430509619593447 ) ) ;
#7625=ORIENTED_EDGE ( 'NONE', *, *, #1855, .T. ) ;
#7626=CARTESIAN_POINT ( 'NONE',  ( 4.725907263620342746, -95.40452850542925489, -1.635492904037697981 ) ) ;
#7627=CARTESIAN_POINT ( 'NONE',  ( 1.686450176301583559, -62.70452850542925916, -2.482926158054133303 ) ) ;
#7628=CARTESIAN_POINT ( 'NONE',  ( -6.628020296210623385, -57.90452850542925489, 2.253526892787613978 ) ) ;
#7629=CARTESIAN_POINT ( 'NONE',  ( 6.686770931921476979, -70.39547149457072805, -2.072711028461788896 ) ) ;
#7631=CARTESIAN_POINT ( 'NONE',  ( -4.784657899331157260, -86.89547149457074227, 1.454677039711874675 ) ) ;
#7632=CARTESIAN_POINT ( 'NONE',  ( -2.823794231030021251, -75.90452850542925489, 1.017458915287783316 ) ) ;
#7637=CARTESIAN_POINT ( 'NONE',  ( 2.882544866740897049, -83.10452850542927195, 0.8366430509618999478 ) ) ;
#7638=CARTESIAN_POINT ( 'NONE',  ( -6.686770931921460992, -62.89547149457074227, 2.072711028461789784 ) ) ;
#7640=PRODUCT_DEFINITION_SHAPE ( 'NONE', 'NONE',  #5865 ) ;
#7641=CARTESIAN_POINT ( 'NONE',  ( 5.257311121191341030, -61.24547149457074369, 0.09995255151718437925 ) ) ;
#7642=CARTESIAN_POINT ( 'NONE',  ( -2.369498399071054529, -96.34547149457074511, 6.969112962950058332 ) ) ;
#7643=CARTESIAN_POINT ( 'NONE',  ( -1.840261337453249491, -93.30452850542926058, -2.371175808195547852 ) ) ;
#7646=CARTESIAN_POINT ( 'NONE',  ( -1.529537955723670795, -73.35452850542922931, 5.030887037049979860 ) ) ;
#7647=CARTESIAN_POINT ( 'NONE',  ( -2.179377348189608821, -95.14547149457074227, -7.030887037049939003 ) ) ;
#7651=SHAPE_DEFINITION_REPRESENTATION ( #7640, #1066 ) ;
#7655=CARTESIAN_POINT ( 'NONE',  ( -5.257311121191323267, -81.75452850542926342, 0.09995255151729526277 ) ) ;
#7656=CARTESIAN_POINT ( 'NONE',  ( -3.015831842038126709, -93.19547149457075363, 3.989209796945492048 ) ) ;
#7658=CARTESIAN_POINT ( 'NONE',  ( 0.8796985632579613634, -72.64547149457072805, 3.030887037049952326 ) ) ;
#7660=CARTESIAN_POINT ( 'NONE',  ( 6.686770931921524941, -80.10452850542927195, 2.072711028461649008 ) ) ;
#7661=CARTESIAN_POINT ( 'NONE',  ( 3.015831842038150690, -91.69547149457073942, -3.989209796945492048 ) ) ;
#7663=CARTESIAN_POINT ( 'NONE',  ( 5.895805022753406455, -74.55452850542926058, -4.407101234057908989 ) ) ;
#7664=CARTESIAN_POINT ( 'NONE',  ( -3.154386672714787565, -89.74547149457073658, -0.09995255151720625064 ) ) ;
#7670=CARTESIAN_POINT ( 'NONE',  ( -5.257311121191321490, -93.75452850542927763, 0.09995255151729529053 ) ) ;
#7671=CARTESIAN_POINT ( 'NONE',  ( 2.823794231030038571, -59.40452850542925489, -1.017458915287783316 ) ) ;
#7673=CARTESIAN_POINT ( 'NONE',  ( 1.529537955723692999, -95.85452850542922931, -5.030887037049978971 ) ) ;
#7674=CARTESIAN_POINT ( 'NONE',  ( -5.895805022753479285, -65.44547149457075363, -4.407101234057782868 ) ) ;
#7675=CARTESIAN_POINT ( 'NONE',  ( -5.257311121191322378, -89.74547149457072237, -0.09995255151718372699 ) ) ;
#7676=CARTESIAN_POINT ( 'NONE',  ( 0.09506052544083881672, -76.50452850542926342, 2.999999999999997780 ) ) ;
#7679=CARTESIAN_POINT ( 'NONE',  ( 2.823794231030041235, -86.40452850542926910, -1.017458915287783316 ) ) ;
#7680=CARTESIAN_POINT ( 'NONE',  ( -2.179377348189612817, -65.14547149457074227, -7.030887037049939003 ) ) ;
#7682=CARTESIAN_POINT ( 'NONE',  ( 1.529537955723793585, -60.64547149457074227, 5.030887037049945221 ) ) ;
#7683=CARTESIAN_POINT ( 'NONE',  ( 2.862020680886597557, -60.79547149457074084, 4.100960146803977580 ) ) ;
#7684=CARTESIAN_POINT ( 'NONE',  ( 0.09506052544084069023, -91.50452850542926342, 2.999999999999997780 ) ) ;
#7686=CARTESIAN_POINT ( 'NONE',  ( -4.194503406049319594, -70.05452850542923215, 3.171033256558100533 ) ) ;
#7687=CARTESIAN_POINT ( 'NONE',  ( 4.191402346623080533, -91.69547149457075363, -5.607243785695398941 ) ) ;
#7695=CARTESIAN_POINT ( 'NONE',  ( 4.312004677471076519, -79.95452850542922363, 3.009306630940844496 ) ) ;
#7696=CARTESIAN_POINT ( 'NONE',  ( 2.862020680886599333, -75.79547149457074795, 4.100960146803977580 ) ) ;
#7698=CARTESIAN_POINT ( 'NONE',  ( -0.8796985632579433778, -74.14547149457074227, -3.030887037049952326 ) ) ;
#7699=CARTESIAN_POINT ( 'NONE',  ( -6.628020296210620721, -75.90452850542925489, 2.253526892787613978 ) ) ;
#7700=CARTESIAN_POINT ( 'NONE',  ( 5.257311121191341918, -82.24547149457070816, 0.09995255151718437925 ) ) ;
#7701=CARTESIAN_POINT ( 'NONE',  ( -1.529537955723672349, -58.35452850542924352, 5.030887037049979860 ) ) ;
#7702=CARTESIAN_POINT ( 'NONE',  ( 4.312004677471078296, -91.95452850542925205, 3.009306630940844496 ) ) ;
#7703=CARTESIAN_POINT ( 'NONE',  ( -7.360235569667858080, -81.75452850542926342, 0.09995255151731782806 ) ) ;
#7704=CARTESIAN_POINT ( 'NONE',  ( 2.823794231030060775, -85.09547149457075932, 1.017458915287723809 ) ) ;
#7709=CARTESIAN_POINT ( 'NONE',  ( -5.257311121191322378, -87.75452850542922079, 0.09995255151729526277 ) ) ;
#7711=CARTESIAN_POINT ( 'NONE',  ( 3.015831842038235067, -85.80452850542926058, 3.989209796945429432 ) ) ;
#7712=CARTESIAN_POINT ( 'NONE',  ( -1.069819614139540187, -63.15452850542925489, -2.969112962950023249 ) ) ;
#7713=CARTESIAN_POINT ( 'NONE',  ( 2.179377348189479591, -59.85452850542925773, -7.030887037049986077 ) ) ;
#7714=CARTESIAN_POINT ( 'NONE',  ( 5.895805022753492608, -72.94547149457073942, 4.407101234057782868 ) ) ;
#7715=CARTESIAN_POINT ( 'NONE',  ( 4.194503406049403083, -84.94547149457073942, 3.171033256558012159 ) ) ;
#7716=CARTESIAN_POINT ( 'NONE',  ( -1.686450176301566017, -73.20452850542925205, 2.482926158054133303 ) ) ;
#7720=CARTESIAN_POINT ( 'NONE',  ( 2.493201789345272701, -86.55452850542926058, -1.934965279058294518 ) ) ;
#7721=CARTESIAN_POINT ( 'NONE',  ( 5.895805022753492608, -60.94547149457074653, 4.407101234057782868 ) ) ;
#7724=CARTESIAN_POINT ( 'NONE',  ( 2.862020680886598445, -66.79547149457073374, 4.100960146803977580 ) ) ;
#7725=CARTESIAN_POINT ( 'NONE',  ( 6.686770931921480532, -97.39547149457074227, -2.072711028461788896 ) ) ;
#7730=CARTESIAN_POINT ( 'NONE',  ( -0.09506052544084261924, -57.00452850542924921, -4.999999999999997335 ) ) ;
#7732=CARTESIAN_POINT ( 'NONE',  ( 4.037591185471564259, -93.79547149457076216, 5.718994135553860936 ) ) ;
#7735=CARTESIAN_POINT ( 'NONE',  ( 1.719659006605391172, -76.65452850542922647, 4.969112962950016588 ) ) ;
#7739=CARTESIAN_POINT ( 'NONE',  ( 4.784657899331177688, -79.39547149457074227, -1.454677039711874009 ) ) ;
#7740=CARTESIAN_POINT ( 'NONE',  ( 0.09506052544075295485, -58.99547149457073658, -4.999999999999997335 ) ) ;
#7741=CARTESIAN_POINT ( 'NONE',  ( -2.882544866740858414, -74.89547149457074227, 0.8366430509619596778 ) ) ;
#7742=CARTESIAN_POINT ( 'NONE',  ( 2.179377348189480923, -68.85452850542924352, -7.030887037049986077 ) ) ;
#7744=CARTESIAN_POINT ( 'NONE',  ( -2.862020680886580237, -80.29547149457074795, -4.100960146803977580 ) ) ;
#7745=CARTESIAN_POINT ( 'NONE',  ( 4.725907263620339194, -62.40452850542925489, -1.635492904037697981 ) ) ;
#7747=CARTESIAN_POINT ( 'NONE',  ( 2.369498399071224171, -67.65452850542925489, 6.969112962950009482 ) ) ;
#7748=CARTESIAN_POINT ( 'NONE',  ( -2.882544866740858414, -74.89547149457074227, 0.8366430509619596778 ) ) ;
#7753=CARTESIAN_POINT ( 'NONE',  ( -4.312004677471056091, -87.45452850542925205, -3.009306630940844052 ) ) ;
#7755=CARTESIAN_POINT ( 'NONE',  ( 0.09506052544086046607, -79.50452850542926342, 4.999999999999997335 ) ) ;
#7756=CARTESIAN_POINT ( 'NONE',  ( 1.069819614139497332, -97.84547149457073090, -2.969112962950042789 ) ) ;
#7757=EDGE_CURVE ( 'NONE', #1139, #4707, #252, .T. ) ;
#7759=CARTESIAN_POINT ( 'NONE',  ( 4.194503406049339134, -86.55452850542926058, -3.171033256558100089 ) ) ;
#7760=CARTESIAN_POINT ( 'NONE',  ( -5.895805022753480173, -59.44547149457074653, -4.407101234057782868 ) ) ;
#7761=CARTESIAN_POINT ( 'NONE',  ( -5.257311121191325043, -80.74547149457075079, -0.09995255151718372699 ) ) ;
#7762=CARTESIAN_POINT ( 'NONE',  ( -1.069819614139538411, -75.15452850542922647, -2.969112962950023249 ) ) ;
#7765=CARTESIAN_POINT ( 'NONE',  ( 2.610703060766985217, -88.95452850542925205, 1.773238653441072232 ) ) ;
#7766=CARTESIAN_POINT ( 'NONE',  ( 6.628020296210643814, -95.40452850542926910, -2.253526892787612645 ) ) ;
#7768=CARTESIAN_POINT ( 'NONE',  ( -1.529537955723670128, -79.35452850542925773, 5.030887037049979860 ) ) ;
#7769=CARTESIAN_POINT ( 'NONE',  ( 6.013306294175080779, -94.54547149457073374, -4.245374608440741326 ) ) ;
#7771=DIRECTION ( 'NONE',  ( -1.261617073437677752E-16, 1.000000000000000000, 0.000000000000000000 ) ) ;
#7772=CARTESIAN_POINT ( 'NONE',  ( 4.194503406049334693, -62.55452850542925347, -3.171033256558100089 ) ) ;
#7774=CARTESIAN_POINT ( 'NONE',  ( 0.09506052544073653743, -94.99547149457075079, -6.999999999999997335 ) ) ;
#7778=CARTESIAN_POINT ( 'NONE',  ( -1.529537955723670795, -73.35452850542922931, 5.030887037049979860 ) ) ;
#7781=CARTESIAN_POINT ( 'NONE',  ( -1.719659006605265050, -78.34547149457074511, 4.969112962950051227 ) ) ;
#7783=CARTESIAN_POINT ( 'NONE',  ( 3.182720709228878064, -96.99999999999995737, -2.580399204195190865 ) ) ;
#7784=CARTESIAN_POINT ( 'NONE',  ( -1.840261337453201973, -66.19547149457073942, 2.371175808195584267 ) ) ;
#7785=CARTESIAN_POINT ( 'NONE',  ( -2.369498399071207739, -69.15452850542926910, -6.969112962950009482 ) ) ;
#7787=CARTESIAN_POINT ( 'NONE',  ( -4.725907263620353405, -77.59547149457074511, -1.635492904037597617 ) ) ;
#7788=CARTESIAN_POINT ( 'NONE',  ( -4.784657899331191899, -60.60452850542925773, -1.454677039711773867 ) ) ;
#7789=CARTESIAN_POINT ( 'NONE',  ( 4.784657899331211439, -86.10452850542925773, 1.454677039711774533 ) ) ;
#7790=CARTESIAN_POINT ( 'NONE',  ( 4.037591185471441690, -68.70452850542925205, -5.718994135553947977 ) ) ;
#7791=CARTESIAN_POINT ( 'NONE',  ( -2.610703060766926153, -78.04547149457074795, 1.773238653441125745 ) ) ;
#7796=CARTESIAN_POINT ( 'NONE',  ( 4.725907263620341858, -86.40452850542926910, -1.635492904037697981 ) ) ;
#7798=CARTESIAN_POINT ( 'NONE',  ( -1.719659006605371410, -84.15452850542925489, -4.969112962950015699 ) ) ;
#7799=CARTESIAN_POINT ( 'NONE',  ( 1.069819614139495556, -85.84547149457074511, -2.969112962950042789 ) ) ;
#7801=CARTESIAN_POINT ( 'NONE',  ( 4.725907263620341858, -89.40452850542926910, -1.635492904037697981 ) ) ;
#7802=CARTESIAN_POINT ( 'NONE',  ( -6.628020296210670459, -59.59547149457074511, -2.253526892787471869 ) ) ;
#7804=CARTESIAN_POINT ( 'NONE',  ( -2.823794231030022139, -66.90452850542925489, 1.017458915287783316 ) ) ;
#7809=CARTESIAN_POINT ( 'NONE',  ( 0.8796985632579006342, -89.85452850542924352, -3.030887037049972310 ) ) ;
#7810=CARTESIAN_POINT ( 'NONE',  ( 4.037591185471560706, -63.79547149457074084, 5.718994135553860936 ) ) ;
#7812=CARTESIAN_POINT ( 'NONE',  ( -4.784657899331190123, -81.60452850542925773, -1.454677039711773867 ) ) ;
#7813=CARTESIAN_POINT ( 'NONE',  ( 6.013306294175080779, -88.54547149457074795, -4.245374608440741326 ) ) ;
#7817=CARTESIAN_POINT ( 'NONE',  ( -1.069819614139475794, -69.34547149457073090, 2.969112962950044121 ) ) ;
#7821=CARTESIAN_POINT ( 'NONE',  ( -6.686770931921456551, -89.89547149457074227, 2.072711028461789784 ) ) ;
#7823=CARTESIAN_POINT ( 'NONE',  ( -4.784657899331190123, -72.60452850542925773, -1.454677039711773867 ) ) ;
#7827=CARTESIAN_POINT ( 'NONE',  ( 1.529537955723795584, -81.64547149457074227, 5.030887037049945221 ) ) ;
#7828=EDGE_CURVE ( 'NONE', #6384, #4976, #2798, .T. ) ;
#7829=CARTESIAN_POINT ( 'NONE',  ( 4.245875450176646915, -97.00000000000000000, 2.474278829614704467 ) ) ;
#7830=CARTESIAN_POINT ( 'NONE',  ( -1.686450176301618864, -62.29547149457074084, -2.482926158054096000 ) ) ;
#7831=CARTESIAN_POINT ( 'NONE',  ( 6.686770931921523164, -74.10452850542924352, 2.072711028461649008 ) ) ;
#7833=CARTESIAN_POINT ( 'NONE',  ( 0.09506052544075563326, -79.99547149457075079, -4.999999999999997335 ) ) ;
#7835=CARTESIAN_POINT ( 'NONE',  ( 2.862020680886515844, -89.70452850542926626, -4.100960146804039752 ) ) ;
#7836=CARTESIAN_POINT ( 'NONE',  ( -2.179377348189462271, -67.35452850542924352, 7.030887037049988741 ) ) ;
#7837=CARTESIAN_POINT ( 'NONE',  ( -0.8796985632579433778, -74.14547149457074227, -3.030887037049952326 ) ) ;
#7840=CARTESIAN_POINT ( 'NONE',  ( -0.09506052544083770650, -96.00452850542926342, -4.999999999999997335 ) ) ;
#7841=CARTESIAN_POINT ( 'NONE',  ( -0.09506052544083884448, -87.00452850542924921, -4.999999999999997335 ) ) ;
#7843=CARTESIAN_POINT ( 'NONE',  ( -1.529537955723669018, -85.35452850542925773, 5.030887037049979860 ) ) ;
#7844=CARTESIAN_POINT ( 'NONE',  ( -2.882544866740855749, -92.89547149457074227, 0.8366430509619596778 ) ) ;
#7846=CARTESIAN_POINT ( 'NONE',  ( 1.529537955723691889, -86.85452850542921510, -5.030887037049978971 ) ) ;
#7848=CARTESIAN_POINT ( 'NONE',  ( -6.686770931921460992, -62.89547149457074227, 2.072711028461789784 ) ) ;
#7849=CARTESIAN_POINT ( 'NONE',  ( 1.686450176301583559, -62.70452850542925916, -2.482926158054133303 ) ) ;
#7852=CARTESIAN_POINT ( 'NONE',  ( 2.610703060766984329, -82.95452850542925205, 1.773238653441072232 ) ) ;
#7853=CARTESIAN_POINT ( 'NONE',  ( -2.369498399071205075, -90.15452850542926910, -6.969112962950009482 ) ) ;
#7855=CARTESIAN_POINT ( 'NONE',  ( 2.179377348189630137, -84.64547149457074227, 7.030887037049939003 ) ) ;
#7859=CARTESIAN_POINT ( 'NONE',  ( 0.8796985632579604752, -66.64547149457072805, 3.030887037049952326 ) ) ;
#7860=CARTESIAN_POINT ( 'NONE',  ( -5.257311121191324155, -60.75452850542925631, 0.09995255151729526277 ) ) ;
#7862=CARTESIAN_POINT ( 'NONE',  ( -1.719659006605374074, -63.15452850542925489, -4.969112962950016588 ) ) ;
#7863=CARTESIAN_POINT ( 'NONE',  ( 6.686770931921479644, -85.39547149457074227, -2.072711028461788896 ) ) ;
#7864=( NAMED_UNIT ( * ) PLANE_ANGLE_UNIT ( ) SI_UNIT ( $, .RADIAN. ) );
#7866=CARTESIAN_POINT ( 'NONE',  ( -4.725907263620320542, -78.90452850542925489, 1.635492904037698647 ) ) ;
#7872=CARTESIAN_POINT ( 'NONE',  ( 5.257311121191341918, -76.24547149457073658, 0.09995255151718437925 ) ) ;
#7873=CARTESIAN_POINT ( 'NONE',  ( -2.938187887435717016E-14, -97.00000000000001421, -3.999999999999997335 ) ) ;
#7874=CARTESIAN_POINT ( 'NONE',  ( -3.154386672714792006, -59.74547149457073658, -0.09995255151720625064 ) ) ;
#7875=CARTESIAN_POINT ( 'NONE',  ( -5.895805022753386027, -73.05452850542926058, 4.407101234057909878 ) ) ;
#7877=CARTESIAN_POINT ( 'NONE',  ( 4.725907263620372945, -76.09547149457074511, 1.635492904037598283 ) ) ;
#7879=CARTESIAN_POINT ( 'NONE',  ( -4.784657899331189235, -87.60452850542925773, -1.454677039711773867 ) ) ;
#7880=CARTESIAN_POINT ( 'NONE',  ( -6.686770931921506289, -66.60452850542924352, -2.072711028461647675 ) ) ;
#7882=CARTESIAN_POINT ( 'NONE',  ( -2.610703060766926153, -75.04547149457074795, 1.773238653441125745 ) ) ;
#7885=CARTESIAN_POINT ( 'NONE',  ( -3.015831842038213306, -93.30452850542926058, -3.989209796945429432 ) ) ;
#7886=CARTESIAN_POINT ( 'NONE',  ( -4.194503406049316041, -85.05452850542926058, 3.171033256558100533 ) ) ;
#7888=CARTESIAN_POINT ( 'NONE',  ( 1.529537955723690112, -74.85452850542925773, -5.030887037049978971 ) ) ;
#7889=CARTESIAN_POINT ( 'NONE',  ( -0.8796985632579414904, -89.14547149457072805, -3.030887037049952326 ) ) ;
#7890=CARTESIAN_POINT ( 'NONE',  ( 4.312004677471078296, -85.95452850542925205, 3.009306630940844496 ) ) ;
#7891=CARTESIAN_POINT ( 'NONE',  ( 4.037591185471445243, -95.70452850542928047, -5.718994135553947977 ) ) ;
#7892=CARTESIAN_POINT ( 'NONE',  ( 0.8796985632578979697, -68.85452850542924352, -3.030887037049972310 ) ) ;
#7896=CARTESIAN_POINT ( 'NONE',  ( 0.8796985632578991909, -77.85452850542925773, -3.030887037049972310 ) ) ;
#7897=CARTESIAN_POINT ( 'NONE',  ( -4.037591185471421262, -91.20452850542925205, 5.718994135553947977 ) ) ;
#7900=CARTESIAN_POINT ( 'NONE',  ( 6.686770931921479644, -85.39547149457074227, -2.072711028461788896 ) ) ;
#7903=CARTESIAN_POINT ( 'NONE',  ( -2.610703060766926598, -69.04547149457074795, 1.773238653441125745 ) ) ;
#7904=CARTESIAN_POINT ( 'NONE',  ( -2.862020680886496304, -61.20452850542925205, 4.100960146804039752 ) ) ;
#7906=CARTESIAN_POINT ( 'NONE',  ( 3.015831842038233290, -70.80452850542926058, 3.989209796945429432 ) ) ;
#7907=CARTESIAN_POINT ( 'NONE',  ( 4.037591185471563371, -81.79547149457074795, 5.718994135553860936 ) ) ;
#7909=CARTESIAN_POINT ( 'NONE',  ( 1.719659006605389839, -70.65452850542926910, 4.969112962950016588 ) ) ;
#7912=CARTESIAN_POINT ( 'NONE',  ( -3.015831842038129817, -69.19547149457073942, 3.989209796945492048 ) ) ;
#7914=CARTESIAN_POINT ( 'NONE',  ( -2.493201789345292241, -62.44547149457074653, -1.934965279058240561 ) ) ;
#7915=CARTESIAN_POINT ( 'NONE',  ( -4.191402346623180009, -66.30452850542926058, -5.607243785695311900 ) ) ;
#7918=CARTESIAN_POINT ( 'NONE',  ( -1.719659006605371188, -84.15452850542925489, -4.969112962950016588 ) ) ;
#7919=CARTESIAN_POINT ( 'NONE',  ( -7.360235569667858968, -69.75452850542926342, 0.09995255151731782806 ) ) ;
#7920=CARTESIAN_POINT ( 'NONE',  ( 2.610703060766946138, -79.54547149457074795, -1.773238653441125523 ) ) ;
#7926=CARTESIAN_POINT ( 'NONE',  ( 1.719659006605390283, -73.65452850542924068, 4.969112962950016588 ) ) ;
#7927=VERTEX_POINT ( 'NONE', #7740 ) ;
#7928=CARTESIAN_POINT ( 'NONE',  ( -2.862020680886495416, -70.20452850542925205, 4.100960146804039752 ) ) ;
#7929=CARTESIAN_POINT ( 'NONE',  ( -2.493201789345289132, -92.44547149457073942, -1.934965279058240561 ) ) ;
#7930=CARTESIAN_POINT ( 'NONE',  ( -4.725907263620319654, -90.90452850542926910, 1.635492904037698647 ) ) ;
#7931=CARTESIAN_POINT ( 'NONE',  ( 4.191402346623076980, -64.69547149457073942, -5.607243785695398941 ) ) ;
#7932=CARTESIAN_POINT ( 'NONE',  ( -2.493201789345253161, -70.05452850542926058, 1.934965279058294518 ) ) ;
#7936=CARTESIAN_POINT ( 'NONE',  ( -1.069819614139538411, -75.15452850542922647, -2.969112962950023249 ) ) ;
#7937=CARTESIAN_POINT ( 'NONE',  ( 2.369498399071227279, -91.65452850542924068, 6.969112962950009482 ) ) ;
#7939=CARTESIAN_POINT ( 'NONE',  ( -6.686770931921456551, -92.89547149457074227, 2.072711028461789784 ) ) ;
#7940=CARTESIAN_POINT ( 'NONE',  ( -2.938187887435717016E-14, -97.00000000000001421, -3.999999999999997335 ) ) ;
#7942=CARTESIAN_POINT ( 'NONE',  ( -2.882544866740859302, -65.89547149457074227, 0.8366430509619596778 ) ) ;
#7947=CARTESIAN_POINT ( 'NONE',  ( -4.312004677471058756, -66.45452850542925205, -3.009306630940844052 ) ) ;
#7948=CARTESIAN_POINT ( 'NONE',  ( -4.037591185471544719, -80.29547149457074795, -5.718994135553860936 ) ) ;
#7951=CARTESIAN_POINT ( 'NONE',  ( 2.862020680886513180, -68.70452850542925205, -4.100960146804039752 ) ) ;
#7953=CARTESIAN_POINT ( 'NONE',  ( -4.312004677470993919, -72.04547149457074795, 3.009306630940933758 ) ) ;
#7955=CARTESIAN_POINT ( 'NONE',  ( 5.257311121191343695, -97.24547149457075079, 0.09995255151718437925 ) ) ;
#7956=CARTESIAN_POINT ( 'NONE',  ( 2.179377348189479591, -59.85452850542925773, -7.030887037049986077 ) ) ;
#7960=CARTESIAN_POINT ( 'NONE',  ( -4.312004677471056979, -81.45452850542923784, -3.009306630940844052 ) ) ;
#7961=CARTESIAN_POINT ( 'NONE',  ( -4.191402346623180897, -63.30452850542926058, -5.607243785695311900 ) ) ;
#7962=CARTESIAN_POINT ( 'NONE',  ( 2.610703060766944805, -73.54547149457074795, -1.773238653441125523 ) ) ;
#7966=CARTESIAN_POINT ( 'NONE',  ( 4.784657899331209663, -77.10452850542925773, 1.454677039711774533 ) ) ;
#7968=CARTESIAN_POINT ( 'NONE',  ( -4.784657899331190123, -72.60452850542925773, -1.454677039711773867 ) ) ;
#7969=CARTESIAN_POINT ( 'NONE',  ( 1.686450176301638182, -93.79547149457076216, 2.482926158054096000 ) ) ;
#7970=CARTESIAN_POINT ( 'NONE',  ( -1.529537955723774489, -95.14547149457074227, -5.030887037049945221 ) ) ;
#7971=CARTESIAN_POINT ( 'NONE',  ( 4.312004677471075631, -76.95452850542923784, 3.009306630940844496 ) ) ;
#7972=CARTESIAN_POINT ( 'NONE',  ( 7.360235569667880284, -89.25452850542926342, -0.09995255151731691212 ) ) ;
#7973=CARTESIAN_POINT ( 'NONE',  ( -1.686450176301566906, -67.20452850542925205, 2.482926158054133303 ) ) ;
#7977=CARTESIAN_POINT ( 'NONE',  ( -1.840261337453251933, -75.30452850542926058, -2.371175808195547852 ) ) ;
#7978=CARTESIAN_POINT ( 'NONE',  ( -2.179377348189459607, -91.35452850542925773, 7.030887037049988741 ) ) ;
#7979=CARTESIAN_POINT ( 'NONE',  ( 2.179377348189630581, -87.64547149457075648, 7.030887037049939003 ) ) ;
#7982=CARTESIAN_POINT ( 'NONE',  ( -3.154386672714790674, -71.74547149457075079, -0.09995255151720625064 ) ) ;
#7986=CARTESIAN_POINT ( 'NONE',  ( -0.09506052544084148126, -66.00452850542926342, -4.999999999999997335 ) ) ;
#7987=CARTESIAN_POINT ( 'NONE',  ( -7.360235569667858080, -83.74547149457075079, -0.09995255151716124498 ) ) ;
#7989=CARTESIAN_POINT ( 'NONE',  ( 3.015831842038148913, -76.69547149457075363, -3.989209796945492048 ) ) ;
#7990=CARTESIAN_POINT ( 'NONE',  ( -1.719659006605373630, -66.15452850542926910, -4.969112962950016588 ) ) ;
#7993=CARTESIAN_POINT ( 'NONE',  ( -4.194503406049384431, -71.44547149457075363, -3.171033256558012159 ) ) ;
#7995=CARTESIAN_POINT ( 'NONE',  ( -1.529537955723774489, -95.14547149457074227, -5.030887037049945221 ) ) ;
#7997=CARTESIAN_POINT ( 'NONE',  ( 6.013306294175167821, -61.95452850542925916, 4.245374608440616093 ) ) ;
#8003=ORIENTED_EDGE ( 'NONE', *, *, #2532, .T. ) ;
#8005=CARTESIAN_POINT ( 'NONE',  ( -5.257311121191323267, -84.75452850542923500, 0.09995255151729526277 ) ) ;
#8006=CARTESIAN_POINT ( 'NONE',  ( -3.015831842038215083, -75.30452850542926058, -3.989209796945429432 ) ) ;
#8008=CARTESIAN_POINT ( 'NONE',  ( -3.015831842038215527, -72.30452850542926058, -3.989209796945429432 ) ) ;
#8009=CARTESIAN_POINT ( 'NONE',  ( 1.840261337453220847, -82.69547149457073942, -2.371175808195584267 ) ) ;
#8011=CARTESIAN_POINT ( 'NONE',  ( 4.784657899331180353, -97.39547149457074227, -1.454677039711874009 ) ) ;
#8012=CARTESIAN_POINT ( 'NONE',  ( 4.194503406049338246, -80.55452850542926058, -3.171033256558100089 ) ) ;
#8013=CARTESIAN_POINT ( 'NONE',  ( -6.628020296210619833, -90.90452850542926910, 2.253526892787613978 ) ) ;
#8015=CARTESIAN_POINT ( 'NONE',  ( -0.8796985632578812053, -61.35452850542925773, 3.030887037049973198 ) ) ;
#8020=CARTESIAN_POINT ( 'NONE',  ( 1.069819614139556840, -73.65452850542925489, 2.969112962950023249 ) ) ;
#8021=CARTESIAN_POINT ( 'NONE',  ( -7.360235569667858080, -84.75452850542926342, 0.09995255151731782806 ) ) ;
#8022=CARTESIAN_POINT ( 'NONE',  ( 6.628020296210689111, -82.09547149457075932, 2.253526892787472757 ) ) ;
#8024=CARTESIAN_POINT ( 'NONE',  ( -1.529537955723774711, -95.14547149457074227, -5.030887037049945221 ) ) ;
#8025=CARTESIAN_POINT ( 'NONE',  ( -2.882544866740876621, -81.60452850542927195, -0.8366430509618996147 ) ) ;
#8030=CARTESIAN_POINT ( 'NONE',  ( -3.015831842038215527, -72.30452850542926058, -3.989209796945429432 ) ) ;
#8031=CARTESIAN_POINT ( 'NONE',  ( -6.013306294175058575, -84.04547149457074795, 4.245374608440741326 ) ) ;
#8033=CARTESIAN_POINT ( 'NONE',  ( 2.862020680886599333, -75.79547149457074795, 4.100960146803977580 ) ) ;
#8034=CARTESIAN_POINT ( 'NONE',  ( 4.312004677471011682, -73.54547149457073374, -3.009306630940933314 ) ) ;
#8035=CARTESIAN_POINT ( 'NONE',  ( -4.312004677471060532, -63.45452850542926626, -3.009306630940844052 ) ) ;
#8037=CARTESIAN_POINT ( 'NONE',  ( 0.09506052544075412059, -67.99547149457075079, -4.999999999999997335 ) ) ;
#8038=CARTESIAN_POINT ( 'NONE',  ( 0.3811618011801478634, -97.00000000000001421, -4.000000000000000888 ) ) ;
#8039=CARTESIAN_POINT ( 'NONE',  ( 5.895805022753402902, -59.55452850542924637, -4.407101234057908989 ) ) ;
#8042=PRODUCT ( 'return spring', 'return spring', '', ( #6346 ) ) ;
#8045=CARTESIAN_POINT ( 'NONE',  ( 2.862020680886514956, -83.70452850542925205, -4.100960146804039752 ) ) ;
#8046=CARTESIAN_POINT ( 'NONE',  ( -4.312004677471056979, -81.45452850542923784, -3.009306630940844052 ) ) ;
#8048=CARTESIAN_POINT ( 'NONE',  ( -2.862020680886495416, -67.20452850542925205, 4.100960146804039752 ) ) ;
#8049=CARTESIAN_POINT ( 'NONE',  ( 2.493201789345310004, -78.94547149457073942, 1.934965279058241006 ) ) ;
#8050=CARTESIAN_POINT ( 'NONE',  ( -3.154386672714792006, -59.74547149457073658, -0.09995255151720625064 ) ) ;
#8051=CARTESIAN_POINT ( 'NONE',  ( 3.015831842038233734, -73.80452850542926058, 3.989209796945429432 ) ) ;
#8052=CARTESIAN_POINT ( 'NONE',  ( 6.013306294175171374, -88.95452850542925205, 4.245374608440616093 ) ) ;
#8054=CARTESIAN_POINT ( 'NONE',  ( -2.610703060766967454, -57.45452850542925916, -1.773238653441072232 ) ) ;
#8058=CARTESIAN_POINT ( 'NONE',  ( -4.056271377811393464E-14, -97.00000000000000000, -4.999999999999996447 ) ) ;
#8059=CARTESIAN_POINT ( 'NONE',  ( -2.882544866740878842, -66.60452850542924352, -0.8366430509618996147 ) ) ;
#8060=CARTESIAN_POINT ( 'NONE',  ( -2.179377348189610597, -77.14547149457074227, -7.030887037049939003 ) ) ;
#8062=CARTESIAN_POINT ( 'NONE',  ( 4.312004677471013459, -94.54547149457073374, -3.009306630940932425 ) ) ;
#8063=CARTESIAN_POINT ( 'NONE',  ( -0.09506052544081858291, -81.00452850542926342, -2.999999999999997780 ) ) ;
#8064=EDGE_CURVE ( 'NONE', #1590, #1139, #1270, .T. ) ;
#8069=CARTESIAN_POINT ( 'NONE',  ( -0.09506052544084261924, -57.00452850542924921, -4.999999999999997335 ) ) ;
#8071=CARTESIAN_POINT ( 'NONE',  ( -0.09506052544071530441, -66.49547149457075079, 6.999999999999997335 ) ) ;
#8072=ORIENTED_EDGE ( 'NONE', *, *, #6344, .T. ) ;
#8073=CARTESIAN_POINT ( 'NONE',  ( -4.784657899331159037, -71.89547149457074227, 1.454677039711874675 ) ) ;
#8074=CARTESIAN_POINT ( 'NONE',  ( 1.719659006605285034, -70.84547149457074511, -4.969112962950050338 ) ) ;
#8075=CARTESIAN_POINT ( 'NONE',  ( -1.719659006605373408, -69.15452850542924068, -4.969112962950016588 ) ) ;
#8079=CARTESIAN_POINT ( 'NONE',  ( 1.719659006605284590, -67.84547149457070248, -4.969112962950050338 ) ) ;
#8080=CARTESIAN_POINT ( 'NONE',  ( -2.369498399071207739, -60.15452850542926200, -6.969112962950009482 ) ) ;
#8087=CARTESIAN_POINT ( 'NONE',  ( 0.09506052544086160405, -88.50452850542924921, 4.999999999999997335 ) ) ;
#8088=CARTESIAN_POINT ( 'NONE',  ( -1.719659006605371854, -78.15452850542925489, -4.969112962950016588 ) ) ;
#8089=CARTESIAN_POINT ( 'NONE',  ( -4.194503406049320482, -61.05452850542925347, 3.171033256558101865 ) ) ;
#8090=CARTESIAN_POINT ( 'NONE',  ( 1.069819614139494446, -76.84547149457073090, -2.969112962950042789 ) ) ;
#8091=MECHANICAL_DESIGN_GEOMETRIC_PRESENTATION_REPRESENTATION('',(#4854),#6602);
#8092=CARTESIAN_POINT ( 'NONE',  ( 4.312004677471013459, -94.54547149457071953, -3.009306630940933314 ) ) ;
#8093=CARTESIAN_POINT ( 'NONE',  ( -1.719659006605373408, -69.15452850542924068, -4.969112962950016588 ) ) ;
#8094=CARTESIAN_POINT ( 'NONE',  ( -6.013306294175150946, -84.45452850542925205, -4.245374608440613429 ) ) ;
#8095=CARTESIAN_POINT ( 'NONE',  ( 0.09506052544083691547, -61.50452850542925631, 2.999999999999997780 ) ) ;
#8102=CARTESIAN_POINT ( 'NONE',  ( 1.686450176301584225, -68.70452850542925205, -2.482926158054133303 ) ) ;
#8103=CARTESIAN_POINT ( 'NONE',  ( -2.179377348189610597, -80.14547149457074227, -7.030887037049939003 ) ) ;
#8104=CARTESIAN_POINT ( 'NONE',  ( -4.784657899331189235, -90.60452850542925773, -1.454677039711773867 ) ) ;
#8105=CARTESIAN_POINT ( 'NONE',  ( 1.719659006605287921, -94.84547149457074511, -4.969112962950050338 ) ) ;
#8106=CARTESIAN_POINT ( 'NONE',  ( 1.069819614139558173, -85.65452850542926910, 2.969112962950023249 ) ) ;
#8109=CARTESIAN_POINT ( 'NONE',  ( 2.823794231030042567, -95.40452850542926910, -1.017458915287783316 ) ) ;
#8110=CARTESIAN_POINT ( 'NONE',  ( -2.369498399071057637, -72.34547149457073090, 6.969112962950058332 ) ) ;
#8111=CARTESIAN_POINT ( 'NONE',  ( 4.430245668755248722, -96.99999999999997158, 2.549500813230844543 ) ) ;
#8114=CARTESIAN_POINT ( 'NONE',  ( 4.784657899331176800, -73.39547149457074227, -1.454677039711874009 ) ) ;
#8115=CARTESIAN_POINT ( 'NONE',  ( 5.257311121191341918, -67.24547149457075079, 0.09995255151718437925 ) ) ;
#8116=CARTESIAN_POINT ( 'NONE',  ( 4.312004677471074743, -67.95452850542922363, 3.009306630940844496 ) ) ;
#8119=CARTESIAN_POINT ( 'NONE',  ( 2.862020680886598001, -63.79547149457074084, 4.100960146803977580 ) ) ;
#8120=CARTESIAN_POINT ( 'NONE',  ( 0.000000000000000000, 0.000000000000000000, 0.000000000000000000 ) ) ;
#8121=CARTESIAN_POINT ( 'NONE',  ( -1.529537955723667908, -94.35452850542922931, 5.030887037049979860 ) ) ;
#8125=CARTESIAN_POINT ( 'NONE',  ( -3.989863994746656317E-14, -97.00000000000000000, -4.999999999999997335 ) ) ;
#8126=CARTESIAN_POINT ( 'NONE',  ( -4.784657899331189235, -90.60452850542925773, -1.454677039711773867 ) ) ;
#8128=CARTESIAN_POINT ( 'NONE',  ( -2.862020680886578905, -92.29547149457074795, -4.100960146803977580 ) ) ;
#8129=CARTESIAN_POINT ( 'NONE',  ( -4.312004677471058756, -66.45452850542925205, -3.009306630940843608 ) ) ;
#8130=CARTESIAN_POINT ( 'NONE',  ( -1.069819614139474240, -81.34547149457074511, 2.969112962950044121 ) ) ;
#8131=CARTESIAN_POINT ( 'NONE',  ( -3.015831842038128041, -84.19547149457073942, 3.989209796945492048 ) ) ;
#8132=CARTESIAN_POINT ( 'NONE',  ( -4.194503406049319594, -67.05452850542926058, 3.171033256558100533 ) ) ;
#8133=CARTESIAN_POINT ( 'NONE',  ( 7.360235569667878508, -83.25452850542926342, -0.09995255151731691212 ) ) ;
#8134=CARTESIAN_POINT ( 'NONE',  ( -1.069819614139472019, -96.34547149457074511, 2.969112962950044121 ) ) ;
#8140=CARTESIAN_POINT ( 'NONE',  ( 4.784657899331212327, -95.10452850542925773, 1.454677039711774533 ) ) ;
#8141=CARTESIAN_POINT ( 'NONE',  ( 0.09506052544083806732, -70.50452850542926342, 2.999999999999997780 ) ) ;
#8142=CARTESIAN_POINT ( 'NONE',  ( -0.09506052544071341703, -81.49547149457075079, 6.999999999999997335 ) ) ;
#8143=CARTESIAN_POINT ( 'NONE',  ( -5.257311121191321490, -93.75452850542926342, 0.09995255151729526277 ) ) ;
#8145=CARTESIAN_POINT ( 'NONE',  ( -2.823794231030019475, -87.90452850542926910, 1.017458915287783316 ) ) ;
#8150=CARTESIAN_POINT ( 'NONE',  ( 3.154386672714811102, -95.25452850542926342, -0.09995255151727241993 ) ) ;
#8151=CARTESIAN_POINT ( 'NONE',  ( 0.09506052544073312349, -67.99547149457075079, -6.999999999999997335 ) ) ;
#8152=CARTESIAN_POINT ( 'NONE',  ( 2.712844317851120124, -96.99999999999997158, -5.329299858373291343 ) ) ;
#8153=CARTESIAN_POINT ( 'NONE',  ( -1.719659006605265272, -78.34547149457074511, 4.969112962950051227 ) ) ;
#8154=CARTESIAN_POINT ( 'NONE',  ( -0.09506052544073578803, -72.49547149457075079, 4.999999999999997335 ) ) ;
#8155=CARTESIAN_POINT ( 'NONE',  ( -1.529537955723672349, -58.35452850542924352, 5.030887037049979860 ) ) ;
#8157=CARTESIAN_POINT ( 'NONE',  ( 4.725907263620340082, -71.40452850542925489, -1.635492904037697981 ) ) ;
#8158=CARTESIAN_POINT ( 'NONE',  ( -5.257311121191324155, -62.74547149457075079, -0.09995255151718371311 ) ) ;
#8164=CARTESIAN_POINT ( 'NONE',  ( -5.257311121191322378, -87.75452850542922079, 0.09995255151729526277 ) ) ;
#8165=CARTESIAN_POINT ( 'NONE',  ( -1.529537955723776044, -86.14547149457074227, -5.030887037049945221 ) ) ;
#8166=CARTESIAN_POINT ( 'NONE',  ( -1.529537955723672127, -61.35452850542925773, 5.030887037049979860 ) ) ;
#8167=CARTESIAN_POINT ( 'NONE',  ( -0.09506052544075634103, -78.49547149457075079, 2.999999999999997780 ) ) ;
#8168=CARTESIAN_POINT ( 'NONE',  ( -6.686770931921506289, -75.60452850542924352, -2.072711028461647675 ) ) ;
#8169=CARTESIAN_POINT ( 'NONE',  ( 0.09506052544075714594, -91.99547149457073658, -4.999999999999997335 ) ) ;
#8170=CARTESIAN_POINT ( 'NONE',  ( -4.194503406049320482, -64.05452850542926058, 3.171033256558100533 ) ) ;
#8171=CARTESIAN_POINT ( 'NONE',  ( -6.013306294175150946, -81.45452850542925205, -4.245374608440613429 ) ) ;
#8172=CARTESIAN_POINT ( 'NONE',  ( 2.493201789345312669, -96.94547149457073942, 1.934965279058241006 ) ) ;
#8177=CARTESIAN_POINT ( 'NONE',  ( -2.862020680886492308, -91.20452850542926626, 4.100960146804039752 ) ) ;
#8178=CARTESIAN_POINT ( 'NONE',  ( 0.09506052544083729017, -64.50452850542926342, 2.999999999999997780 ) ) ;
#8179=CARTESIAN_POINT ( 'NONE',  ( -5.895805022753386915, -61.05452850542925347, 4.407101234057909878 ) ) ;
#8180=CARTESIAN_POINT ( 'NONE',  ( 7.360235569667877620, -79.24547149457073658, 0.09995255151716216091 ) ) ;
#8182=CARTESIAN_POINT ( 'NONE',  ( -1.529537955723776488, -83.14547149457072805, -5.030887037049945221 ) ) ;
#8183=CARTESIAN_POINT ( 'NONE',  ( 2.823794231030041235, -83.40452850542925489, -1.017458915287783316 ) ) ;
#8187=CARTESIAN_POINT ( 'NONE',  ( -1.840261337453249491, -93.30452850542926058, -2.371175808195547852 ) ) ;
#8188=CARTESIAN_POINT ( 'NONE',  ( 2.179377348189629249, -72.64547149457072805, 7.030887037049939003 ) ) ;
#8189=CARTESIAN_POINT ( 'NONE',  ( 4.742539934031843707, -96.99999999999982947, 2.318475365005189026 ) ) ;
#8190=CARTESIAN_POINT ( 'NONE',  ( -4.725907263620354293, -68.59547149457073090, -1.635492904037597617 ) ) ;
#8191=CARTESIAN_POINT ( 'NONE',  ( 0.09506052544075374588, -64.99547149457075079, -4.999999999999997335 ) ) ;
#8192=CARTESIAN_POINT ( 'NONE',  ( 1.686450176301588000, -95.70452850542928047, -2.482926158054133303 ) ) ;
#8194=CARTESIAN_POINT ( 'NONE',  ( 4.725907263620340082, -65.40452850542925489, -1.635492904037697981 ) ) ;
#8195=CARTESIAN_POINT ( 'NONE',  ( 4.191402346623081421, -97.69547149457076785, -5.607243785695398941 ) ) ;
#8196=ORIENTED_EDGE ( 'NONE', *, *, #8064, .F. ) ;
#8202=CARTESIAN_POINT ( 'NONE',  ( -2.862020680886494084, -79.20452850542925205, 4.100960146804039752 ) ) ;
#8203=CARTESIAN_POINT ( 'NONE',  ( -4.312004677470991254, -93.04547149457074795, 3.009306630940933758 ) ) ;
#8205=CARTESIAN_POINT ( 'NONE',  ( 1.529537955723688336, -59.85452850542925063, -5.030887037049978971 ) ) ;
#8206=CARTESIAN_POINT ( 'NONE',  ( 0.09506052544077554789, -70.99547149457075079, -2.999999999999997780 ) ) ;
#8207=CARTESIAN_POINT ( 'NONE',  ( 6.013306294175169597, -79.95452850542925205, 4.245374608440616093 ) ) ;
#8208=CARTESIAN_POINT ( 'NONE',  ( -4.194503406049382654, -92.44547149457073942, -3.171033256558012159 ) ) ;
#8209=CARTESIAN_POINT ( 'NONE',  ( 4.312004677471073855, -64.95452850542926626, 3.009306630940844496 ) ) ;
#8211=CARTESIAN_POINT ( 'NONE',  ( 6.628020296210641149, -74.40452850542925489, -2.253526892787612645 ) ) ;
#8212=CARTESIAN_POINT ( 'NONE',  ( -1.840261337453198864, -87.19547149457073942, 2.371175808195584267 ) ) ;
#8218=CARTESIAN_POINT ( 'NONE',  ( -4.725907263620319654, -87.90452850542926910, 1.635492904037698647 ) ) ;
#8219=CARTESIAN_POINT ( 'NONE',  ( -1.686450176301566684, -70.20452850542925205, 2.482926158054133303 ) ) ;
#8220=CARTESIAN_POINT ( 'NONE',  ( -6.013306294175155386, -57.45452850542925916, -4.245374608440613429 ) ) ;
#8221=CARTESIAN_POINT ( 'NONE',  ( -6.013306294175061240, -69.04547149457074795, 4.245374608440741326 ) ) ;
#8222=CARTESIAN_POINT ( 'NONE',  ( 4.725907263620373833, -82.09547149457074511, 1.635492904037598283 ) ) ;
#8223=CARTESIAN_POINT ( 'NONE',  ( 2.610703060766983885, -79.95452850542925205, 1.773238653441072232 ) ) ;
#8226=CARTESIAN_POINT ( 'NONE',  ( -4.784657899331192787, -57.60452850542925773, -1.454677039711773867 ) ) ;
#8227=CARTESIAN_POINT ( 'NONE',  ( 4.037591185471561595, -69.79547149457074795, 5.718994135553860936 ) ) ;
#8229=CARTESIAN_POINT ( 'NONE',  ( 4.546448683094512333, -96.99999999999961631, 2.488164940520385837 ) ) ;
#8230=CARTESIAN_POINT ( 'NONE',  ( 4.194503406049400418, -66.94547149457075363, 3.171033256558012159 ) ) ;
#8231=CARTESIAN_POINT ( 'NONE',  ( -0.09506052544073692601, -63.49547149457074369, 4.999999999999997335 ) ) ;
#8232=CARTESIAN_POINT ( 'NONE',  ( -2.493201789345250052, -94.05452850542926058, 1.934965279058294518 ) ) ;
#8234=CARTESIAN_POINT ( 'NONE',  ( -1.529537955723671683, -64.35452850542924352, 5.030887037049979860 ) ) ;
#8235=CARTESIAN_POINT ( 'NONE',  ( -4.725907263620355181, -62.59547149457074511, -1.635492904037597617 ) ) ;
#8241=DIRECTION ( 'NONE',  ( 0.9954714945707483498, 0.09506052544079827971, -1.047588144072330487E-14 ) ) ;
#8242=CARTESIAN_POINT ( 'NONE',  ( 5.257311121191341918, -74.25452850542924921, -0.09995255151729465215 ) ) ;
#8243=CARTESIAN_POINT ( 'NONE',  ( -2.862020680886579349, -89.29547149457074795, -4.100960146803977580 ) ) ;
#8244=CARTESIAN_POINT ( 'NONE',  ( -4.725907263620323207, -60.90452850542925489, 1.635492904037698647 ) ) ;
#8245=CARTESIAN_POINT ( 'NONE',  ( 3.154386672714807549, -67.24547149457075079, 0.09995255151720662534 ) ) ;
#8246=CARTESIAN_POINT ( 'NONE',  ( 2.179377348189481811, -77.85452850542925773, -7.030887037049986077 ) ) ;
#8247=CARTESIAN_POINT ( 'NONE',  ( -5.257311121191322378, -92.74547149457073658, -0.09995255151718371311 ) ) ;
#8248=CARTESIAN_POINT ( 'NONE',  ( -3.015831842038216415, -66.30452850542926058, -3.989209796945429432 ) ) ;
#8249=CARTESIAN_POINT ( 'NONE',  ( 7.360235569667878508, -80.25452850542926342, -0.09995255151731691212 ) ) ;
#8251=CARTESIAN_POINT ( 'NONE',  ( -1.840261337453199531, -84.19547149457073942, 2.371175808195584267 ) ) ;
#8256=CARTESIAN_POINT ( 'NONE',  ( -0.09506052544083846978, -90.00452850542924921, -4.999999999999997335 ) ) ;
#8257=CARTESIAN_POINT ( 'NONE',  ( -2.823794231030023028, -60.90452850542925489, 1.017458915287783316 ) ) ;
#8258=CARTESIAN_POINT ( 'NONE',  ( 4.191402346623195996, -61.80452850542926058, 5.607243785695311900 ) ) ;
#8261=CARTESIAN_POINT ( 'NONE',  ( -7.360235569667858968, -68.74547149457075079, -0.09995255151716124498 ) ) ;
#8262=CARTESIAN_POINT ( 'NONE',  ( 1.529537955723796028, -81.64547149457074227, 5.030887037049945221 ) ) ;
#8263=CARTESIAN_POINT ( 'NONE',  ( 1.686450176301586001, -80.70452850542925205, -2.482926158054133303 ) ) ;
#8267=CARTESIAN_POINT ( 'NONE',  ( -2.610703060766962569, -87.45452850542925205, -1.773238653441072232 ) ) ;
#8268=CARTESIAN_POINT ( 'NONE',  ( -6.628020296210668683, -65.59547149457073090, -2.253526892787471869 ) ) ;
#8270=CARTESIAN_POINT ( 'NONE',  ( -4.784657899331159925, -65.89547149457074227, 1.454677039711874675 ) ) ;
#8271=CARTESIAN_POINT ( 'NONE',  ( 4.191402346623081421, -94.69547149457076785, -5.607243785695398941 ) ) ;
#8273=CARTESIAN_POINT ( 'NONE',  ( -2.882544866740875289, -93.60452850542925773, -0.8366430509618996147 ) ) ;
#8276=CARTESIAN_POINT ( 'NONE',  ( -4.784657899331191011, -69.60452850542925773, -1.454677039711773867 ) ) ;
#8277=CARTESIAN_POINT ( 'NONE',  ( 0.09506052544075298261, -58.99547149457073658, -4.999999999999997335 ) ) ;
#8283=CARTESIAN_POINT ( 'NONE',  ( 4.784657899331210551, -80.10452850542925773, 1.454677039711774533 ) ) ;
#8284=CARTESIAN_POINT ( 'NONE',  ( 1.719659006605286367, -85.84547149457075932, -4.969112962950050338 ) ) ;
#8285=CARTESIAN_POINT ( 'NONE',  ( 4.069559105654484199, -96.99999999999998579, -1.141996675047574517 ) ) ;
#8286=CARTESIAN_POINT ( 'NONE',  ( 2.493201789345309116, -69.94547149457073942, 1.934965279058241006 ) ) ;
#8287=CARTESIAN_POINT ( 'NONE',  ( 6.013306294175169597, -82.95452850542925205, 4.245374608440616093 ) ) ;
#8288=CARTESIAN_POINT ( 'NONE',  ( -2.862020680886579349, -86.29547149457074795, -4.100960146803977580 ) ) ;
#8290=CARTESIAN_POINT ( 'NONE',  ( 1.529537955723688336, -59.85452850542924352, -5.030887037049978971 ) ) ;
#8291=CARTESIAN_POINT ( 'NONE',  ( -0.09506052544086139588, -75.00452850542926342, -6.999999999999997335 ) ) ;
#8292=CARTESIAN_POINT ( 'NONE',  ( 2.493201789345311781, -90.94547149457073942, 1.934965279058241006 ) ) ;
#8293=ORIENTED_EDGE ( 'NONE', *, *, #83, .F. ) ;
#8297=CARTESIAN_POINT ( 'NONE',  ( -1.719659006605370966, -87.15452850542926910, -4.969112962950015699 ) ) ;
#8298=CARTESIAN_POINT ( 'NONE',  ( -1.069819614139472019, -96.34547149457074511, 2.969112962950044121 ) ) ;
#8299=CARTESIAN_POINT ( 'NONE',  ( -4.191402346623181785, -57.30452850542924637, -5.607243785695311900 ) ) ;
#8300=CARTESIAN_POINT ( 'NONE',  ( 2.369498399071075845, -67.84547149457071669, -6.969112962950057444 ) ) ;
#8301=CARTESIAN_POINT ( 'NONE',  ( -4.725907263620352516, -86.59547149457075932, -1.635492904037597617 ) ) ;
#8302=CARTESIAN_POINT ( 'NONE',  ( 2.493201789345272257, -80.55452850542926058, -1.934965279058294518 ) ) ;
#8304=CARTESIAN_POINT ( 'NONE',  ( 2.882544866740897493, -86.10452850542924352, 0.8366430509618999478 ) ) ;
#8305=CARTESIAN_POINT ( 'NONE',  ( 7.360235569667880284, -95.25452850542926342, -0.09995255151731691212 ) ) ;
#8310=CARTESIAN_POINT ( 'NONE',  ( 3.015831842038147581, -67.69547149457073942, -3.989209796945492048 ) ) ;
#8311=CARTESIAN_POINT ( 'NONE',  ( -1.719659006605267493, -63.34547149457075221, 4.969112962950051227 ) ) ;
#8312=CARTESIAN_POINT ( 'NONE',  ( 2.610703060766986106, -91.95452850542925205, 1.773238653441072232 ) ) ;
#8316=CARTESIAN_POINT ( 'NONE',  ( -4.312004677471058756, -69.45452850542925205, -3.009306630940844052 ) ) ;
#8317=CARTESIAN_POINT ( 'NONE',  ( -0.09506052544071229293, -90.49547149457075079, 6.999999999999997335 ) ) ;
#8324=CARTESIAN_POINT ( 'NONE',  ( 3.015831842038233734, -76.80452850542926058, 3.989209796945429432 ) ) ;
#8325=CARTESIAN_POINT ( 'NONE',  ( 0.09506052544075600796, -82.99547149457075079, -4.999999999999997335 ) ) ;
#8326=CARTESIAN_POINT ( 'NONE',  ( 3.305848925379873293, -97.00000000000001421, -2.438564738088757622 ) ) ;
#8327=CARTESIAN_POINT ( 'NONE',  ( 2.882544866740876621, -70.39547149457072805, -0.8366430509619593447 ) ) ;
#8329=CARTESIAN_POINT ( 'NONE',  ( 4.191402346623198660, -82.80452850542926058, 5.607243785695311900 ) ) ;
#8330=CARTESIAN_POINT ( 'NONE',  ( -5.257311121191324155, -77.74547149457070816, -0.09995255151718371311 ) ) ;
#8331=CARTESIAN_POINT ( 'NONE',  ( -4.194503406049321370, -58.05452850542925347, 3.171033256558100533 ) ) ;
#8332=CARTESIAN_POINT ( 'NONE',  ( -3.015831842038213306, -93.30452850542926058, -3.989209796945429432 ) ) ;
#8333=CARTESIAN_POINT ( 'NONE',  ( 4.191402346623198660, -79.80452850542926058, 5.607243785695311900 ) ) ;
#8334=CARTESIAN_POINT ( 'NONE',  ( -2.882544866740857081, -83.89547149457074227, 0.8366430509619596778 ) ) ;
#8337=CARTESIAN_POINT ( 'NONE',  ( -3.154386672714788453, -84.75452850542926342, 0.09995255151727280851 ) ) ;
ENDSEC;
END-ISO-10303-21;
